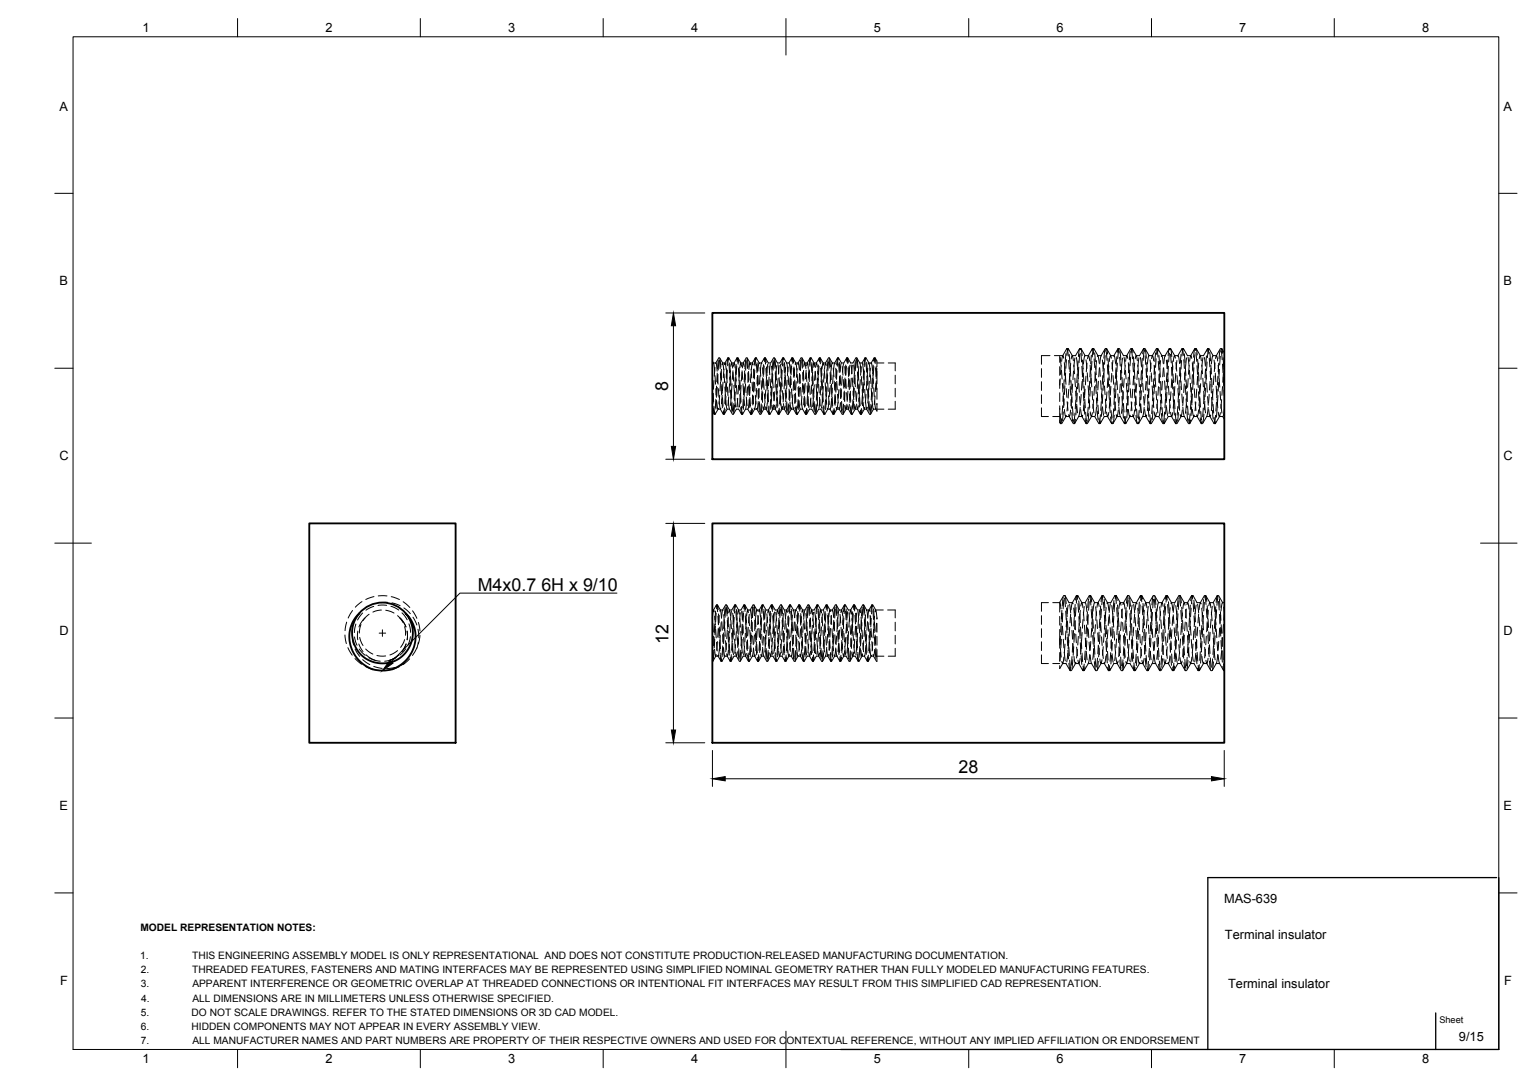
ISO-10303-21;
HEADER;
/* Generated by software containing ST-Developer
 * from STEP Tools, Inc. (www.steptools.com) 
 */

FILE_DESCRIPTION(
/* description */ ('Independent maintained push-to-latch/pull-to-reset mushroom-operator 
CAD. Two opposed spring-loaded ball detents in turned circular seats b
ias both travel stops; direct normally-closed bridge opens6mm when pre
ssed. Rounded palm/pull rim, captured head screw, removable detent clo
sures, native Coil spring families, insulated shared terminals and ord
inary machining features. Manual geometric states and ideal same-mater
ial spring-energy direction only; no electrical/safety certification, 
force/contact dynamics, wear, load or life rating. Requested blue/gray
 visual palette, not safety identification. External wiring/anchors an
d application engineering omitted.'),
/* implementation_level */ '2;1');

FILE_NAME(
/* name */ 'Terminal insulator.step',
/* time_stamp */ '2026-11-08T17:54:26-08:00',
/* author */ (''),
/* organization */ (''),
/* preprocessor_version */ 'ST-DEVELOPER v20.2',
/* originating_system */ 'Autodesk Translation Framework v15.17.0.0',
/* authorisation */ '');

FILE_SCHEMA (('AUTOMOTIVE_DESIGN { 1 0 10303 214 3 1 1 }'));
ENDSEC;

DATA;
#10=MECHANICAL_DESIGN_GEOMETRIC_PRESENTATION_REPRESENTATION('',(#197),#43980);
#163=SHAPE_REPRESENTATION_RELATIONSHIP('SRR','None',#44063,#180);
#180=ADVANCED_BREP_SHAPE_REPRESENTATION('',(#214),#43970);
#197=STYLED_ITEM('',(#44156),#214);
#214=MANIFOLD_SOLID_BREP('Body1',#11238);
#243=B_SPLINE_SURFACE_WITH_KNOTS('',3,3,((#32192,#32193,#32194,#32195,#32196,
#32197,#32198,#32199,#32200,#32201,#32202,#32203,#32204,#32205,#32206,#32207,
#32208,#32209,#32210,#32211,#32212,#32213,#32214,#32215,#32216,#32217,#32218,
#32219,#32220,#32221,#32222,#32223,#32224,#32225,#32226,#32227,#32228,#32229,
#32230,#32231,#32232,#32233,#32234,#32235,#32236,#32237,#32238,#32239,#32240,
#32241,#32242,#32243,#32244,#32245,#32246,#32247,#32248,#32249,#32250,#32251,
#32252,#32253,#32254,#32255,#32256,#32257,#32258,#32259,#32260,#32261,#32262,
#32263,#32264,#32265,#32266,#32267,#32268,#32269,#32270,#32271,#32272,#32273,
#32274,#32275,#32276,#32277,#32278,#32279,#32280,#32281,#32282,#32283,#32284,
#32285,#32286,#32287,#32288,#32289,#32290,#32291,#32292,#32293,#32294,#32295,
#32296,#32297,#32298,#32299,#32300,#32301,#32302,#32303,#32304,#32305,#32306,
#32307,#32308,#32309,#32310),(#32311,#32312,#32313,#32314,#32315,#32316,
#32317,#32318,#32319,#32320,#32321,#32322,#32323,#32324,#32325,#32326,#32327,
#32328,#32329,#32330,#32331,#32332,#32333,#32334,#32335,#32336,#32337,#32338,
#32339,#32340,#32341,#32342,#32343,#32344,#32345,#32346,#32347,#32348,#32349,
#32350,#32351,#32352,#32353,#32354,#32355,#32356,#32357,#32358,#32359,#32360,
#32361,#32362,#32363,#32364,#32365,#32366,#32367,#32368,#32369,#32370,#32371,
#32372,#32373,#32374,#32375,#32376,#32377,#32378,#32379,#32380,#32381,#32382,
#32383,#32384,#32385,#32386,#32387,#32388,#32389,#32390,#32391,#32392,#32393,
#32394,#32395,#32396,#32397,#32398,#32399,#32400,#32401,#32402,#32403,#32404,
#32405,#32406,#32407,#32408,#32409,#32410,#32411,#32412,#32413,#32414,#32415,
#32416,#32417,#32418,#32419,#32420,#32421,#32422,#32423,#32424,#32425,#32426,
#32427,#32428,#32429),(#32430,#32431,#32432,#32433,#32434,#32435,#32436,
#32437,#32438,#32439,#32440,#32441,#32442,#32443,#32444,#32445,#32446,#32447,
#32448,#32449,#32450,#32451,#32452,#32453,#32454,#32455,#32456,#32457,#32458,
#32459,#32460,#32461,#32462,#32463,#32464,#32465,#32466,#32467,#32468,#32469,
#32470,#32471,#32472,#32473,#32474,#32475,#32476,#32477,#32478,#32479,#32480,
#32481,#32482,#32483,#32484,#32485,#32486,#32487,#32488,#32489,#32490,#32491,
#32492,#32493,#32494,#32495,#32496,#32497,#32498,#32499,#32500,#32501,#32502,
#32503,#32504,#32505,#32506,#32507,#32508,#32509,#32510,#32511,#32512,#32513,
#32514,#32515,#32516,#32517,#32518,#32519,#32520,#32521,#32522,#32523,#32524,
#32525,#32526,#32527,#32528,#32529,#32530,#32531,#32532,#32533,#32534,#32535,
#32536,#32537,#32538,#32539,#32540,#32541,#32542,#32543,#32544,#32545,#32546,
#32547,#32548),(#32549,#32550,#32551,#32552,#32553,#32554,#32555,#32556,
#32557,#32558,#32559,#32560,#32561,#32562,#32563,#32564,#32565,#32566,#32567,
#32568,#32569,#32570,#32571,#32572,#32573,#32574,#32575,#32576,#32577,#32578,
#32579,#32580,#32581,#32582,#32583,#32584,#32585,#32586,#32587,#32588,#32589,
#32590,#32591,#32592,#32593,#32594,#32595,#32596,#32597,#32598,#32599,#32600,
#32601,#32602,#32603,#32604,#32605,#32606,#32607,#32608,#32609,#32610,#32611,
#32612,#32613,#32614,#32615,#32616,#32617,#32618,#32619,#32620,#32621,#32622,
#32623,#32624,#32625,#32626,#32627,#32628,#32629,#32630,#32631,#32632,#32633,
#32634,#32635,#32636,#32637,#32638,#32639,#32640,#32641,#32642,#32643,#32644,
#32645,#32646,#32647,#32648,#32649,#32650,#32651,#32652,#32653,#32654,#32655,
#32656,#32657,#32658,#32659,#32660,#32661,#32662,#32663,#32664,#32665,#32666,
#32667)),.UNSPECIFIED.,.F.,.F.,.F.,(4,4),(4,1,1,1,1,1,1,1,1,1,1,1,1,1,1,
1,1,1,1,1,1,1,1,1,1,1,1,1,1,1,1,1,1,1,1,1,1,1,1,1,1,1,1,1,1,1,1,1,1,1,1,
1,1,1,1,1,1,1,1,1,1,1,1,1,1,1,1,1,1,1,1,1,1,1,1,1,1,1,1,1,1,1,1,1,1,1,1,
1,1,1,1,1,1,1,1,1,1,1,1,1,1,1,1,1,1,1,1,1,1,1,1,1,1,1,1,1,4),(0.,0.0321584099938621),
(11.8553612635792,12.8477570223809,13.8401527811825,14.8325485399841,15.8249442987858,
16.8173400575874,17.809735816389,18.8021315751907,19.7945273339923,20.7869230927939,
21.7793188515956,22.7717146103972,23.7641103691988,24.7565061280005,25.7489018868021,
26.7412976456037,27.7336934044054,28.726089163207,29.7184849220086,30.7108806808103,
31.7032764396119,32.6956721984135,33.6880679572152,34.6804637160168,35.6728594748184,
36.6652552336201,37.6576509924217,38.6500467512233,39.642442510025,40.6348382688266,
41.6272340276282,42.6196297864299,43.6120255452315,44.6044213040331,45.5968170628348,
46.5892128216364,47.581608580438,48.5740043392397,49.5664000980413,50.5587958568429,
51.5511916156446,52.5435873744462,53.5359831332478,54.5283788920495,55.5207746508511,
56.5131704096527,57.5055661684544,58.497961927256,59.4903576860576,60.4827534448593,
61.4751492036609,62.4675449624625,63.4599407212642,64.4523364800658,65.4447322388674,
66.4371279976691,67.4295237564707,68.4219195152723,69.4143152740739,70.4067110328756,
71.3991067916772,72.3915025504788,73.3838983092805,74.3762940680821,75.3686898268838,
76.3610855856854,77.353481344487,78.3458771032886,79.3382728620903,80.3306686208919,
81.3230643796935,82.3154601384952,83.3078558972968,84.3002516560985,85.2926474149001,
86.2850431737017,87.2774389325033,88.269834691305,89.2622304501066,90.2546262089082,
91.2470219677099,92.2394177265115,93.2318134853131,94.2242092441148,95.2166050029164,
96.209000761718,97.2013965205197,98.1937922793213,99.1861880381229,100.178583796925,
101.170979555726,102.163375314528,103.155771073329,104.148166832131,105.140562590933,
106.132958349734,107.125354108536,108.117749867338,109.110145626139,110.102541384941,
111.094937143743,112.087332902544,113.079728661346,114.072124420147,115.064520178949,
116.056915937751,117.049311696552,118.041707455354,119.034103214156,120.026498972957,
121.018894731759,122.01129049056,123.003686249362,123.996082008164,124.988477766965,
125.980873525767,126.973269284569),.UNSPECIFIED.);
#244=B_SPLINE_SURFACE_WITH_KNOTS('',3,3,((#32742,#32743,#32744,#32745,#32746,
#32747,#32748,#32749,#32750,#32751,#32752,#32753,#32754,#32755,#32756,#32757,
#32758,#32759,#32760,#32761,#32762,#32763,#32764,#32765,#32766,#32767,#32768,
#32769,#32770,#32771,#32772,#32773,#32774,#32775,#32776,#32777,#32778,#32779,
#32780,#32781,#32782,#32783,#32784,#32785,#32786,#32787,#32788,#32789,#32790,
#32791,#32792,#32793,#32794,#32795,#32796,#32797,#32798,#32799,#32800,#32801,
#32802,#32803,#32804,#32805,#32806,#32807,#32808,#32809,#32810,#32811,#32812,
#32813,#32814,#32815,#32816,#32817,#32818,#32819,#32820,#32821,#32822,#32823,
#32824,#32825,#32826,#32827,#32828,#32829,#32830,#32831,#32832,#32833,#32834,
#32835,#32836,#32837,#32838,#32839,#32840,#32841,#32842,#32843,#32844,#32845,
#32846,#32847,#32848,#32849,#32850,#32851,#32852,#32853,#32854,#32855,#32856,
#32857,#32858,#32859,#32860),(#32861,#32862,#32863,#32864,#32865,#32866,
#32867,#32868,#32869,#32870,#32871,#32872,#32873,#32874,#32875,#32876,#32877,
#32878,#32879,#32880,#32881,#32882,#32883,#32884,#32885,#32886,#32887,#32888,
#32889,#32890,#32891,#32892,#32893,#32894,#32895,#32896,#32897,#32898,#32899,
#32900,#32901,#32902,#32903,#32904,#32905,#32906,#32907,#32908,#32909,#32910,
#32911,#32912,#32913,#32914,#32915,#32916,#32917,#32918,#32919,#32920,#32921,
#32922,#32923,#32924,#32925,#32926,#32927,#32928,#32929,#32930,#32931,#32932,
#32933,#32934,#32935,#32936,#32937,#32938,#32939,#32940,#32941,#32942,#32943,
#32944,#32945,#32946,#32947,#32948,#32949,#32950,#32951,#32952,#32953,#32954,
#32955,#32956,#32957,#32958,#32959,#32960,#32961,#32962,#32963,#32964,#32965,
#32966,#32967,#32968,#32969,#32970,#32971,#32972,#32973,#32974,#32975,#32976,
#32977,#32978,#32979),(#32980,#32981,#32982,#32983,#32984,#32985,#32986,
#32987,#32988,#32989,#32990,#32991,#32992,#32993,#32994,#32995,#32996,#32997,
#32998,#32999,#33000,#33001,#33002,#33003,#33004,#33005,#33006,#33007,#33008,
#33009,#33010,#33011,#33012,#33013,#33014,#33015,#33016,#33017,#33018,#33019,
#33020,#33021,#33022,#33023,#33024,#33025,#33026,#33027,#33028,#33029,#33030,
#33031,#33032,#33033,#33034,#33035,#33036,#33037,#33038,#33039,#33040,#33041,
#33042,#33043,#33044,#33045,#33046,#33047,#33048,#33049,#33050,#33051,#33052,
#33053,#33054,#33055,#33056,#33057,#33058,#33059,#33060,#33061,#33062,#33063,
#33064,#33065,#33066,#33067,#33068,#33069,#33070,#33071,#33072,#33073,#33074,
#33075,#33076,#33077,#33078,#33079,#33080,#33081,#33082,#33083,#33084,#33085,
#33086,#33087,#33088,#33089,#33090,#33091,#33092,#33093,#33094,#33095,#33096,
#33097,#33098),(#33099,#33100,#33101,#33102,#33103,#33104,#33105,#33106,
#33107,#33108,#33109,#33110,#33111,#33112,#33113,#33114,#33115,#33116,#33117,
#33118,#33119,#33120,#33121,#33122,#33123,#33124,#33125,#33126,#33127,#33128,
#33129,#33130,#33131,#33132,#33133,#33134,#33135,#33136,#33137,#33138,#33139,
#33140,#33141,#33142,#33143,#33144,#33145,#33146,#33147,#33148,#33149,#33150,
#33151,#33152,#33153,#33154,#33155,#33156,#33157,#33158,#33159,#33160,#33161,
#33162,#33163,#33164,#33165,#33166,#33167,#33168,#33169,#33170,#33171,#33172,
#33173,#33174,#33175,#33176,#33177,#33178,#33179,#33180,#33181,#33182,#33183,
#33184,#33185,#33186,#33187,#33188,#33189,#33190,#33191,#33192,#33193,#33194,
#33195,#33196,#33197,#33198,#33199,#33200,#33201,#33202,#33203,#33204,#33205,
#33206,#33207,#33208,#33209,#33210,#33211,#33212,#33213,#33214,#33215,#33216,
#33217)),.UNSPECIFIED.,.F.,.F.,.F.,(4,4),(4,1,1,1,1,1,1,1,1,1,1,1,1,1,1,
1,1,1,1,1,1,1,1,1,1,1,1,1,1,1,1,1,1,1,1,1,1,1,1,1,1,1,1,1,1,1,1,1,1,1,1,
1,1,1,1,1,1,1,1,1,1,1,1,1,1,1,1,1,1,1,1,1,1,1,1,1,1,1,1,1,1,1,1,1,1,1,1,
1,1,1,1,1,1,1,1,1,1,1,1,1,1,1,1,1,1,1,1,1,1,1,1,1,1,1,1,1,4),(0.,0.0321584099938621),
(14.3984001269718,15.3907958857734,16.383191644575,17.3755874033767,18.3679831621783,
19.3603789209799,20.3527746797816,21.3451704385832,22.3375661973848,23.3299619561865,
24.3223577149881,25.3147534737897,26.3071492325914,27.299544991393,28.2919407501946,
29.2843365089963,30.2767322677979,31.2691280265995,32.2615237854012,33.2539195442028,
34.2463153030044,35.2387110618061,36.2311068206077,37.2235025794093,38.215898338211,
39.2082940970126,40.2006898558142,41.1930856146159,42.1854813734175,43.1778771322191,
44.1702728910208,45.1626686498224,46.155064408624,47.1474601674257,48.1398559262273,
49.1322516850289,50.1246474438306,51.1170432026322,52.1094389614338,53.1018347202355,
54.0942304790371,55.0866262378387,56.0790219966403,57.071417755442,58.0638135142436,
59.0562092730452,60.0486050318469,61.0410007906485,62.0333965494501,63.0257923082518,
64.0181880670534,65.010583825855,66.0029795846567,66.9953753434583,67.9877711022599,
68.9801668610616,69.9725626198632,70.9649583786648,71.9573541374665,72.9497498962681,
73.9421456550697,74.9345414138714,75.926937172673,76.9193329314746,77.9117286902763,
78.9041244490779,79.8965202078795,80.8889159666812,81.8813117254828,82.8737074842844,
83.8661032430861,84.8584990018877,85.8508947606893,86.8432905194909,87.8356862782926,
88.8280820370942,89.8204777958959,90.8128735546975,91.8052693134991,92.7976650723007,
93.7900608311024,94.782456589904,95.7748523487057,96.7672481075073,97.7596438663089,
98.7520396251105,99.7444353839122,100.736831142714,101.729226901515,102.721622660317,
103.714018419119,104.70641417792,105.698809936722,106.691205695524,107.683601454325,
108.675997213127,109.668392971929,110.66078873073,111.653184489532,112.645580248333,
113.637976007135,114.630371765937,115.622767524738,116.61516328354,117.607559042342,
118.599954801143,119.592350559945,120.584746318746,121.577142077548,122.56953783635,
123.561933595151,124.554329353953,125.546725112755,126.539120871556,127.531516630358,
128.52391238916,129.516308147961),.UNSPECIFIED.);
#245=B_SPLINE_SURFACE_WITH_KNOTS('',3,3,((#33424,#33425,#33426,#33427,#33428,
#33429,#33430,#33431,#33432,#33433,#33434,#33435,#33436,#33437,#33438,#33439,
#33440,#33441,#33442,#33443,#33444,#33445,#33446,#33447,#33448,#33449,#33450,
#33451,#33452,#33453,#33454,#33455,#33456,#33457,#33458,#33459,#33460,#33461,
#33462,#33463,#33464,#33465,#33466,#33467,#33468,#33469,#33470,#33471,#33472,
#33473,#33474,#33475,#33476,#33477,#33478,#33479,#33480,#33481,#33482,#33483,
#33484,#33485,#33486,#33487,#33488,#33489,#33490,#33491,#33492,#33493,#33494,
#33495,#33496,#33497,#33498,#33499,#33500,#33501,#33502,#33503,#33504,#33505,
#33506,#33507,#33508,#33509),(#33510,#33511,#33512,#33513,#33514,#33515,
#33516,#33517,#33518,#33519,#33520,#33521,#33522,#33523,#33524,#33525,#33526,
#33527,#33528,#33529,#33530,#33531,#33532,#33533,#33534,#33535,#33536,#33537,
#33538,#33539,#33540,#33541,#33542,#33543,#33544,#33545,#33546,#33547,#33548,
#33549,#33550,#33551,#33552,#33553,#33554,#33555,#33556,#33557,#33558,#33559,
#33560,#33561,#33562,#33563,#33564,#33565,#33566,#33567,#33568,#33569,#33570,
#33571,#33572,#33573,#33574,#33575,#33576,#33577,#33578,#33579,#33580,#33581,
#33582,#33583,#33584,#33585,#33586,#33587,#33588,#33589,#33590,#33591,#33592,
#33593,#33594,#33595),(#33596,#33597,#33598,#33599,#33600,#33601,#33602,
#33603,#33604,#33605,#33606,#33607,#33608,#33609,#33610,#33611,#33612,#33613,
#33614,#33615,#33616,#33617,#33618,#33619,#33620,#33621,#33622,#33623,#33624,
#33625,#33626,#33627,#33628,#33629,#33630,#33631,#33632,#33633,#33634,#33635,
#33636,#33637,#33638,#33639,#33640,#33641,#33642,#33643,#33644,#33645,#33646,
#33647,#33648,#33649,#33650,#33651,#33652,#33653,#33654,#33655,#33656,#33657,
#33658,#33659,#33660,#33661,#33662,#33663,#33664,#33665,#33666,#33667,#33668,
#33669,#33670,#33671,#33672,#33673,#33674,#33675,#33676,#33677,#33678,#33679,
#33680,#33681),(#33682,#33683,#33684,#33685,#33686,#33687,#33688,#33689,
#33690,#33691,#33692,#33693,#33694,#33695,#33696,#33697,#33698,#33699,#33700,
#33701,#33702,#33703,#33704,#33705,#33706,#33707,#33708,#33709,#33710,#33711,
#33712,#33713,#33714,#33715,#33716,#33717,#33718,#33719,#33720,#33721,#33722,
#33723,#33724,#33725,#33726,#33727,#33728,#33729,#33730,#33731,#33732,#33733,
#33734,#33735,#33736,#33737,#33738,#33739,#33740,#33741,#33742,#33743,#33744,
#33745,#33746,#33747,#33748,#33749,#33750,#33751,#33752,#33753,#33754,#33755,
#33756,#33757,#33758,#33759,#33760,#33761,#33762,#33763,#33764,#33765,#33766,
#33767)),.UNSPECIFIED.,.F.,.F.,.F.,(4,4),(4,1,1,1,1,1,1,1,1,1,1,1,1,1,1,
1,1,1,1,1,1,1,1,1,1,1,1,1,1,1,1,1,1,1,1,1,1,1,1,1,1,1,1,1,1,1,1,1,1,1,1,
1,1,1,1,1,1,1,1,1,1,1,1,1,1,1,1,1,1,1,1,1,1,1,1,1,1,1,1,1,1,1,1,4),(0.,
0.0448889834294934),(11.8615800042567,12.8591513772396,13.8567227502225,
14.8542941232054,15.8518654961884,16.8494368691713,17.8470082421542,18.8445796151372,
19.8421509881201,20.839722361103,21.837293734086,22.8348651070689,23.8324364800518,
24.8300078530348,25.8275792260177,26.8251505990006,27.8227219719836,28.8202933449665,
29.8178647179494,30.8154360909324,31.8130074639153,32.8105788368982,33.8081502098812,
34.8057215828641,35.803292955847,36.80086432883,37.7984357018129,38.7960070747958,
39.7935784477788,40.7911498207617,41.7887211937446,42.7862925667276,43.7838639397105,
44.7814353126934,45.7790066856764,46.7765780586593,47.7741494316422,48.7717208046252,
49.7692921776081,50.766863550591,51.764434923574,52.7620062965569,53.7595776695398,
54.7571490425228,55.7547204155057,56.7522917884886,57.7498631614716,58.7474345344545,
59.7450059074374,60.7425772804204,61.7401486534033,62.7377200263862,63.7352913993692,
64.7328627723521,65.730434145335,66.728005518318,67.7255768913009,68.7231482642838,
69.7207196372668,70.7182910102497,71.7158623832326,72.7134337562156,73.7110051291985,
74.7085765021814,75.7061478751643,76.7037192481473,77.7012906211302,78.6988619941132,
79.6964333670961,80.694004740079,81.691576113062,82.6891474860449,83.6867188590278,
84.6842902320108,85.6818616049937,86.6794329779766,87.6770043509595,88.6745757239425,
89.6721470969254,90.6697184699083,91.6672898428913,92.6648612158742,93.6624325888571,
94.6600039618401),.UNSPECIFIED.);
#246=B_SPLINE_SURFACE_WITH_KNOTS('',3,3,((#33845,#33846,#33847,#33848,#33849,
#33850,#33851,#33852,#33853,#33854,#33855,#33856,#33857,#33858,#33859,#33860,
#33861,#33862,#33863,#33864,#33865,#33866,#33867,#33868,#33869,#33870,#33871,
#33872,#33873,#33874,#33875,#33876,#33877,#33878,#33879,#33880,#33881,#33882,
#33883,#33884,#33885,#33886,#33887,#33888,#33889,#33890,#33891,#33892,#33893,
#33894,#33895,#33896,#33897,#33898,#33899,#33900,#33901,#33902,#33903,#33904,
#33905,#33906,#33907,#33908,#33909,#33910,#33911,#33912,#33913,#33914,#33915,
#33916,#33917,#33918,#33919,#33920,#33921,#33922,#33923,#33924,#33925,#33926,
#33927,#33928,#33929,#33930),(#33931,#33932,#33933,#33934,#33935,#33936,
#33937,#33938,#33939,#33940,#33941,#33942,#33943,#33944,#33945,#33946,#33947,
#33948,#33949,#33950,#33951,#33952,#33953,#33954,#33955,#33956,#33957,#33958,
#33959,#33960,#33961,#33962,#33963,#33964,#33965,#33966,#33967,#33968,#33969,
#33970,#33971,#33972,#33973,#33974,#33975,#33976,#33977,#33978,#33979,#33980,
#33981,#33982,#33983,#33984,#33985,#33986,#33987,#33988,#33989,#33990,#33991,
#33992,#33993,#33994,#33995,#33996,#33997,#33998,#33999,#34000,#34001,#34002,
#34003,#34004,#34005,#34006,#34007,#34008,#34009,#34010,#34011,#34012,#34013,
#34014,#34015,#34016),(#34017,#34018,#34019,#34020,#34021,#34022,#34023,
#34024,#34025,#34026,#34027,#34028,#34029,#34030,#34031,#34032,#34033,#34034,
#34035,#34036,#34037,#34038,#34039,#34040,#34041,#34042,#34043,#34044,#34045,
#34046,#34047,#34048,#34049,#34050,#34051,#34052,#34053,#34054,#34055,#34056,
#34057,#34058,#34059,#34060,#34061,#34062,#34063,#34064,#34065,#34066,#34067,
#34068,#34069,#34070,#34071,#34072,#34073,#34074,#34075,#34076,#34077,#34078,
#34079,#34080,#34081,#34082,#34083,#34084,#34085,#34086,#34087,#34088,#34089,
#34090,#34091,#34092,#34093,#34094,#34095,#34096,#34097,#34098,#34099,#34100,
#34101,#34102),(#34103,#34104,#34105,#34106,#34107,#34108,#34109,#34110,
#34111,#34112,#34113,#34114,#34115,#34116,#34117,#34118,#34119,#34120,#34121,
#34122,#34123,#34124,#34125,#34126,#34127,#34128,#34129,#34130,#34131,#34132,
#34133,#34134,#34135,#34136,#34137,#34138,#34139,#34140,#34141,#34142,#34143,
#34144,#34145,#34146,#34147,#34148,#34149,#34150,#34151,#34152,#34153,#34154,
#34155,#34156,#34157,#34158,#34159,#34160,#34161,#34162,#34163,#34164,#34165,
#34166,#34167,#34168,#34169,#34170,#34171,#34172,#34173,#34174,#34175,#34176,
#34177,#34178,#34179,#34180,#34181,#34182,#34183,#34184,#34185,#34186,#34187,
#34188)),.UNSPECIFIED.,.F.,.F.,.F.,(4,4),(4,1,1,1,1,1,1,1,1,1,1,1,1,1,1,
1,1,1,1,1,1,1,1,1,1,1,1,1,1,1,1,1,1,1,1,1,1,1,1,1,1,1,1,1,1,1,1,1,1,1,1,
1,1,1,1,1,1,1,1,1,1,1,1,1,1,1,1,1,1,1,1,1,1,1,1,1,1,1,1,1,1,1,1,4),(0.,
0.0448889834294934),(14.3981410127769,15.3957123857598,16.3932837587428,
17.3908551317257,18.3884265047086,19.3859978776916,20.3835692506745,21.3811406236574,
22.3787119966404,23.3762833696233,24.3738547426062,25.3714261155892,26.3689974885721,
27.366568861555,28.364140234538,29.3617116075209,30.3592829805038,31.3568543534868,
32.3544257264697,33.3519970994526,34.3495684724355,35.3471398454185,36.3447112184014,
37.3422825913843,38.3398539643673,39.3374253373502,40.3349967103331,41.3325680833161,
42.330139456299,43.3277108292819,44.3252822022649,45.3228535752478,46.3204249482307,
47.3179963212137,48.3155676941966,49.3131390671795,50.3107104401625,51.3082818131454,
52.3058531861283,53.3034245591113,54.3009959320942,55.2985673050771,56.2961386780601,
57.293710051043,58.2912814240259,59.2888527970089,60.2864241699918,61.2839955429747,
62.2815669159577,63.2791382889406,64.2767096619235,65.2742810349065,66.2718524078894,
67.2694237808723,68.2669951538553,69.2645665268382,70.2621378998211,71.2597092728041,
72.257280645787,73.2548520187699,74.2524233917529,75.2499947647358,76.2475661377187,
77.2451375107017,78.2427088836846,79.2402802566675,80.2378516296505,81.2354230026334,
82.2329943756163,83.2305657485993,84.2281371215822,85.2257084945651,86.2232798675481,
87.220851240531,88.2184226135139,89.2159939864969,90.2135653594798,91.2111367324627,
92.2087081054457,93.2062794784286,94.2038508514115,95.2014222243944,96.1989935973774,
97.1965649703603),.UNSPECIFIED.);
#315=FACE_BOUND('',#1577,.T.);
#316=FACE_BOUND('',#1579,.T.);
#413=PLANE('',#11969);
#414=PLANE('',#11972);
#415=PLANE('',#11973);
#416=PLANE('',#11976);
#417=PLANE('',#11977);
#418=PLANE('',#11978);
#419=PLANE('',#11979);
#420=PLANE('',#11980);
#421=PLANE('',#11981);
#422=PLANE('',#11982);
#820=FACE_OUTER_BOUND('',#1499,.T.);
#821=FACE_OUTER_BOUND('',#1500,.T.);
#822=FACE_OUTER_BOUND('',#1501,.T.);
#823=FACE_OUTER_BOUND('',#1502,.T.);
#824=FACE_OUTER_BOUND('',#1503,.T.);
#825=FACE_OUTER_BOUND('',#1504,.T.);
#826=FACE_OUTER_BOUND('',#1505,.T.);
#827=FACE_OUTER_BOUND('',#1506,.T.);
#828=FACE_OUTER_BOUND('',#1507,.T.);
#829=FACE_OUTER_BOUND('',#1508,.T.);
#830=FACE_OUTER_BOUND('',#1509,.T.);
#831=FACE_OUTER_BOUND('',#1510,.T.);
#832=FACE_OUTER_BOUND('',#1511,.T.);
#833=FACE_OUTER_BOUND('',#1512,.T.);
#834=FACE_OUTER_BOUND('',#1513,.T.);
#835=FACE_OUTER_BOUND('',#1514,.T.);
#836=FACE_OUTER_BOUND('',#1515,.T.);
#837=FACE_OUTER_BOUND('',#1516,.T.);
#838=FACE_OUTER_BOUND('',#1517,.T.);
#839=FACE_OUTER_BOUND('',#1518,.T.);
#840=FACE_OUTER_BOUND('',#1519,.T.);
#841=FACE_OUTER_BOUND('',#1520,.T.);
#842=FACE_OUTER_BOUND('',#1521,.T.);
#843=FACE_OUTER_BOUND('',#1522,.T.);
#844=FACE_OUTER_BOUND('',#1523,.T.);
#845=FACE_OUTER_BOUND('',#1524,.T.);
#846=FACE_OUTER_BOUND('',#1525,.T.);
#847=FACE_OUTER_BOUND('',#1526,.T.);
#848=FACE_OUTER_BOUND('',#1527,.T.);
#849=FACE_OUTER_BOUND('',#1528,.T.);
#850=FACE_OUTER_BOUND('',#1529,.T.);
#851=FACE_OUTER_BOUND('',#1530,.T.);
#852=FACE_OUTER_BOUND('',#1531,.T.);
#853=FACE_OUTER_BOUND('',#1532,.T.);
#854=FACE_OUTER_BOUND('',#1533,.T.);
#855=FACE_OUTER_BOUND('',#1534,.T.);
#856=FACE_OUTER_BOUND('',#1535,.T.);
#857=FACE_OUTER_BOUND('',#1536,.T.);
#858=FACE_OUTER_BOUND('',#1537,.T.);
#859=FACE_OUTER_BOUND('',#1538,.T.);
#860=FACE_OUTER_BOUND('',#1539,.T.);
#861=FACE_OUTER_BOUND('',#1540,.T.);
#862=FACE_OUTER_BOUND('',#1541,.T.);
#863=FACE_OUTER_BOUND('',#1542,.T.);
#864=FACE_OUTER_BOUND('',#1543,.T.);
#865=FACE_OUTER_BOUND('',#1544,.T.);
#866=FACE_OUTER_BOUND('',#1545,.T.);
#867=FACE_OUTER_BOUND('',#1546,.T.);
#868=FACE_OUTER_BOUND('',#1547,.T.);
#869=FACE_OUTER_BOUND('',#1548,.T.);
#870=FACE_OUTER_BOUND('',#1549,.T.);
#871=FACE_OUTER_BOUND('',#1550,.T.);
#872=FACE_OUTER_BOUND('',#1551,.T.);
#873=FACE_OUTER_BOUND('',#1552,.T.);
#874=FACE_OUTER_BOUND('',#1553,.T.);
#875=FACE_OUTER_BOUND('',#1554,.T.);
#876=FACE_OUTER_BOUND('',#1555,.T.);
#877=FACE_OUTER_BOUND('',#1556,.T.);
#878=FACE_OUTER_BOUND('',#1557,.T.);
#879=FACE_OUTER_BOUND('',#1558,.T.);
#880=FACE_OUTER_BOUND('',#1559,.T.);
#881=FACE_OUTER_BOUND('',#1560,.T.);
#882=FACE_OUTER_BOUND('',#1561,.T.);
#883=FACE_OUTER_BOUND('',#1562,.T.);
#884=FACE_OUTER_BOUND('',#1563,.T.);
#885=FACE_OUTER_BOUND('',#1564,.T.);
#886=FACE_OUTER_BOUND('',#1565,.T.);
#887=FACE_OUTER_BOUND('',#1566,.T.);
#888=FACE_OUTER_BOUND('',#1567,.T.);
#889=FACE_OUTER_BOUND('',#1568,.T.);
#890=FACE_OUTER_BOUND('',#1569,.T.);
#891=FACE_OUTER_BOUND('',#1570,.T.);
#892=FACE_OUTER_BOUND('',#1571,.T.);
#893=FACE_OUTER_BOUND('',#1572,.T.);
#894=FACE_OUTER_BOUND('',#1573,.T.);
#895=FACE_OUTER_BOUND('',#1574,.T.);
#896=FACE_OUTER_BOUND('',#1575,.T.);
#897=FACE_OUTER_BOUND('',#1576,.T.);
#898=FACE_OUTER_BOUND('',#1578,.T.);
#1499=EDGE_LOOP('',(#8651,#8652,#8653,#8654,#8655,#8656,#8657,#8658));
#1500=EDGE_LOOP('',(#8659,#8660,#8661,#8662));
#1501=EDGE_LOOP('',(#8663,#8664,#8665,#8666));
#1502=EDGE_LOOP('',(#8667,#8668,#8669,#8670));
#1503=EDGE_LOOP('',(#8671,#8672,#8673,#8674));
#1504=EDGE_LOOP('',(#8675,#8676,#8677,#8678));
#1505=EDGE_LOOP('',(#8679,#8680,#8681,#8682));
#1506=EDGE_LOOP('',(#8683,#8684,#8685,#8686));
#1507=EDGE_LOOP('',(#8687,#8688,#8689,#8690));
#1508=EDGE_LOOP('',(#8691,#8692,#8693,#8694));
#1509=EDGE_LOOP('',(#8695,#8696,#8697,#8698));
#1510=EDGE_LOOP('',(#8699,#8700,#8701,#8702));
#1511=EDGE_LOOP('',(#8703,#8704,#8705,#8706));
#1512=EDGE_LOOP('',(#8707,#8708,#8709,#8710));
#1513=EDGE_LOOP('',(#8711,#8712,#8713,#8714));
#1514=EDGE_LOOP('',(#8715,#8716,#8717,#8718));
#1515=EDGE_LOOP('',(#8719,#8720,#8721,#8722));
#1516=EDGE_LOOP('',(#8723,#8724,#8725,#8726));
#1517=EDGE_LOOP('',(#8727,#8728,#8729,#8730));
#1518=EDGE_LOOP('',(#8731,#8732,#8733,#8734));
#1519=EDGE_LOOP('',(#8735,#8736,#8737,#8738));
#1520=EDGE_LOOP('',(#8739,#8740,#8741,#8742));
#1521=EDGE_LOOP('',(#8743,#8744,#8745,#8746));
#1522=EDGE_LOOP('',(#8747,#8748,#8749,#8750));
#1523=EDGE_LOOP('',(#8751,#8752,#8753,#8754));
#1524=EDGE_LOOP('',(#8755,#8756,#8757,#8758,#8759,#8760,#8761,#8762));
#1525=EDGE_LOOP('',(#8763,#8764,#8765,#8766));
#1526=EDGE_LOOP('',(#8767,#8768,#8769,#8770));
#1527=EDGE_LOOP('',(#8771,#8772,#8773,#8774));
#1528=EDGE_LOOP('',(#8775,#8776,#8777,#8778));
#1529=EDGE_LOOP('',(#8779,#8780,#8781,#8782));
#1530=EDGE_LOOP('',(#8783,#8784,#8785,#8786));
#1531=EDGE_LOOP('',(#8787,#8788,#8789,#8790));
#1532=EDGE_LOOP('',(#8791,#8792,#8793,#8794));
#1533=EDGE_LOOP('',(#8795,#8796,#8797,#8798));
#1534=EDGE_LOOP('',(#8799,#8800,#8801,#8802));
#1535=EDGE_LOOP('',(#8803,#8804,#8805,#8806));
#1536=EDGE_LOOP('',(#8807,#8808,#8809,#8810));
#1537=EDGE_LOOP('',(#8811,#8812,#8813,#8814));
#1538=EDGE_LOOP('',(#8815,#8816,#8817,#8818));
#1539=EDGE_LOOP('',(#8819,#8820,#8821,#8822));
#1540=EDGE_LOOP('',(#8823,#8824,#8825,#8826));
#1541=EDGE_LOOP('',(#8827,#8828,#8829,#8830));
#1542=EDGE_LOOP('',(#8831,#8832,#8833,#8834));
#1543=EDGE_LOOP('',(#8835,#8836,#8837,#8838));
#1544=EDGE_LOOP('',(#8839,#8840,#8841,#8842));
#1545=EDGE_LOOP('',(#8843,#8844,#8845,#8846));
#1546=EDGE_LOOP('',(#8847,#8848,#8849,#8850));
#1547=EDGE_LOOP('',(#8851,#8852,#8853,#8854));
#1548=EDGE_LOOP('',(#8855,#8856,#8857,#8858));
#1549=EDGE_LOOP('',(#8859,#8860,#8861,#8862));
#1550=EDGE_LOOP('',(#8863,#8864,#8865,#8866));
#1551=EDGE_LOOP('',(#8867,#8868,#8869,#8870));
#1552=EDGE_LOOP('',(#8871,#8872,#8873,#8874));
#1553=EDGE_LOOP('',(#8875,#8876,#8877,#8878));
#1554=EDGE_LOOP('',(#8879,#8880,#8881,#8882));
#1555=EDGE_LOOP('',(#8883,#8884,#8885,#8886));
#1556=EDGE_LOOP('',(#8887,#8888,#8889,#8890));
#1557=EDGE_LOOP('',(#8891,#8892,#8893,#8894));
#1558=EDGE_LOOP('',(#8895,#8896,#8897,#8898));
#1559=EDGE_LOOP('',(#8899,#8900,#8901,#8902));
#1560=EDGE_LOOP('',(#8903,#8904,#8905,#8906,#8907));
#1561=EDGE_LOOP('',(#8908,#8909,#8910,#8911));
#1562=EDGE_LOOP('',(#8912,#8913,#8914,#8915,#8916,#8917,#8918,#8919,#8920,
#8921,#8922,#8923,#8924,#8925,#8926,#8927,#8928,#8929,#8930,#8931,#8932,
#8933,#8934,#8935,#8936,#8937,#8938,#8939,#8940,#8941,#8942,#8943,#8944,
#8945,#8946,#8947,#8948,#8949,#8950,#8951));
#1563=EDGE_LOOP('',(#8952,#8953,#8954,#8955,#8956,#8957,#8958,#8959,#8960,
#8961,#8962,#8963,#8964,#8965,#8966,#8967,#8968,#8969,#8970,#8971,#8972,
#8973,#8974,#8975,#8976,#8977,#8978,#8979,#8980,#8981,#8982,#8983,#8984,
#8985,#8986,#8987,#8988,#8989,#8990,#8991));
#1564=EDGE_LOOP('',(#8992,#8993,#8994,#8995));
#1565=EDGE_LOOP('',(#8996));
#1566=EDGE_LOOP('',(#8997,#8998,#8999,#9000));
#1567=EDGE_LOOP('',(#9001,#9002,#9003,#9004));
#1568=EDGE_LOOP('',(#9005,#9006,#9007,#9008,#9009,#9010,#9011,#9012,#9013,
#9014,#9015,#9016,#9017,#9018,#9019,#9020,#9021,#9022,#9023,#9024,#9025,
#9026,#9027,#9028,#9029,#9030,#9031,#9032,#9033,#9034));
#1569=EDGE_LOOP('',(#9035,#9036,#9037,#9038,#9039,#9040,#9041,#9042,#9043,
#9044,#9045,#9046,#9047,#9048,#9049,#9050,#9051,#9052,#9053,#9054,#9055,
#9056,#9057,#9058,#9059,#9060,#9061,#9062,#9063));
#1570=EDGE_LOOP('',(#9064,#9065,#9066,#9067));
#1571=EDGE_LOOP('',(#9068));
#1572=EDGE_LOOP('',(#9069,#9070,#9071,#9072));
#1573=EDGE_LOOP('',(#9073,#9074,#9075,#9076));
#1574=EDGE_LOOP('',(#9077,#9078,#9079,#9080));
#1575=EDGE_LOOP('',(#9081,#9082,#9083,#9084));
#1576=EDGE_LOOP('',(#9085,#9086,#9087,#9088));
#1577=EDGE_LOOP('',(#9089,#9090,#9091,#9092));
#1578=EDGE_LOOP('',(#9093,#9094,#9095,#9096));
#1579=EDGE_LOOP('',(#9097,#9098,#9099,#9100));
#1936=CIRCLE('',#11898,0.1666);
#1937=CIRCLE('',#11899,0.1666);
#1938=CIRCLE('',#11911,0.1666);
#1939=CIRCLE('',#11913,0.205475);
#1940=CIRCLE('',#11926,0.205475);
#1941=CIRCLE('',#11928,0.12645);
#1942=CIRCLE('',#11929,0.12645);
#1943=CIRCLE('',#11930,0.12645);
#1944=CIRCLE('',#11948,0.12645);
#1945=CIRCLE('',#11950,0.1543);
#1946=CIRCLE('',#11968,0.1543);
#2422=B_SPLINE_CURVE_WITH_KNOTS('',3,(#29861,#29862,#29863,#29864,#29865,
#29866,#29867,#29868,#29869,#29870,#29871,#29872,#29873,#29874,#29875,#29876,
#29877,#29878,#29879,#29880,#29881,#29882),.UNSPECIFIED.,.F.,.F.,(4,3,3,
3,3,3,3,4),(76.7080459413271,76.8129957196858,77.8105670926688,78.8081384656517,
79.8057098386346,80.8032812116176,81.8008525846005,82.7984239575834),
 .UNSPECIFIED.);
#2423=B_SPLINE_CURVE_WITH_KNOTS('',3,(#29886,#29887,#29888,#29889,#29890,
#29891,#29892),.UNSPECIFIED.,.F.,.F.,(4,3,4),(-80.783811092309,-79.8057098386346,
-79.2446069498474),.UNSPECIFIED.);
#2424=B_SPLINE_CURVE_WITH_KNOTS('',3,(#29896,#29897,#29898,#29899,#29900,
#29901,#29902,#29903,#29904,#29905,#29906,#29907,#29908,#29909,#29910,#29911,
#29912,#29913,#29914,#29915,#29916,#29917),.UNSPECIFIED.,.F.,.F.,(4,3,3,
3,3,3,3,4),(-79.2446069498474,-78.8081384656517,-77.8105670926688,-76.8129957196858,
-75.8154243467029,-74.81785297372,-73.820281600737,-72.9614216426678),
 .UNSPECIFIED.);
#2425=B_SPLINE_CURVE_WITH_KNOTS('',3,(#29922,#29923,#29924,#29925,#29926,
#29927,#29928,#29929,#29930,#29931,#29932,#29933,#29934,#29935,#29936,#29937,
#29938,#29939,#29940,#29941,#29942,#29943),.UNSPECIFIED.,.F.,.F.,(4,3,3,
3,3,3,3,4),(70.4248606341475,70.8275674817882,71.8251388547712,72.8227102277541,
73.820281600737,74.81785297372,75.8154243467029,76.7080459413271),
 .UNSPECIFIED.);
#2426=B_SPLINE_CURVE_WITH_KNOTS('',3,(#29944,#29945,#29946,#29947,#29948,
#29949,#29950,#29951,#29952,#29953,#29954,#29955,#29956,#29957,#29958,#29959,
#29960,#29961,#29962,#29963,#29964,#29965,#29966,#29967,#29968),
 .UNSPECIFIED.,.F.,.F.,(4,3,3,3,3,3,3,3,4),(-72.9614216426678,-72.8227102277541,
-71.8251388547712,-70.8275674817882,-69.8299961088053,-68.8324247358224,
-67.8348533628394,-66.8372819898565,-66.6782363354882),.UNSPECIFIED.);
#2427=B_SPLINE_CURVE_WITH_KNOTS('',3,(#29973,#29974,#29975,#29976,#29977,
#29978,#29979,#29980,#29981,#29982,#29983,#29984,#29985,#29986,#29987,#29988,
#29989,#29990,#29991,#29992,#29993,#29994),.UNSPECIFIED.,.F.,.F.,(4,3,3,
3,3,3,3,4),(64.1416753269679,64.8421392438906,65.8397106168736,66.8372819898565,
67.8348533628394,68.8324247358224,69.8299961088053,70.4248606341475),
 .UNSPECIFIED.);
#2428=B_SPLINE_CURVE_WITH_KNOTS('',3,(#29995,#29996,#29997,#29998,#29999,
#30000,#30001,#30002,#30003,#30004,#30005,#30006,#30007,#30008,#30009,#30010,
#30011,#30012,#30013,#30014,#30015,#30016),.UNSPECIFIED.,.F.,.F.,(4,3,3,
3,3,3,3,4),(-66.6782363354882,-65.8397106168736,-64.8421392438907,-63.8445678709077,
-62.8469964979248,-61.8494251249419,-60.8518537519589,-60.3950510283086),
 .UNSPECIFIED.);
#2429=B_SPLINE_CURVE_WITH_KNOTS('',3,(#30021,#30022,#30023,#30024,#30025,
#30026,#30027,#30028,#30029,#30030,#30031,#30032,#30033,#30034,#30035,#30036,
#30037,#30038,#30039,#30040,#30041,#30042),.UNSPECIFIED.,.F.,.F.,(4,3,3,
3,3,3,3,4),(57.8584900197883,58.856711005993,59.854282378976,60.8518537519589,
61.8494251249418,62.8469964979247,63.8445678709077,64.1416753269679),
 .UNSPECIFIED.);
#2430=B_SPLINE_CURVE_WITH_KNOTS('',3,(#30043,#30044,#30045,#30046,#30047,
#30048,#30049,#30050,#30051,#30052,#30053,#30054,#30055,#30056,#30057,#30058,
#30059,#30060,#30061,#30062,#30063,#30064),.UNSPECIFIED.,.F.,.F.,(4,3,3,
3,3,3,3,4),(-60.3950510283086,-59.854282378976,-58.856711005993,-57.8591396330101,
-56.8615682600272,-55.8639968870442,-54.8664255140613,-54.111865721129),
 .UNSPECIFIED.);
#2431=B_SPLINE_CURVE_WITH_KNOTS('',3,(#30069,#30070,#30071,#30072,#30073,
#30074,#30075,#30076,#30077,#30078,#30079,#30080,#30081,#30082,#30083,#30084,
#30085,#30086,#30087,#30088,#30089,#30090),.UNSPECIFIED.,.F.,.F.,(4,3,3,
3,3,3,3,4),(51.5753047126087,51.8737113951125,52.8712827680954,53.8688541410784,
54.8664255140613,55.8639968870442,56.8615682600272,57.8584900197883),
 .UNSPECIFIED.);
#2432=B_SPLINE_CURVE_WITH_KNOTS('',3,(#30091,#30092,#30093,#30094,#30095,
#30096,#30097,#30098,#30099,#30100,#30101,#30102,#30103,#30104,#30105,#30106,
#30107,#30108,#30109,#30110,#30111,#30112,#30113,#30114,#30115),
 .UNSPECIFIED.,.F.,.F.,(4,3,3,3,3,3,3,3,4),(-54.111865721129,-53.8688541410784,
-52.8712827680954,-51.8737113951125,-50.8761400221296,-49.8785686491466,
-48.8809972761637,-47.8834259031808,-47.8286804139494),.UNSPECIFIED.);
#2433=B_SPLINE_CURVE_WITH_KNOTS('',3,(#30120,#30121,#30122,#30123,#30124,
#30125,#30126,#30127,#30128,#30129,#30130,#30131,#30132,#30133,#30134,#30135,
#30136,#30137,#30138,#30139,#30140,#30141),.UNSPECIFIED.,.F.,.F.,(4,3,3,
3,3,3,3,4),(45.2921194054291,45.8882831572149,46.8858545301978,47.8834259031808,
48.8809972761637,49.8785686491466,50.8761400221296,51.5753047126087),
 .UNSPECIFIED.);
#2434=B_SPLINE_CURVE_WITH_KNOTS('',3,(#30142,#30143,#30144,#30145,#30146,
#30147,#30148,#30149,#30150,#30151,#30152,#30153,#30154,#30155,#30156,#30157,
#30158,#30159,#30160,#30161,#30162,#30163),.UNSPECIFIED.,.F.,.F.,(4,3,3,
3,3,3,3,4),(-47.8286804139494,-46.8858545301979,-45.8882831572149,-44.890711784232,
-43.893140411249,-42.8955690382661,-41.8979976652832,-41.5454951067698),
 .UNSPECIFIED.);
#2435=B_SPLINE_CURVE_WITH_KNOTS('',3,(#30168,#30169,#30170,#30171,#30172,
#30173,#30174,#30175,#30176,#30177,#30178,#30179,#30180,#30181,#30182,#30183,
#30184,#30185,#30186,#30187,#30188,#30189),.UNSPECIFIED.,.F.,.F.,(4,3,3,
3,3,3,3,4),(39.0089340982495,39.9028549193173,40.9004262923002,41.8979976652832,
42.8955690382661,43.893140411249,44.890711784232,45.2921194054291),
 .UNSPECIFIED.);
#2436=B_SPLINE_CURVE_WITH_KNOTS('',3,(#30190,#30191,#30192,#30193,#30194,
#30195,#30196,#30197,#30198,#30199,#30200,#30201,#30202,#30203,#30204,#30205,
#30206,#30207,#30208,#30209,#30210,#30211),.UNSPECIFIED.,.F.,.F.,(4,3,3,
3,3,3,3,4),(-41.5454951067698,-40.9004262923003,-39.9028549193173,-38.9052835463344,
-37.9077121733515,-36.9101408003685,-35.9125694273856,-35.2623097995902),
 .UNSPECIFIED.);
#2437=B_SPLINE_CURVE_WITH_KNOTS('',3,(#30216,#30217,#30218,#30219,#30220,
#30221,#30222,#30223,#30224,#30225,#30226,#30227,#30228,#30229,#30230,#30231,
#30232,#30233,#30234,#30235,#30236,#30237,#30238,#30239,#30240),
 .UNSPECIFIED.,.F.,.F.,(4,3,3,3,3,3,3,3,4),(32.7257487910699,32.9198553084368,
33.9174266814197,34.9149980544027,35.9125694273856,36.9101408003685,37.9077121733514,
38.9052835463344,39.0089340982495),.UNSPECIFIED.);
#2438=B_SPLINE_CURVE_WITH_KNOTS('',3,(#30241,#30242,#30243,#30244,#30245,
#30246,#30247,#30248,#30249,#30250,#30251,#30252,#30253,#30254,#30255,#30256,
#30257,#30258,#30259,#30260,#30261,#30262),.UNSPECIFIED.,.F.,.F.,(4,3,3,
3,3,3,3,4),(-35.2623097995902,-34.9149980544027,-33.9174266814197,-32.9198553084368,
-31.9222839354538,-30.9247125624709,-29.927141189488,-28.9791244924106),
 .UNSPECIFIED.);
#2439=B_SPLINE_CURVE_WITH_KNOTS('',3,(#30267,#30268,#30269,#30270,#30271,
#30272,#30273,#30274,#30275,#30276,#30277,#30278,#30279,#30280,#30281,#30282,
#30283,#30284,#30285,#30286,#30287,#30288),.UNSPECIFIED.,.F.,.F.,(4,3,3,
3,3,3,3,4),(26.4425634838903,26.9344270705392,27.9319984435221,28.929569816505,
29.927141189488,30.9247125624709,31.9222839354538,32.7257487910699),
 .UNSPECIFIED.);
#2440=B_SPLINE_CURVE_WITH_KNOTS('',3,(#30289,#30290,#30291,#30292,#30293,
#30294,#30295,#30296,#30297,#30298,#30299,#30300,#30301,#30302,#30303,#30304,
#30305,#30306,#30307,#30308,#30309,#30310,#30311,#30312,#30313),
 .UNSPECIFIED.,.F.,.F.,(4,3,3,3,3,3,3,3,4),(-28.9791244924106,-28.929569816505,
-27.9319984435221,-26.9344270705392,-25.9368556975562,-24.9392843245733,
-23.9417129515904,-22.9441415786075,-22.695939185231),.UNSPECIFIED.);
#2441=B_SPLINE_CURVE_WITH_KNOTS('',3,(#30318,#30319,#30320,#30321,#30322,
#30323,#30324,#30325,#30326,#30327,#30328,#30329,#30330,#30331,#30332,#30333,
#30334,#30335,#30336,#30337,#30338,#30339),.UNSPECIFIED.,.F.,.F.,(4,3,3,
3,3,3,3,4),(20.1593781767107,20.9489988326416,21.9465702056245,22.9441415786074,
23.9417129515904,24.9392843245733,25.9368556975562,26.4425634838903),
 .UNSPECIFIED.);
#2442=B_SPLINE_CURVE_WITH_KNOTS('',3,(#30340,#30341,#30342,#30343,#30344,
#30345,#30346,#30347,#30348,#30349,#30350,#30351,#30352,#30353,#30354,#30355,
#30356,#30357,#30358,#30359,#30360,#30361),.UNSPECIFIED.,.F.,.F.,(4,3,3,
3,3,3,3,4),(-22.695939185231,-21.9465702056245,-20.9489988326416,-19.9514274596586,
-18.9538560866757,-17.9562847136928,-16.9587133407099,-16.4127538780514),
 .UNSPECIFIED.);
#2443=B_SPLINE_CURVE_WITH_KNOTS('',3,(#30366,#30367,#30368,#30369,#30370,
#30371,#30372,#30373,#30374,#30375,#30376,#30377,#30378,#30379,#30380,#30381,
#30382,#30383,#30384,#30385,#30386,#30387,#30388,#30389,#30390),
 .UNSPECIFIED.,.F.,.F.,(4,3,3,3,3,3,3,3,4),(13.8761928695311,13.9659992217611,
14.963570594744,15.9611419677269,16.9587133407099,17.9562847136928,18.9538560866757,
19.9514274596586,20.1593781767107),.UNSPECIFIED.);
#2444=B_SPLINE_CURVE_WITH_KNOTS('',3,(#30391,#30392,#30393,#30394,#30395,
#30396,#30397,#30398,#30399,#30400,#30401,#30402,#30403,#30404,#30405,#30406,
#30407,#30408,#30409,#30410,#30411,#30412),.UNSPECIFIED.,.F.,.F.,(4,3,3,
3,3,3,3,4),(-16.4127538780514,-15.9611419677269,-14.963570594744,-13.9659992217611,
-12.9684278487781,-11.9708564757952,-10.9732851028123,-10.1295685708718),
 .UNSPECIFIED.);
#2445=B_SPLINE_CURVE_WITH_KNOTS('',3,(#30418,#30419,#30420,#30421,#30422,
#30423,#30424,#30425,#30426,#30427,#30428,#30429,#30430),.UNSPECIFIED.,
 .F.,.F.,(4,3,3,3,4),(-3.84638326369226,-2.9927141189488,-1.99514274596587,
-0.997571372982931,0.),.UNSPECIFIED.);
#2446=B_SPLINE_CURVE_WITH_KNOTS('',3,(#30433,#30434,#30435,#30436,#30437,
#30438,#30439,#30440,#30441,#30442,#30443,#30444,#30445,#30446,#30447,#30448,
#30449,#30450,#30451),.UNSPECIFIED.,.F.,.F.,(4,3,3,3,3,3,4),(2.01461286527445,
2.9927141189488,3.99028549193173,4.98785686491467,5.9854282378976,6.98299961088053,
7.59300756235155),.UNSPECIFIED.);
#2447=B_SPLINE_CURVE_WITH_KNOTS('',3,(#30457,#30458,#30459,#30460,#30461,
#30462,#30463),.UNSPECIFIED.,.F.,.F.,(4,1,1,1,4),(91.106186954104,91.6672898428913,
92.6648612158742,93.6624325888571,94.6600039618401),.UNSPECIFIED.);
#2448=B_SPLINE_CURVE_WITH_KNOTS('',3,(#30466,#30467,#30468,#30469,#30470,
#30471,#30472,#30473),.UNSPECIFIED.,.F.,.F.,(4,1,1,1,1,4),(91.106186954104,
91.2111367324627,92.2087081054457,93.2062794784286,94.2038508514115,95.1819521050859),
 .UNSPECIFIED.);
#2449=B_SPLINE_CURVE_WITH_KNOTS('',3,(#30478,#30479,#30480,#30481,#30482,
#30483,#30484,#30485,#30486,#30487),.UNSPECIFIED.,.F.,.F.,(4,1,1,1,1,1,
1,4),(84.8230016469244,85.6818616049937,86.6794329779766,87.6770043509595,
88.6745757239425,89.6721470969254,90.6697184699083,91.106186954104),
 .UNSPECIFIED.);
#2450=B_SPLINE_CURVE_WITH_KNOTS('',3,(#30488,#30489,#30490,#30491,#30492,
#30493,#30494,#30495,#30496,#30497),.UNSPECIFIED.,.F.,.F.,(4,1,1,1,1,1,
1,4),(84.8230016469244,85.2257084945651,86.2232798675481,87.220851240531,
88.2184226135139,89.2159939864969,90.2135653594798,91.106186954104),
 .UNSPECIFIED.);
#2451=B_SPLINE_CURVE_WITH_KNOTS('',3,(#30502,#30503,#30504,#30505,#30506,
#30507,#30508,#30509,#30510,#30511,#30512),.UNSPECIFIED.,.F.,.F.,(4,1,1,
1,1,1,1,1,4),(78.5398163397448,78.6988619941132,79.6964333670961,80.694004740079,
81.691576113062,82.6891474860449,83.6867188590278,84.6842902320108,84.8230016469244),
 .UNSPECIFIED.);
#2452=B_SPLINE_CURVE_WITH_KNOTS('',3,(#30513,#30514,#30515,#30516,#30517,
#30518,#30519,#30520,#30521,#30522),.UNSPECIFIED.,.F.,.F.,(4,1,1,1,1,1,
1,4),(78.5398163397448,79.2402802566675,80.2378516296505,81.2354230026334,
82.2329943756163,83.2305657485993,84.2281371215822,84.8230016469244),
 .UNSPECIFIED.);
#2453=B_SPLINE_CURVE_WITH_KNOTS('',3,(#30527,#30528,#30529,#30530,#30531,
#30532,#30533,#30534,#30535,#30536),.UNSPECIFIED.,.F.,.F.,(4,1,1,1,1,1,
1,4),(72.2566310325652,72.7134337562156,73.7110051291985,74.7085765021814,
75.7061478751643,76.7037192481473,77.7012906211302,78.5398163397448),
 .UNSPECIFIED.);
#2454=B_SPLINE_CURVE_WITH_KNOTS('',3,(#30537,#30538,#30539,#30540,#30541,
#30542,#30543,#30544,#30545,#30546,#30547),.UNSPECIFIED.,.F.,.F.,(4,1,1,
1,1,1,1,1,4),(72.2566310325652,72.257280645787,73.2548520187699,74.2524233917529,
75.2499947647358,76.2475661377187,77.2451375107017,78.2427088836846,78.5398163397448),
 .UNSPECIFIED.);
#2455=B_SPLINE_CURVE_WITH_KNOTS('',3,(#30552,#30553,#30554,#30555,#30556,
#30557,#30558,#30559,#30560,#30561),.UNSPECIFIED.,.F.,.F.,(4,1,1,1,1,1,
1,4),(65.9734457253856,66.728005518318,67.7255768913009,68.7231482642838,
69.7207196372668,70.7182910102497,71.7158623832326,72.2566310325652),
 .UNSPECIFIED.);
#2456=B_SPLINE_CURVE_WITH_KNOTS('',3,(#30562,#30563,#30564,#30565,#30566,
#30567,#30568,#30569,#30570,#30571),.UNSPECIFIED.,.F.,.F.,(4,1,1,1,1,1,
1,4),(65.9734457253856,66.2718524078894,67.2694237808723,68.2669951538553,
69.2645665268382,70.2621378998211,71.2597092728041,72.2566310325652),
 .UNSPECIFIED.);
#2457=B_SPLINE_CURVE_WITH_KNOTS('',3,(#30576,#30577,#30578,#30579,#30580,
#30581,#30582,#30583,#30584,#30585,#30586),.UNSPECIFIED.,.F.,.F.,(4,1,1,
1,1,1,1,1,4),(59.690260418206,59.7450059074374,60.7425772804204,61.7401486534033,
62.7377200263862,63.7352913993692,64.7328627723521,65.730434145335,65.9734457253856),
 .UNSPECIFIED.);
#2458=B_SPLINE_CURVE_WITH_KNOTS('',3,(#30587,#30588,#30589,#30590,#30591,
#30592,#30593,#30594,#30595,#30596),.UNSPECIFIED.,.F.,.F.,(4,1,1,1,1,1,
1,4),(59.690260418206,60.2864241699918,61.2839955429747,62.2815669159577,
63.2791382889406,64.2767096619235,65.2742810349065,65.9734457253856),
 .UNSPECIFIED.);
#2459=B_SPLINE_CURVE_WITH_KNOTS('',3,(#30601,#30602,#30603,#30604,#30605,
#30606,#30607,#30608,#30609,#30610),.UNSPECIFIED.,.F.,.F.,(4,1,1,1,1,1,
1,4),(53.4070751110264,53.7595776695398,54.7571490425228,55.7547204155057,
56.7522917884886,57.7498631614716,58.7474345344545,59.690260418206),
 .UNSPECIFIED.);
#2460=B_SPLINE_CURVE_WITH_KNOTS('',3,(#30611,#30612,#30613,#30614,#30615,
#30616,#30617,#30618,#30619,#30620),.UNSPECIFIED.,.F.,.F.,(4,1,1,1,1,1,
1,4),(53.4070751110264,54.3009959320942,55.2985673050771,56.2961386780601,
57.293710051043,58.2912814240259,59.2888527970089,59.690260418206),
 .UNSPECIFIED.);
#2461=B_SPLINE_CURVE_WITH_KNOTS('',3,(#30625,#30626,#30627,#30628,#30629,
#30630,#30631,#30632,#30633,#30634),.UNSPECIFIED.,.F.,.F.,(4,1,1,1,1,1,
1,4),(47.1238898038468,47.7741494316422,48.7717208046252,49.7692921776081,
50.766863550591,51.764434923574,52.7620062965569,53.4070751110264),
 .UNSPECIFIED.);
#2462=B_SPLINE_CURVE_WITH_KNOTS('',3,(#30635,#30636,#30637,#30638,#30639,
#30640,#30641,#30642,#30643,#30644,#30645),.UNSPECIFIED.,.F.,.F.,(4,1,1,
1,1,1,1,1,4),(47.1238898038468,47.3179963212137,48.3155676941966,49.3131390671795,
50.3107104401625,51.3082818131454,52.3058531861283,53.3034245591113,53.4070751110264),
 .UNSPECIFIED.);
#2463=B_SPLINE_CURVE_WITH_KNOTS('',3,(#30650,#30651,#30652,#30653,#30654,
#30655,#30656,#30657,#30658,#30659),.UNSPECIFIED.,.F.,.F.,(4,1,1,1,1,1,
1,4),(40.8407044966673,41.7887211937446,42.7862925667276,43.7838639397105,
44.7814353126934,45.7790066856764,46.7765780586593,47.1238898038468),
 .UNSPECIFIED.);
#2464=B_SPLINE_CURVE_WITH_KNOTS('',3,(#30660,#30661,#30662,#30663,#30664,
#30665,#30666,#30667,#30668,#30669),.UNSPECIFIED.,.F.,.F.,(4,1,1,1,1,1,
1,4),(40.8407044966673,41.3325680833161,42.330139456299,43.3277108292819,
44.3252822022649,45.3228535752478,46.3204249482307,47.1238898038468),
 .UNSPECIFIED.);
#2465=B_SPLINE_CURVE_WITH_KNOTS('',3,(#30674,#30675,#30676,#30677,#30678,
#30679,#30680,#30681,#30682,#30683,#30684),.UNSPECIFIED.,.F.,.F.,(4,1,1,
1,1,1,1,1,4),(34.5575191894876,34.8057215828641,35.803292955847,36.80086432883,
37.7984357018129,38.7960070747958,39.7935784477788,40.7911498207617,40.8407044966673),
 .UNSPECIFIED.);
#2466=B_SPLINE_CURVE_WITH_KNOTS('',3,(#30685,#30686,#30687,#30688,#30689,
#30690,#30691,#30692,#30693,#30694),.UNSPECIFIED.,.F.,.F.,(4,1,1,1,1,1,
1,4),(34.5575191894876,35.3471398454185,36.3447112184014,37.3422825913843,
38.3398539643673,39.3374253373502,40.3349967103331,40.8407044966673),
 .UNSPECIFIED.);
#2467=B_SPLINE_CURVE_WITH_KNOTS('',3,(#30699,#30700,#30701,#30702,#30703,
#30704,#30705,#30706,#30707,#30708),.UNSPECIFIED.,.F.,.F.,(4,1,1,1,1,1,
1,4),(28.2743338823081,28.8202933449665,29.8178647179494,30.8154360909324,
31.8130074639153,32.8105788368982,33.8081502098812,34.5575191894876),
 .UNSPECIFIED.);
#2468=B_SPLINE_CURVE_WITH_KNOTS('',3,(#30709,#30710,#30711,#30712,#30713,
#30714,#30715,#30716,#30717,#30718,#30719),.UNSPECIFIED.,.F.,.F.,(4,1,1,
1,1,1,1,1,4),(28.2743338823081,28.364140234538,29.3617116075209,30.3592829805038,
31.3568543534868,32.3544257264697,33.3519970994526,34.3495684724355,34.5575191894876),
 .UNSPECIFIED.);
#2469=B_SPLINE_CURVE_WITH_KNOTS('',3,(#30724,#30725,#30726,#30727,#30728,
#30729,#30730,#30731,#30732,#30733),.UNSPECIFIED.,.F.,.F.,(4,1,1,1,1,1,
1,4),(21.9911485751285,22.8348651070689,23.8324364800518,24.8300078530348,
25.8275792260177,26.8251505990006,27.8227219719836,28.2743338823081),
 .UNSPECIFIED.);
#2470=B_SPLINE_CURVE_WITH_KNOTS('',3,(#30734,#30735,#30736,#30737,#30738,
#30739,#30740,#30741,#30742,#30743),.UNSPECIFIED.,.F.,.F.,(4,1,1,1,1,1,
1,4),(21.9911485751285,22.3787119966404,23.3762833696233,24.3738547426062,
25.3714261155892,26.3689974885721,27.366568861555,28.2743338823081),
 .UNSPECIFIED.);
#2471=B_SPLINE_CURVE_WITH_KNOTS('',3,(#30749,#30750,#30751,#30752,#30753),
 .UNSPECIFIED.,.F.,.F.,(4,1,4),(14.3981410127769,15.3957123857598,15.7079632679489),
 .UNSPECIFIED.);
#2472=B_SPLINE_CURVE_WITH_KNOTS('',3,(#30756,#30757,#30758,#30759,#30760),
 .UNSPECIFIED.,.F.,.F.,(4,1,4),(13.8761928695311,14.8542941232054,15.7079632679489),
 .UNSPECIFIED.);
#2473=B_SPLINE_CURVE_WITH_KNOTS('',3,(#30766,#30767,#30768,#30769),
 .UNSPECIFIED.,.F.,.F.,(4,4),(114.40689867021,115.117908020989),
 .UNSPECIFIED.);
#2474=B_SPLINE_CURVE_WITH_KNOTS('',3,(#30777,#30778,#30779,#30780,#30781,
#30782,#30783,#30784,#30785,#30786),.UNSPECIFIED.,.F.,.F.,(4,3,3,4),(-113.097335529232,
-112.140720744584,-111.148324985783,-110.666752226423),.UNSPECIFIED.);
#2475=B_SPLINE_CURVE_WITH_KNOTS('',3,(#30791,#30792,#30793,#30794,#30795,
#30796,#30797,#30798,#30799,#30800,#30801,#30802,#30803,#30804,#30805,#30806,
#30807,#30808,#30809,#30810,#30811,#30812,#30813,#30814,#30815),
 .UNSPECIFIED.,.F.,.F.,(4,3,3,3,3,3,3,3,4),(108.12371336303,108.171137709378,
109.16353346818,110.155929226981,111.148324985783,112.140720744584,113.133116503386,
114.125512262188,114.40689867021),.UNSPECIFIED.);
#2476=B_SPLINE_CURVE_WITH_KNOTS('',3,(#30816,#30817,#30818,#30819,#30820,
#30821,#30822,#30823,#30824,#30825,#30826,#30827,#30828,#30829,#30830,#30831,
#30832,#30833,#30834,#30835,#30836,#30837),.UNSPECIFIED.,.F.,.F.,(4,3,3,
3,3,3,3,4),(-110.666752226423,-110.155929226981,-109.16353346818,-108.171137709378,
-107.178741950576,-106.186346191775,-105.193950432973,-104.383566919243),
 .UNSPECIFIED.);
#2477=B_SPLINE_CURVE_WITH_KNOTS('',3,(#30842,#30843,#30844,#30845,#30846,
#30847,#30848,#30849,#30850,#30851,#30852,#30853,#30854,#30855,#30856,#30857,
#30858,#30859,#30860,#30861,#30862,#30863),.UNSPECIFIED.,.F.,.F.,(4,3,3,
3,3,3,3,4),(101.84052805585,102.216763156568,103.20915891537,104.201554674171,
105.193950432973,106.186346191775,107.178741950576,108.12371336303),
 .UNSPECIFIED.);
#2478=B_SPLINE_CURVE_WITH_KNOTS('',3,(#30864,#30865,#30866,#30867,#30868,
#30869,#30870,#30871,#30872,#30873,#30874,#30875,#30876,#30877,#30878,#30879,
#30880,#30881,#30882,#30883,#30884,#30885,#30886,#30887,#30888),
 .UNSPECIFIED.,.F.,.F.,(4,3,3,3,3,3,3,3,4),(-104.383566919243,-104.201554674171,
-103.20915891537,-102.216763156568,-101.224367397767,-100.231971638965,
-99.2395758801633,-98.2471801213616,-98.1003816120635),.UNSPECIFIED.);
#2479=B_SPLINE_CURVE_WITH_KNOTS('',3,(#30893,#30894,#30895,#30896,#30897,
#30898,#30899,#30900,#30901,#30902,#30903,#30904,#30905,#30906,#30907,#30908,
#30909,#30910,#30911,#30912,#30913,#30914),.UNSPECIFIED.,.F.,.F.,(4,3,3,
3,3,3,3,4),(95.5573427486709,96.2623886037584,97.25478436256,98.2471801213616,
99.2395758801633,100.231971638965,101.224367397767,101.84052805585),
 .UNSPECIFIED.);
#2480=B_SPLINE_CURVE_WITH_KNOTS('',3,(#30915,#30916,#30917,#30918,#30919,
#30920,#30921,#30922,#30923,#30924,#30925,#30926,#30927,#30928,#30929,#30930,
#30931,#30932,#30933,#30934,#30935,#30936),.UNSPECIFIED.,.F.,.F.,(4,3,3,
3,3,3,3,4),(-98.1003816120635,-97.25478436256,-96.2623886037584,-95.2699928449567,
-94.2775970861551,-93.2852013273535,-92.2928055685519,-91.8171963048839),
 .UNSPECIFIED.);
#2481=B_SPLINE_CURVE_WITH_KNOTS('',3,(#30941,#30942,#30943,#30944,#30945,
#30946,#30947,#30948,#30949,#30950,#30951,#30952,#30953,#30954,#30955,#30956,
#30957,#30958,#30959,#30960,#30961,#30962,#30963,#30964,#30965),
 .UNSPECIFIED.,.F.,.F.,(4,3,3,3,3,3,3,3,4),(89.2741574414912,89.3156182921469,
90.3080140509486,91.3004098097502,92.2928055685518,93.2852013273535,94.2775970861551,
95.2699928449567,95.5573427486709),.UNSPECIFIED.);
#2482=B_SPLINE_CURVE_WITH_KNOTS('',3,(#30966,#30967,#30968,#30969,#30970,
#30971,#30972,#30973,#30974,#30975,#30976,#30977,#30978,#30979,#30980,#30981,
#30982,#30983,#30984,#30985,#30986,#30987),.UNSPECIFIED.,.F.,.F.,(4,3,3,
3,3,3,3,4),(-91.8171963048839,-91.3004098097502,-90.3080140509486,-89.315618292147,
-88.3232225333453,-87.3308267745437,-86.338431015742,-85.5340109977043),
 .UNSPECIFIED.);
#2483=B_SPLINE_CURVE_WITH_KNOTS('',3,(#30992,#30993,#30994,#30995,#30996,
#30997,#30998,#30999,#31000,#31001,#31002,#31003,#31004,#31005,#31006,#31007,
#31008,#31009,#31010,#31011,#31012,#31013),.UNSPECIFIED.,.F.,.F.,(4,3,3,
3,3,3,3,4),(82.9909721343117,83.3612437393372,84.3536394981388,85.3460352569404,
86.338431015742,87.3308267745437,88.3232225333453,89.2741574414912),
 .UNSPECIFIED.);
#2484=B_SPLINE_CURVE_WITH_KNOTS('',3,(#31014,#31015,#31016,#31017,#31018,
#31019,#31020,#31021,#31022,#31023,#31024,#31025,#31026,#31027,#31028,#31029,
#31030,#31031,#31032,#31033,#31034,#31035,#31036,#31037,#31038),
 .UNSPECIFIED.,.F.,.F.,(4,3,3,3,3,3,3,3,4),(-85.5340109977043,-85.3460352569404,
-84.3536394981388,-83.3612437393372,-82.3688479805355,-81.3764522217339,
-80.3840564629323,-79.3916607041306,-79.2508256905247),.UNSPECIFIED.);
#2485=B_SPLINE_CURVE_WITH_KNOTS('',3,(#31043,#31044,#31045,#31046,#31047,
#31048,#31049,#31050,#31051,#31052,#31053,#31054,#31055,#31056,#31057,#31058,
#31059,#31060,#31061,#31062,#31063,#31064),.UNSPECIFIED.,.F.,.F.,(4,3,3,
3,3,3,3,4),(76.7077868271321,77.4068691865273,78.399264945329,79.3916607041306,
80.3840564629322,81.3764522217339,82.3688479805355,82.9909721343117),
 .UNSPECIFIED.);
#2486=B_SPLINE_CURVE_WITH_KNOTS('',3,(#31065,#31066,#31067,#31068,#31069,
#31070,#31071,#31072,#31073,#31074,#31075,#31076,#31077,#31078,#31079,#31080,
#31081,#31082,#31083,#31084,#31085,#31086),.UNSPECIFIED.,.F.,.F.,(4,3,3,
3,3,3,3,4),(-79.2508256905247,-78.399264945329,-77.4068691865274,-76.4144734277257,
-75.4220776689241,-74.4296819101224,-73.4372861513208,-72.9676403833451),
 .UNSPECIFIED.);
#2487=B_SPLINE_CURVE_WITH_KNOTS('',3,(#31091,#31092,#31093,#31094,#31095,
#31096,#31097,#31098,#31099,#31100,#31101,#31102,#31103,#31104,#31105,#31106,
#31107,#31108,#31109,#31110,#31111,#31112,#31113,#31114,#31115),
 .UNSPECIFIED.,.F.,.F.,(4,3,3,3,3,3,3,3,4),(70.4246015199525,70.4600988749159,
71.4524946337175,72.4448903925192,73.4372861513208,74.4296819101224,75.4220776689241,
76.4144734277257,76.7077868271321),.UNSPECIFIED.);
#2488=B_SPLINE_CURVE_WITH_KNOTS('',3,(#31116,#31117,#31118,#31119,#31120,
#31121,#31122,#31123,#31124,#31125,#31126,#31127,#31128,#31129,#31130,#31131,
#31132,#31133,#31134,#31135,#31136,#31137),.UNSPECIFIED.,.F.,.F.,(4,3,3,
3,3,3,3,4),(-72.9676403833451,-72.4448903925192,-71.4524946337175,-70.4600988749159,
-69.4677031161143,-68.4753073573127,-67.482911598511,-66.6844550761655),
 .UNSPECIFIED.);
#2489=B_SPLINE_CURVE_WITH_KNOTS('',3,(#31142,#31143,#31144,#31145,#31146,
#31147,#31148,#31149,#31150,#31151,#31152,#31153,#31154,#31155,#31156,#31157,
#31158,#31159,#31160,#31161,#31162,#31163),.UNSPECIFIED.,.F.,.F.,(4,3,3,
3,3,3,3,4),(64.1414162127729,64.5057243221061,65.4981200809078,66.4905158397094,
67.482911598511,68.4753073573126,69.4677031161143,70.4246015199525),
 .UNSPECIFIED.);
#2490=B_SPLINE_CURVE_WITH_KNOTS('',3,(#31164,#31165,#31166,#31167,#31168,
#31169,#31170,#31171,#31172,#31173,#31174,#31175,#31176,#31177,#31178,#31179,
#31180,#31181,#31182,#31183,#31184,#31185,#31186,#31187,#31188),
 .UNSPECIFIED.,.F.,.F.,(4,3,3,3,3,3,3,3,4),(-66.6844550761655,-66.4905158397094,
-65.4981200809078,-64.5057243221061,-63.5133285633045,-62.5209328045029,
-61.5285370457012,-60.5361412868996,-60.4012697689859),.UNSPECIFIED.);
#2491=B_SPLINE_CURVE_WITH_KNOTS('',3,(#31193,#31194,#31195,#31196,#31197,
#31198,#31199,#31200,#31201,#31202,#31203,#31204,#31205,#31206,#31207,#31208,
#31209,#31210,#31211,#31212,#31213,#31214),.UNSPECIFIED.,.F.,.F.,(4,3,3,
3,3,3,3,4),(57.8582309055933,58.5513497692963,59.543745528098,60.5361412868996,
61.5285370457012,62.5209328045029,63.5133285633045,64.1414162127729),
 .UNSPECIFIED.);
#2492=B_SPLINE_CURVE_WITH_KNOTS('',3,(#31215,#31216,#31217,#31218,#31219,
#31220,#31221,#31222,#31223,#31224,#31225,#31226,#31227,#31228,#31229,#31230,
#31231,#31232,#31233,#31234,#31235,#31236),.UNSPECIFIED.,.F.,.F.,(4,3,3,
3,3,3,3,4),(-60.4012697689859,-59.543745528098,-58.5513497692964,-57.5589540104947,
-56.5665582516931,-55.5741624928914,-54.5817667340898,-54.1180844618063),
 .UNSPECIFIED.);
#2493=B_SPLINE_CURVE_WITH_KNOTS('',3,(#31241,#31242,#31243,#31244,#31245,
#31246,#31247,#31248,#31249,#31250,#31251,#31252,#31253,#31254,#31255,#31256,
#31257,#31258,#31259,#31260,#31261,#31262,#31263,#31264,#31265),
 .UNSPECIFIED.,.F.,.F.,(4,3,3,3,3,3,3,3,4),(51.5750455984137,51.6045794576849,
52.5969752164865,53.5893709752882,54.5817667340898,55.5741624928914,56.5665582516931,
57.5589540104947,57.8582309055933),.UNSPECIFIED.);
#2494=B_SPLINE_CURVE_WITH_KNOTS('',3,(#31266,#31267,#31268,#31269,#31270,
#31271,#31272,#31273,#31274,#31275,#31276,#31277,#31278,#31279,#31280,#31281,
#31282,#31283,#31284,#31285,#31286,#31287),.UNSPECIFIED.,.F.,.F.,(4,3,3,
3,3,3,3,4),(-54.1180844618063,-53.5893709752882,-52.5969752164865,-51.6045794576849,
-50.6121836988833,-49.6197879400816,-48.62739218128,-47.8348991546267),
 .UNSPECIFIED.);
#2495=B_SPLINE_CURVE_WITH_KNOTS('',3,(#31292,#31293,#31294,#31295,#31296,
#31297,#31298,#31299,#31300,#31301,#31302,#31303,#31304,#31305,#31306,#31307,
#31308,#31309,#31310,#31311,#31312,#31313),.UNSPECIFIED.,.F.,.F.,(4,3,3,
3,3,3,3,4),(45.2918602912341,45.6502049048751,46.6426006636767,47.6349964224784,
48.62739218128,49.6197879400816,50.6121836988833,51.5750455984137),
 .UNSPECIFIED.);
#2496=B_SPLINE_CURVE_WITH_KNOTS('',3,(#31314,#31315,#31316,#31317,#31318,
#31319,#31320,#31321,#31322,#31323,#31324,#31325,#31326,#31327,#31328,#31329,
#31330,#31331,#31332,#31333,#31334,#31335,#31336,#31337,#31338),
 .UNSPECIFIED.,.F.,.F.,(4,3,3,3,3,3,3,3,4),(-47.8348991546267,-47.6349964224784,
-46.6426006636767,-45.6502049048751,-44.6578091460735,-43.6654133872718,
-42.6730176284702,-41.6806218696686,-41.5517138474472),.UNSPECIFIED.);
#2497=B_SPLINE_CURVE_WITH_KNOTS('',3,(#31343,#31344,#31345,#31346,#31347,
#31348,#31349,#31350,#31351,#31352,#31353,#31354,#31355,#31356,#31357,#31358,
#31359,#31360,#31361,#31362,#31363,#31364),.UNSPECIFIED.,.F.,.F.,(4,3,3,
3,3,3,3,4),(39.0086749840545,39.6958303520653,40.6882261108669,41.6806218696686,
42.6730176284702,43.6654133872718,44.6578091460735,45.2918602912341),
 .UNSPECIFIED.);
#2498=B_SPLINE_CURVE_WITH_KNOTS('',3,(#31365,#31366,#31367,#31368,#31369,
#31370,#31371,#31372,#31373,#31374,#31375,#31376,#31377,#31378,#31379,#31380,
#31381,#31382,#31383,#31384,#31385,#31386),.UNSPECIFIED.,.F.,.F.,(4,3,3,
3,3,3,3,4),(-41.5517138474472,-40.6882261108669,-39.6958303520653,-38.7034345932637,
-37.711038834462,-36.7186430756604,-35.7262473168588,-35.2685285402675),
 .UNSPECIFIED.);
#2499=B_SPLINE_CURVE_WITH_KNOTS('',3,(#31391,#31392,#31393,#31394,#31395,
#31396,#31397,#31398,#31399,#31400,#31401,#31402,#31403,#31404,#31405,#31406,
#31407,#31408,#31409,#31410,#31411,#31412,#31413,#31414,#31415),
 .UNSPECIFIED.,.F.,.F.,(4,3,3,3,3,3,3,3,4),(32.725489676875,32.7490600404539,
33.7414557992555,34.7338515580571,35.7262473168588,36.7186430756604,37.711038834462,
38.7034345932637,39.0086749840545),.UNSPECIFIED.);
#2500=B_SPLINE_CURVE_WITH_KNOTS('',3,(#31416,#31417,#31418,#31419,#31420,
#31421,#31422,#31423,#31424,#31425,#31426,#31427,#31428,#31429,#31430,#31431,
#31432,#31433,#31434,#31435,#31436,#31437),.UNSPECIFIED.,.F.,.F.,(4,3,3,
3,3,3,3,4),(-35.2685285402675,-34.7338515580572,-33.7414557992555,-32.7490600404539,
-31.7566642816523,-30.7642685228506,-29.771872764049,-28.985343233088),
 .UNSPECIFIED.);
#2501=B_SPLINE_CURVE_WITH_KNOTS('',3,(#31442,#31443,#31444,#31445,#31446,
#31447,#31448,#31449,#31450,#31451,#31452,#31453,#31454,#31455,#31456,#31457,
#31458,#31459,#31460,#31461,#31462,#31463),.UNSPECIFIED.,.F.,.F.,(4,3,3,
3,3,3,3,4),(26.4423043696953,26.7946854876441,27.7870812464457,28.7794770052473,
29.771872764049,30.7642685228506,31.7566642816522,32.725489676875),
 .UNSPECIFIED.);
#2502=B_SPLINE_CURVE_WITH_KNOTS('',3,(#31464,#31465,#31466,#31467,#31468,
#31469,#31470,#31471,#31472,#31473,#31474,#31475,#31476,#31477,#31478,#31479,
#31480,#31481,#31482,#31483,#31484,#31485,#31486,#31487,#31488),
 .UNSPECIFIED.,.F.,.F.,(4,3,3,3,3,3,3,3,4),(-28.985343233088,-28.7794770052474,
-27.7870812464457,-26.7946854876441,-25.8022897288425,-24.8098939700408,
-23.8174982112392,-22.8251024524376,-22.7021579259084),.UNSPECIFIED.);
#2503=B_SPLINE_CURVE_WITH_KNOTS('',3,(#31493,#31494,#31495,#31496,#31497,
#31498,#31499,#31500,#31501,#31502,#31503,#31504,#31505,#31506,#31507,#31508,
#31509,#31510,#31511,#31512,#31513,#31514),.UNSPECIFIED.,.F.,.F.,(4,3,3,
3,3,3,3,4),(20.1591190625158,20.8403109348343,21.8327066936359,22.8251024524376,
23.8174982112392,24.8098939700408,25.8022897288424,26.4423043696953),
 .UNSPECIFIED.);
#2504=B_SPLINE_CURVE_WITH_KNOTS('',3,(#31515,#31516,#31517,#31518,#31519,
#31520,#31521,#31522,#31523,#31524,#31525,#31526,#31527,#31528,#31529,#31530,
#31531,#31532,#31533,#31534,#31535,#31536),.UNSPECIFIED.,.F.,.F.,(4,3,3,
3,3,3,3,4),(-22.7021579259084,-21.8327066936359,-20.8403109348343,-19.8479151760327,
-18.855519417231,-17.8631236584294,-16.8707278996278,-16.4189726187288),
 .UNSPECIFIED.);
#2505=B_SPLINE_CURVE_WITH_KNOTS('',3,(#31541,#31542,#31543,#31544,#31545,
#31546,#31547,#31548,#31549,#31550,#31551,#31552,#31553,#31554,#31555,#31556,
#31557,#31558,#31559,#31560,#31561,#31562,#31563,#31564,#31565),
 .UNSPECIFIED.,.F.,.F.,(4,3,3,3,3,3,3,3,4),(13.8759337553361,13.8935406232229,
14.8859363820245,15.8783321408261,16.8707278996278,17.8631236584294,18.855519417231,
19.8479151760327,20.1591190625158),.UNSPECIFIED.);
#2506=B_SPLINE_CURVE_WITH_KNOTS('',3,(#31566,#31567,#31568,#31569,#31570,
#31571,#31572,#31573,#31574,#31575,#31576,#31577,#31578,#31579,#31580,#31581,
#31582,#31583,#31584,#31585,#31586,#31587),.UNSPECIFIED.,.F.,.F.,(4,3,3,
3,3,3,3,4),(-16.4189726187288,-15.8783321408261,-14.8859363820245,-13.8935406232229,
-12.9011448644212,-11.9087491056196,-10.916353346818,-10.1357873115492),
 .UNSPECIFIED.);
#2507=B_SPLINE_CURVE_WITH_KNOTS('',3,(#31593,#31594,#31595,#31596,#31597,
#31598,#31599,#31600,#31601,#31602,#31603,#31604,#31605),.UNSPECIFIED.,
 .F.,.F.,(4,3,3,3,4),(-3.85260200436961,-2.9771872764049,-1.98479151760327,
-0.992395758801633,0.),.UNSPECIFIED.);
#2508=B_SPLINE_CURVE_WITH_KNOTS('',3,(#31608,#31609,#31610,#31611,#31612,
#31613,#31614,#31615,#31616,#31617,#31618,#31619,#31620,#31621,#31622,#31623,
#31624,#31625,#31626),.UNSPECIFIED.,.F.,.F.,(4,3,3,3,3,3,4),(2.0205724917569,
2.9771872764049,3.96958303520653,4.96197879400816,5.9543745528098,6.94677031161143,
7.59274844815659),.UNSPECIFIED.);
#2509=B_SPLINE_CURVE_WITH_KNOTS('',3,(#31632,#31633,#31634,#31635,#31636,
#31637,#31638,#31639),.UNSPECIFIED.,.F.,.F.,(4,1,1,1,1,4),(122.522113490002,
123.003686249362,123.996082008164,124.988477766965,125.980873525767,126.973269284569),
 .UNSPECIFIED.);
#2510=B_SPLINE_CURVE_WITH_KNOTS('',3,(#31642,#31643,#31644,#31645,#31646,
#31647,#31648,#31649,#31650),.UNSPECIFIED.,.F.,.F.,(4,1,1,1,1,1,4),(122.522113490002,
122.56953783635,123.561933595151,124.554329353953,125.546725112755,126.539120871556,
127.495735656204),.UNSPECIFIED.);
#2511=B_SPLINE_CURVE_WITH_KNOTS('',3,(#31655,#31656,#31657,#31658,#31659,
#31660,#31661,#31662,#31663,#31664),.UNSPECIFIED.,.F.,.F.,(4,1,1,1,1,1,
1,4),(116.238928182822,117.049311696552,118.041707455354,119.034103214156,
120.026498972957,121.018894731759,122.01129049056,122.522113490002),
 .UNSPECIFIED.);
#2512=B_SPLINE_CURVE_WITH_KNOTS('',3,(#31665,#31666,#31667,#31668,#31669,
#31670,#31671,#31672,#31673,#31674),.UNSPECIFIED.,.F.,.F.,(4,1,1,1,1,1,
1,4),(116.238928182822,116.61516328354,117.607559042342,118.599954801143,
119.592350559945,120.584746318746,121.577142077548,122.522113490002),
 .UNSPECIFIED.);
#2513=B_SPLINE_CURVE_WITH_KNOTS('',3,(#31679,#31680,#31681,#31682,#31683,
#31684,#31685,#31686,#31687,#31688,#31689),.UNSPECIFIED.,.F.,.F.,(4,1,1,
1,1,1,1,1,4),(109.955742875643,110.102541384941,111.094937143743,112.087332902544,
113.079728661346,114.072124420147,115.064520178949,116.056915937751,116.238928182822),
 .UNSPECIFIED.);
#2514=B_SPLINE_CURVE_WITH_KNOTS('',3,(#31690,#31691,#31692,#31693,#31694,
#31695,#31696,#31697,#31698,#31699),.UNSPECIFIED.,.F.,.F.,(4,1,1,1,1,1,
1,4),(109.955742875643,110.66078873073,111.653184489532,112.645580248333,
113.637976007135,114.630371765937,115.622767524738,116.238928182822),
 .UNSPECIFIED.);
#2515=B_SPLINE_CURVE_WITH_KNOTS('',3,(#31704,#31705,#31706,#31707,#31708,
#31709,#31710,#31711,#31712,#31713),.UNSPECIFIED.,.F.,.F.,(4,1,1,1,1,1,
1,4),(103.672557568463,104.148166832131,105.140562590933,106.132958349734,
107.125354108536,108.117749867338,109.110145626139,109.955742875643),
 .UNSPECIFIED.);
#2516=B_SPLINE_CURVE_WITH_KNOTS('',3,(#31714,#31715,#31716,#31717,#31718,
#31719,#31720,#31721,#31722,#31723,#31724),.UNSPECIFIED.,.F.,.F.,(4,1,1,
1,1,1,1,1,4),(103.672557568463,103.714018419119,104.70641417792,105.698809936722,
106.691205695524,107.683601454325,108.675997213127,109.668392971929,109.955742875643),
 .UNSPECIFIED.);
#2517=B_SPLINE_CURVE_WITH_KNOTS('',3,(#31729,#31730,#31731,#31732,#31733,
#31734,#31735,#31736,#31737,#31738),.UNSPECIFIED.,.F.,.F.,(4,1,1,1,1,1,
1,4),(97.3893722612835,98.1937922793213,99.1861880381229,100.178583796925,
101.170979555726,102.163375314528,103.155771073329,103.672557568463),
 .UNSPECIFIED.);
#2518=B_SPLINE_CURVE_WITH_KNOTS('',3,(#31739,#31740,#31741,#31742,#31743,
#31744,#31745,#31746,#31747,#31748),.UNSPECIFIED.,.F.,.F.,(4,1,1,1,1,1,
1,4),(97.3893722612835,97.7596438663089,98.7520396251105,99.7444353839122,
100.736831142714,101.729226901515,102.721622660317,103.672557568463),
 .UNSPECIFIED.);
#2519=B_SPLINE_CURVE_WITH_KNOTS('',3,(#31753,#31754,#31755,#31756,#31757,
#31758,#31759,#31760,#31761,#31762,#31763),.UNSPECIFIED.,.F.,.F.,(4,1,1,
1,1,1,1,1,4),(91.106186954104,91.2470219677099,92.2394177265115,93.2318134853131,
94.2242092441148,95.2166050029164,96.209000761718,97.2013965205197,97.3893722612835),
 .UNSPECIFIED.);
#2520=B_SPLINE_CURVE_WITH_KNOTS('',3,(#31764,#31765,#31766,#31767,#31768,
#31769,#31770,#31771,#31772,#31773),.UNSPECIFIED.,.F.,.F.,(4,1,1,1,1,1,
1,4),(91.106186954104,91.8052693134991,92.7976650723007,93.7900608311024,
94.782456589904,95.7748523487057,96.7672481075073,97.3893722612835),
 .UNSPECIFIED.);
#2521=B_SPLINE_CURVE_WITH_KNOTS('',3,(#31778,#31779,#31780,#31781,#31782,
#31783,#31784,#31785,#31786,#31787),.UNSPECIFIED.,.F.,.F.,(4,1,1,1,1,1,
1,4),(84.8230016469243,85.2926474149001,86.2850431737017,87.2774389325033,
88.269834691305,89.2622304501066,90.2546262089082,91.106186954104),
 .UNSPECIFIED.);
#2522=B_SPLINE_CURVE_WITH_KNOTS('',3,(#31788,#31789,#31790,#31791,#31792,
#31793,#31794,#31795,#31796,#31797,#31798),.UNSPECIFIED.,.F.,.F.,(4,1,1,
1,1,1,1,1,4),(84.8230016469243,84.8584990018877,85.8508947606893,86.8432905194909,
87.8356862782926,88.8280820370942,89.8204777958959,90.8128735546975,91.106186954104),
 .UNSPECIFIED.);
#2523=B_SPLINE_CURVE_WITH_KNOTS('',3,(#31803,#31804,#31805,#31806,#31807,
#31808,#31809,#31810,#31811,#31812),.UNSPECIFIED.,.F.,.F.,(4,1,1,1,1,1,
1,4),(78.5398163397448,79.3382728620903,80.3306686208919,81.3230643796935,
82.3154601384952,83.3078558972968,84.3002516560985,84.8230016469243),
 .UNSPECIFIED.);
#2524=B_SPLINE_CURVE_WITH_KNOTS('',3,(#31813,#31814,#31815,#31816,#31817,
#31818,#31819,#31820,#31821,#31822),.UNSPECIFIED.,.F.,.F.,(4,1,1,1,1,1,
1,4),(78.5398163397448,78.9041244490779,79.8965202078795,80.8889159666812,
81.8813117254828,82.8737074842844,83.8661032430861,84.8230016469243),
 .UNSPECIFIED.);
#2525=B_SPLINE_CURVE_WITH_KNOTS('',3,(#31827,#31828,#31829,#31830,#31831,
#31832,#31833,#31834,#31835,#31836,#31837),.UNSPECIFIED.,.F.,.F.,(4,1,1,
1,1,1,1,1,4),(72.2566310325651,72.3915025504788,73.3838983092805,74.3762940680821,
75.3686898268838,76.3610855856854,77.353481344487,78.3458771032886,78.5398163397448),
 .UNSPECIFIED.);
#2526=B_SPLINE_CURVE_WITH_KNOTS('',3,(#31838,#31839,#31840,#31841,#31842,
#31843,#31844,#31845,#31846,#31847),.UNSPECIFIED.,.F.,.F.,(4,1,1,1,1,1,
1,4),(72.2566310325651,72.9497498962681,73.9421456550697,74.9345414138714,
75.926937172673,76.9193329314746,77.9117286902763,78.5398163397448),
 .UNSPECIFIED.);
#2527=B_SPLINE_CURVE_WITH_KNOTS('',3,(#31852,#31853,#31854,#31855,#31856,
#31857,#31858,#31859,#31860,#31861),.UNSPECIFIED.,.F.,.F.,(4,1,1,1,1,1,
1,4),(65.9734457253856,66.4371279976691,67.4295237564707,68.4219195152723,
69.4143152740739,70.4067110328756,71.3991067916772,72.2566310325651),
 .UNSPECIFIED.);
#2528=B_SPLINE_CURVE_WITH_KNOTS('',3,(#31862,#31863,#31864,#31865,#31866,
#31867,#31868,#31869,#31870,#31871,#31872),.UNSPECIFIED.,.F.,.F.,(4,1,1,
1,1,1,1,1,4),(65.9734457253856,66.0029795846567,66.9953753434583,67.9877711022599,
68.9801668610616,69.9725626198632,70.9649583786648,71.9573541374665,72.2566310325651),
 .UNSPECIFIED.);
#2529=B_SPLINE_CURVE_WITH_KNOTS('',3,(#31877,#31878,#31879,#31880,#31881,
#31882,#31883,#31884,#31885,#31886),.UNSPECIFIED.,.F.,.F.,(4,1,1,1,1,1,
1,4),(59.690260418206,60.4827534448593,61.4751492036609,62.4675449624625,
63.4599407212642,64.4523364800658,65.4447322388674,65.9734457253856),
 .UNSPECIFIED.);
#2530=B_SPLINE_CURVE_WITH_KNOTS('',3,(#31887,#31888,#31889,#31890,#31891,
#31892,#31893,#31894,#31895,#31896),.UNSPECIFIED.,.F.,.F.,(4,1,1,1,1,1,
1,4),(59.690260418206,60.0486050318469,61.0410007906485,62.0333965494501,
63.0257923082518,64.0181880670534,65.010583825855,65.9734457253856),
 .UNSPECIFIED.);
#2531=B_SPLINE_CURVE_WITH_KNOTS('',3,(#31901,#31902,#31903,#31904,#31905,
#31906,#31907,#31908,#31909,#31910,#31911),.UNSPECIFIED.,.F.,.F.,(4,1,1,
1,1,1,1,1,4),(53.4070751110264,53.5359831332478,54.5283788920495,55.5207746508511,
56.5131704096527,57.5055661684544,58.497961927256,59.4903576860576,59.690260418206),
 .UNSPECIFIED.);
#2532=B_SPLINE_CURVE_WITH_KNOTS('',3,(#31912,#31913,#31914,#31915,#31916,
#31917,#31918,#31919,#31920,#31921),.UNSPECIFIED.,.F.,.F.,(4,1,1,1,1,1,
1,4),(53.4070751110264,54.0942304790371,55.0866262378387,56.0790219966403,
57.071417755442,58.0638135142436,59.0562092730452,59.690260418206),
 .UNSPECIFIED.);
#2533=B_SPLINE_CURVE_WITH_KNOTS('',3,(#31926,#31927,#31928,#31929,#31930,
#31931,#31932,#31933,#31934,#31935),.UNSPECIFIED.,.F.,.F.,(4,1,1,1,1,1,
1,4),(47.1238898038468,47.581608580438,48.5740043392397,49.5664000980413,
50.5587958568429,51.5511916156446,52.5435873744462,53.4070751110264),
 .UNSPECIFIED.);
#2534=B_SPLINE_CURVE_WITH_KNOTS('',3,(#31936,#31937,#31938,#31939,#31940,
#31941,#31942,#31943,#31944,#31945,#31946),.UNSPECIFIED.,.F.,.F.,(4,1,1,
1,1,1,1,1,4),(47.1238898038468,47.1474601674257,48.1398559262273,49.1322516850289,
50.1246474438306,51.1170432026322,52.1094389614338,53.1018347202355,53.4070751110264),
 .UNSPECIFIED.);
#2535=B_SPLINE_CURVE_WITH_KNOTS('',3,(#31951,#31952,#31953,#31954,#31955,
#31956,#31957,#31958,#31959,#31960),.UNSPECIFIED.,.F.,.F.,(4,1,1,1,1,1,
1,4),(40.8407044966672,41.6272340276282,42.6196297864299,43.6120255452315,
44.6044213040331,45.5968170628348,46.5892128216364,47.1238898038468),
 .UNSPECIFIED.);
#2536=B_SPLINE_CURVE_WITH_KNOTS('',3,(#31961,#31962,#31963,#31964,#31965,
#31966,#31967,#31968,#31969,#31970),.UNSPECIFIED.,.F.,.F.,(4,1,1,1,1,1,
1,4),(40.8407044966672,41.1930856146159,42.1854813734175,43.1778771322191,
44.1702728910208,45.1626686498224,46.155064408624,47.1238898038468),
 .UNSPECIFIED.);
#2537=B_SPLINE_CURVE_WITH_KNOTS('',3,(#31975,#31976,#31977,#31978,#31979,
#31980,#31981,#31982,#31983,#31984,#31985),.UNSPECIFIED.,.F.,.F.,(4,1,1,
1,1,1,1,1,4),(34.5575191894876,34.6804637160168,35.6728594748184,36.6652552336201,
37.6576509924217,38.6500467512233,39.642442510025,40.6348382688266,40.8407044966672),
 .UNSPECIFIED.);
#2538=B_SPLINE_CURVE_WITH_KNOTS('',3,(#31986,#31987,#31988,#31989,#31990,
#31991,#31992,#31993,#31994,#31995),.UNSPECIFIED.,.F.,.F.,(4,1,1,1,1,1,
1,4),(34.5575191894876,35.2387110618061,36.2311068206077,37.2235025794093,
38.215898338211,39.2082940970126,40.2006898558142,40.8407044966672),
 .UNSPECIFIED.);
#2539=B_SPLINE_CURVE_WITH_KNOTS('',3,(#32000,#32001,#32002,#32003,#32004,
#32005,#32006,#32007,#32008,#32009),.UNSPECIFIED.,.F.,.F.,(4,1,1,1,1,1,
1,4),(28.274333882308,28.726089163207,29.7184849220086,30.7108806808103,
31.7032764396119,32.6956721984135,33.6880679572152,34.5575191894876),
 .UNSPECIFIED.);
#2540=B_SPLINE_CURVE_WITH_KNOTS('',3,(#32010,#32011,#32012,#32013,#32014,
#32015,#32016,#32017,#32018,#32019,#32020),.UNSPECIFIED.,.F.,.F.,(4,1,1,
1,1,1,1,1,4),(28.274333882308,28.2919407501946,29.2843365089963,30.2767322677979,
31.2691280265995,32.2615237854012,33.2539195442028,34.2463153030044,34.5575191894876),
 .UNSPECIFIED.);
#2541=B_SPLINE_CURVE_WITH_KNOTS('',3,(#32025,#32026,#32027,#32028,#32029,
#32030,#32031,#32032,#32033,#32034),.UNSPECIFIED.,.F.,.F.,(4,1,1,1,1,1,
1,4),(21.9911485751284,22.7717146103972,23.7641103691988,24.7565061280005,
25.7489018868021,26.7412976456037,27.7336934044054,28.274333882308),
 .UNSPECIFIED.);
#2542=B_SPLINE_CURVE_WITH_KNOTS('',3,(#32035,#32036,#32037,#32038,#32039,
#32040,#32041,#32042,#32043,#32044),.UNSPECIFIED.,.F.,.F.,(4,1,1,1,1,1,
1,4),(21.9911485751284,22.3375661973848,23.3299619561865,24.3223577149881,
25.3147534737897,26.3071492325914,27.299544991393,28.274333882308),
 .UNSPECIFIED.);
#2543=B_SPLINE_CURVE_WITH_KNOTS('',3,(#32050,#32051,#32052,#32053,#32054),
 .UNSPECIFIED.,.F.,.F.,(4,1,4),(14.3984001269718,15.3907958857734,15.7079632679489),
 .UNSPECIFIED.);
#2544=B_SPLINE_CURVE_WITH_KNOTS('',3,(#32057,#32058,#32059,#32060,#32061),
 .UNSPECIFIED.,.F.,.F.,(4,1,4),(13.8759337553361,14.8325485399841,15.7079632679489),
 .UNSPECIFIED.);
#2545=B_SPLINE_CURVE_WITH_KNOTS('',3,(#32063,#32064,#32065,#32066,#32067,
#32068,#32069,#32070,#32071,#32072,#32073,#32074,#32075,#32076,#32077,#32078,
#32079,#32080,#32081,#32082,#32083,#32084,#32085,#32086,#32087,#32088,#32089,
#32090,#32091,#32092,#32093,#32094,#32095,#32096,#32097,#32098,#32099,#32100,
#32101,#32102,#32103,#32104,#32105,#32106,#32107,#32108,#32109,#32110,#32111,
#32112,#32113,#32114),.UNSPECIFIED.,.F.,.F.,(4,3,3,3,3,3,3,3,3,3,3,3,3,
3,3,3,3,4),(-0.286347380332279,-0.266347789416864,-0.254098115456061,-0.230501751705225,
-0.216536610693349,-0.18668269284242,-0.173443188538191,-0.164130900566406,
-0.152678732927651,-0.129952909210668,-0.116365164485228,-0.106745630798174,
-0.0814440134366876,-0.0640046809373957,-0.0520446962100768,-0.0197039455308333,
-0.00553916135222766,0.),.UNSPECIFIED.);
#2546=B_SPLINE_CURVE_WITH_KNOTS('',3,(#32115,#32116,#32117,#32118,#32119,
#32120,#32121,#32122,#32123,#32124,#32125,#32126,#32127,#32128,#32129,#32130,
#32131,#32132,#32133,#32134,#32135,#32136,#32137,#32138,#32139,#32140,#32141,
#32142,#32143,#32144,#32145,#32146,#32147,#32148,#32149,#32150,#32151,#32152,
#32153,#32154,#32155,#32156,#32157,#32158,#32159,#32160,#32161,#32162,#32163,
#32164,#32165,#32166,#32167,#32168,#32169),.UNSPECIFIED.,.F.,.F.,(4,3,3,
3,3,3,3,3,3,3,3,3,3,3,3,3,3,3,4),(-0.2851428039951,-0.264876660632172,-0.2498967274825,
-0.236025660645345,-0.214587312757531,-0.204671023974553,-0.173775777047669,
-0.160111619860766,-0.150128525406277,-0.138317788758425,-0.118237251615849,
-0.10321155298755,-0.092840846421164,-0.0707715126256338,-0.0558839316601653,
-0.043797399607841,-0.0161434201156718,-0.00456351123904309,0.),
 .UNSPECIFIED.);
#2547=B_SPLINE_CURVE_WITH_KNOTS('',3,(#32171,#32172,#32173,#32174,#32175,
#32176,#32177,#32178,#32179,#32180,#32181),.UNSPECIFIED.,.F.,.F.,(4,1,1,
1,1,1,1,1,4),(15.7079632679489,15.8249442987858,16.8173400575874,17.809735816389,
18.8021315751907,19.7945273339923,20.7869230927939,21.7793188515956,21.9911485751284),
 .UNSPECIFIED.);
#2548=B_SPLINE_CURVE_WITH_KNOTS('',3,(#32182,#32183,#32184,#32185,#32186,
#32187,#32188,#32189,#32190,#32191),.UNSPECIFIED.,.F.,.F.,(4,1,1,1,1,1,
1,4),(15.7079632679489,16.383191644575,17.3755874033767,18.3679831621783,
19.3603789209799,20.3527746797816,21.3451704385832,21.9911485751284),
 .UNSPECIFIED.);
#2549=B_SPLINE_CURVE_WITH_KNOTS('',3,(#32668,#32669,#32670,#32671,#32672,
#32673,#32674,#32675,#32676,#32677,#32678,#32679,#32680,#32681,#32682,#32683,
#32684,#32685,#32686,#32687,#32688,#32689,#32690,#32691,#32692,#32693,#32694,
#32695,#32696,#32697,#32698,#32699,#32700,#32701,#32702,#32703,#32704,#32705,
#32706,#32707,#32708,#32709,#32710,#32711,#32712,#32713,#32714,#32715,#32716),
 .UNSPECIFIED.,.F.,.F.,(4,3,3,3,3,3,3,3,3,3,3,3,3,3,3,3,4),(0.,0.027427935344833,
0.0485975213880563,0.057338544085104,0.0868715743464506,0.0993492225585254,
0.10874754786483,0.133259321258805,0.148225404936155,0.157073224224447,
0.187711488807199,0.203788900709552,0.214227532674886,0.239511221647469,
0.25730153039039,0.279626282555456,0.285142803995123),.UNSPECIFIED.);
#2550=B_SPLINE_CURVE_WITH_KNOTS('',3,(#32717,#32718,#32719,#32720,#32721,
#32722,#32723,#32724,#32725,#32726,#32727,#32728,#32729,#32730,#32731,#32732,
#32733,#32734,#32735,#32736,#32737,#32738,#32739,#32740,#32741),
 .UNSPECIFIED.,.F.,.F.,(4,3,3,3,3,3,3,3,4),(-10.1357873115492,-9.92395758801633,
-8.9315618292147,-7.93916607041306,-6.94677031161143,-5.9543745528098,-4.96197879400816,
-3.96958303520653,-3.85260200436961),.UNSPECIFIED.);
#2551=B_SPLINE_CURVE_WITH_KNOTS('',3,(#33218,#33219,#33220,#33221,#33222,
#33223,#33224,#33225,#33226,#33227,#33228,#33229,#33230,#33231,#33232,#33233,
#33234,#33235,#33236,#33237,#33238,#33239),.UNSPECIFIED.,.F.,.F.,(4,3,3,
3,3,3,3,4),(7.59274844815659,7.93916607041306,8.9315618292147,9.92395758801632,
10.916353346818,11.9087491056196,12.9011448644212,13.8759337553361),
 .UNSPECIFIED.);
#2552=B_SPLINE_CURVE_WITH_KNOTS('',3,(#33240,#33241,#33242,#33243,#33244,
#33245,#33246,#33247,#33248,#33249,#33250,#33251,#33252,#33253,#33254,#33255,
#33256,#33257,#33258,#33259,#33260,#33261,#33262,#33263,#33264,#33265,#33266,
#33267,#33268,#33269,#33270,#33271,#33272,#33273,#33274,#33275,#33276,#33277,
#33278,#33279,#33280,#33281,#33282,#33283,#33284,#33285,#33286,#33287,#33288),
 .UNSPECIFIED.,.F.,.F.,(4,3,3,3,3,3,3,3,3,3,3,3,3,3,3,3,4),(0.,0.0320359961493654,
0.0578351282991586,0.0686833515155324,0.0999463544758613,0.113502099149543,
0.123023834848469,0.14759884188358,0.169881710030997,0.180117784856696,
0.205530503004595,0.220530951880297,0.231030371326071,0.247789211594336,
0.263619336128737,0.281768657448294,0.286347380332258),.UNSPECIFIED.);
#2553=B_SPLINE_CURVE_WITH_KNOTS('',3,(#33292,#33293,#33294,#33295,#33296,
#33297,#33298,#33299,#33300,#33301,#33302,#33303,#33304,#33305,#33306,#33307,
#33308,#33309,#33310,#33311,#33312,#33313,#33314,#33315,#33316,#33317,#33318,
#33319,#33320,#33321,#33322,#33323,#33324,#33325,#33326,#33327,#33328,#33329,
#33330,#33331,#33332,#33333,#33334,#33335,#33336,#33337,#33338,#33339,#33340,
#33341,#33342,#33343,#33344,#33345,#33346),.UNSPECIFIED.,.F.,.F.,(4,3,3,
3,3,3,3,3,3,3,3,3,3,3,3,3,3,3,4),(-0.378621596831434,-0.353562249903933,
-0.339726595154467,-0.324795073175994,-0.299958563910779,-0.289109739323556,
-0.25235894447449,-0.234461207277299,-0.219335840287605,-0.20082949567809,
-0.174834335133969,-0.155874235881852,-0.144961055903939,-0.109724944879178,
-0.089723852283725,-0.0773553386782937,-0.0372306048514265,-0.00401661180489575,
0.),.UNSPECIFIED.);
#2554=B_SPLINE_CURVE_WITH_KNOTS('',3,(#33347,#33348,#33349,#33350,#33351,
#33352,#33353,#33354,#33355,#33356,#33357,#33358,#33359,#33360,#33361,#33362,
#33363,#33364,#33365,#33366,#33367,#33368,#33369,#33370,#33371,#33372,#33373,
#33374,#33375,#33376,#33377,#33378,#33379,#33380,#33381,#33382,#33383,#33384,
#33385,#33386,#33387,#33388,#33389,#33390,#33391,#33392,#33393,#33394,#33395,
#33396,#33397,#33398,#33399,#33400,#33401),.UNSPECIFIED.,.F.,.F.,(4,3,3,
3,3,3,3,3,3,3,3,3,3,3,3,3,3,3,4),(-0.376940817211603,-0.35160224691684,
-0.332515709335319,-0.31822436103578,-0.288310916204436,-0.272711478712379,
-0.234501138719602,-0.216951876329547,-0.20548608487052,-0.180854828870935,
-0.153741722238776,-0.136717958714649,-0.126362699189128,-0.0955896266494597,
-0.0668165609022854,-0.0558907541314208,-0.0219997397314357,-0.00327040903045418,
0.),.UNSPECIFIED.);
#2555=B_SPLINE_CURVE_WITH_KNOTS('',3,(#33403,#33404,#33405,#33406,#33407,
#33408,#33409,#33410,#33411,#33412,#33413),.UNSPECIFIED.,.F.,.F.,(4,1,1,
1,1,1,1,1,4),(15.7079632679489,15.8518654961884,16.8494368691713,17.8470082421542,
18.8445796151372,19.8421509881201,20.839722361103,21.837293734086,21.9911485751285),
 .UNSPECIFIED.);
#2556=B_SPLINE_CURVE_WITH_KNOTS('',3,(#33414,#33415,#33416,#33417,#33418,
#33419,#33420,#33421,#33422,#33423),.UNSPECIFIED.,.F.,.F.,(4,1,1,1,1,1,
1,4),(15.7079632679489,16.3932837587428,17.3908551317257,18.3884265047086,
19.3859978776916,20.3835692506745,21.3811406236574,21.9911485751285),
 .UNSPECIFIED.);
#2557=B_SPLINE_CURVE_WITH_KNOTS('',3,(#33768,#33769,#33770,#33771,#33772,
#33773,#33774,#33775,#33776,#33777,#33778,#33779,#33780,#33781,#33782,#33783,
#33784,#33785,#33786,#33787,#33788,#33789,#33790,#33791,#33792,#33793,#33794,
#33795,#33796,#33797,#33798,#33799,#33800,#33801,#33802,#33803,#33804,#33805,
#33806,#33807,#33808,#33809,#33810,#33811,#33812,#33813,#33814,#33815,#33816,
#33817,#33818,#33819),.UNSPECIFIED.,.F.,.F.,(4,3,3,3,3,3,3,3,3,3,3,3,3,
3,3,3,3,4),(0.,0.0336989330766502,0.058737806914676,0.0734856897216009,
0.109795026944167,0.13287001176372,0.143641059388719,0.177205256270034,
0.195910789941764,0.207613330853891,0.24488927972035,0.269584354829063,
0.282495236861346,0.310139624218381,0.327566593080831,0.34255192583909,
0.372940760482297,0.376940817211641),.UNSPECIFIED.);
#2558=B_SPLINE_CURVE_WITH_KNOTS('',3,(#33820,#33821,#33822,#33823,#33824,
#33825,#33826,#33827,#33828,#33829,#33830,#33831,#33832,#33833,#33834,#33835,
#33836,#33837,#33838,#33839,#33840,#33841,#33842,#33843,#33844),
 .UNSPECIFIED.,.F.,.F.,(4,3,3,3,3,3,3,3,4),(-10.1295685708718,-9.97571372982933,
-8.9781423568464,-7.98057098386346,-6.98299961088053,-5.9854282378976,-4.98785686491466,
-3.99028549193173,-3.84638326369226),.UNSPECIFIED.);
#2559=B_SPLINE_CURVE_WITH_KNOTS('',3,(#34189,#34190,#34191,#34192,#34193,
#34194,#34195,#34196,#34197,#34198,#34199,#34200,#34201,#34202,#34203,#34204,
#34205,#34206,#34207,#34208,#34209,#34210),.UNSPECIFIED.,.F.,.F.,(4,3,3,
3,3,3,3,4),(7.59300756235155,7.98057098386346,8.9781423568464,9.97571372982933,
10.9732851028123,11.9708564757952,12.9684278487781,13.8761928695311),
 .UNSPECIFIED.);
#2560=B_SPLINE_CURVE_WITH_KNOTS('',3,(#34211,#34212,#34213,#34214,#34215,
#34216,#34217,#34218,#34219,#34220,#34221,#34222,#34223,#34224,#34225,#34226,
#34227,#34228,#34229,#34230,#34231,#34232,#34233,#34234,#34235,#34236,#34237,
#34238,#34239,#34240,#34241,#34242,#34243,#34244,#34245,#34246,#34247,#34248,
#34249,#34250,#34251,#34252,#34253,#34254,#34255,#34256,#34257,#34258,#34259,
#34260,#34261,#34262),.UNSPECIFIED.,.F.,.F.,(4,3,3,3,3,3,3,3,3,3,3,3,3,
3,3,3,3,4),(0.,0.0396836996751474,0.0598295377036724,0.0776045542344442,
0.089287041955902,0.127960856426141,0.1530367876033,0.165008599097631,0.197163594226426,
0.224449840232547,0.234157399588655,0.269452851616206,0.2876129966593,0.30541494242687,
0.333061769489462,0.34722178230466,0.375339207698859,0.378621596831421),
 .UNSPECIFIED.);
#3160=LINE('',#29859,#3792);
#3161=LINE('',#29894,#3793);
#3162=LINE('',#29921,#3794);
#3163=LINE('',#29972,#3795);
#3164=LINE('',#30020,#3796);
#3165=LINE('',#30068,#3797);
#3166=LINE('',#30119,#3798);
#3167=LINE('',#30167,#3799);
#3168=LINE('',#30215,#3800);
#3169=LINE('',#30266,#3801);
#3170=LINE('',#30317,#3802);
#3171=LINE('',#30365,#3803);
#3172=LINE('',#30416,#3804);
#3173=LINE('',#30455,#3805);
#3174=LINE('',#30477,#3806);
#3175=LINE('',#30501,#3807);
#3176=LINE('',#30526,#3808);
#3177=LINE('',#30551,#3809);
#3178=LINE('',#30575,#3810);
#3179=LINE('',#30600,#3811);
#3180=LINE('',#30624,#3812);
#3181=LINE('',#30649,#3813);
#3182=LINE('',#30673,#3814);
#3183=LINE('',#30698,#3815);
#3184=LINE('',#30723,#3816);
#3185=LINE('',#30747,#3817);
#3186=LINE('',#30764,#3818);
#3187=LINE('',#30773,#3819);
#3188=LINE('',#30790,#3820);
#3189=LINE('',#30841,#3821);
#3190=LINE('',#30892,#3822);
#3191=LINE('',#30940,#3823);
#3192=LINE('',#30991,#3824);
#3193=LINE('',#31042,#3825);
#3194=LINE('',#31090,#3826);
#3195=LINE('',#31141,#3827);
#3196=LINE('',#31192,#3828);
#3197=LINE('',#31240,#3829);
#3198=LINE('',#31291,#3830);
#3199=LINE('',#31342,#3831);
#3200=LINE('',#31390,#3832);
#3201=LINE('',#31441,#3833);
#3202=LINE('',#31492,#3834);
#3203=LINE('',#31540,#3835);
#3204=LINE('',#31591,#3836);
#3205=LINE('',#31630,#3837);
#3206=LINE('',#31654,#3838);
#3207=LINE('',#31678,#3839);
#3208=LINE('',#31703,#3840);
#3209=LINE('',#31728,#3841);
#3210=LINE('',#31752,#3842);
#3211=LINE('',#31777,#3843);
#3212=LINE('',#31802,#3844);
#3213=LINE('',#31826,#3845);
#3214=LINE('',#31851,#3846);
#3215=LINE('',#31876,#3847);
#3216=LINE('',#31900,#3848);
#3217=LINE('',#31925,#3849);
#3218=LINE('',#31950,#3850);
#3219=LINE('',#31974,#3851);
#3220=LINE('',#31999,#3852);
#3221=LINE('',#32024,#3853);
#3222=LINE('',#32048,#3854);
#3223=LINE('',#34268,#3855);
#3224=LINE('',#34270,#3856);
#3225=LINE('',#34272,#3857);
#3226=LINE('',#34273,#3858);
#3227=LINE('',#34276,#3859);
#3228=LINE('',#34278,#3860);
#3229=LINE('',#34279,#3861);
#3230=LINE('',#34282,#3862);
#3231=LINE('',#34284,#3863);
#3232=LINE('',#34285,#3864);
#3233=LINE('',#34287,#3865);
#3234=LINE('',#34288,#3866);
#3792=VECTOR('',#13521,0.2);
#3793=VECTOR('',#13524,0.2);
#3794=VECTOR('',#13529,0.2);
#3795=VECTOR('',#13532,0.2);
#3796=VECTOR('',#13535,0.2);
#3797=VECTOR('',#13538,0.2);
#3798=VECTOR('',#13541,0.2);
#3799=VECTOR('',#13544,0.2);
#3800=VECTOR('',#13547,0.2);
#3801=VECTOR('',#13550,0.2);
#3802=VECTOR('',#13553,0.2);
#3803=VECTOR('',#13556,0.2);
#3804=VECTOR('',#13559,0.2);
#3805=VECTOR('',#13564,0.205475);
#3806=VECTOR('',#13569,0.205475);
#3807=VECTOR('',#13572,0.205475);
#3808=VECTOR('',#13575,0.205475);
#3809=VECTOR('',#13578,0.205475);
#3810=VECTOR('',#13581,0.205475);
#3811=VECTOR('',#13584,0.205475);
#3812=VECTOR('',#13587,0.205475);
#3813=VECTOR('',#13590,0.205475);
#3814=VECTOR('',#13593,0.205475);
#3815=VECTOR('',#13596,0.205475);
#3816=VECTOR('',#13599,0.205475);
#3817=VECTOR('',#13602,0.205475);
#3818=VECTOR('',#13607,0.15);
#3819=VECTOR('',#13610,0.15);
#3820=VECTOR('',#13617,0.15);
#3821=VECTOR('',#13620,0.15);
#3822=VECTOR('',#13623,0.15);
#3823=VECTOR('',#13626,0.15);
#3824=VECTOR('',#13629,0.15);
#3825=VECTOR('',#13632,0.15);
#3826=VECTOR('',#13635,0.15);
#3827=VECTOR('',#13638,0.15);
#3828=VECTOR('',#13641,0.15);
#3829=VECTOR('',#13644,0.15);
#3830=VECTOR('',#13647,0.15);
#3831=VECTOR('',#13650,0.15);
#3832=VECTOR('',#13653,0.15);
#3833=VECTOR('',#13656,0.15);
#3834=VECTOR('',#13659,0.15);
#3835=VECTOR('',#13662,0.15);
#3836=VECTOR('',#13665,0.15);
#3837=VECTOR('',#13670,0.1543);
#3838=VECTOR('',#13675,0.1543);
#3839=VECTOR('',#13678,0.1543);
#3840=VECTOR('',#13681,0.1543);
#3841=VECTOR('',#13684,0.1543);
#3842=VECTOR('',#13687,0.1543);
#3843=VECTOR('',#13690,0.1543);
#3844=VECTOR('',#13693,0.1543);
#3845=VECTOR('',#13696,0.1543);
#3846=VECTOR('',#13699,0.1543);
#3847=VECTOR('',#13702,0.1543);
#3848=VECTOR('',#13705,0.1543);
#3849=VECTOR('',#13708,0.1543);
#3850=VECTOR('',#13711,0.1543);
#3851=VECTOR('',#13714,0.1543);
#3852=VECTOR('',#13717,0.1543);
#3853=VECTOR('',#13720,0.1543);
#3854=VECTOR('',#13723,0.1543);
#3855=VECTOR('',#13744,1.);
#3856=VECTOR('',#13745,1.);
#3857=VECTOR('',#13746,1.);
#3858=VECTOR('',#13747,1.);
#3859=VECTOR('',#13750,1.);
#3860=VECTOR('',#13751,1.);
#3861=VECTOR('',#13752,1.);
#3862=VECTOR('',#13755,1.);
#3863=VECTOR('',#13756,1.);
#3864=VECTOR('',#13757,1.);
#3865=VECTOR('',#13760,1.);
#3866=VECTOR('',#13761,1.);
#4688=VERTEX_POINT('',#29857);
#4689=VERTEX_POINT('',#29858);
#4690=VERTEX_POINT('',#29860);
#4691=VERTEX_POINT('',#29883);
#4692=VERTEX_POINT('',#29885);
#4693=VERTEX_POINT('',#29893);
#4694=VERTEX_POINT('',#29919);
#4695=VERTEX_POINT('',#29920);
#4696=VERTEX_POINT('',#29970);
#4697=VERTEX_POINT('',#29971);
#4698=VERTEX_POINT('',#30018);
#4699=VERTEX_POINT('',#30019);
#4700=VERTEX_POINT('',#30066);
#4701=VERTEX_POINT('',#30067);
#4702=VERTEX_POINT('',#30117);
#4703=VERTEX_POINT('',#30118);
#4704=VERTEX_POINT('',#30165);
#4705=VERTEX_POINT('',#30166);
#4706=VERTEX_POINT('',#30213);
#4707=VERTEX_POINT('',#30214);
#4708=VERTEX_POINT('',#30264);
#4709=VERTEX_POINT('',#30265);
#4710=VERTEX_POINT('',#30315);
#4711=VERTEX_POINT('',#30316);
#4712=VERTEX_POINT('',#30363);
#4713=VERTEX_POINT('',#30364);
#4714=VERTEX_POINT('',#30414);
#4715=VERTEX_POINT('',#30415);
#4716=VERTEX_POINT('',#30417);
#4717=VERTEX_POINT('',#30431);
#4718=VERTEX_POINT('',#30453);
#4719=VERTEX_POINT('',#30454);
#4720=VERTEX_POINT('',#30456);
#4721=VERTEX_POINT('',#30464);
#4722=VERTEX_POINT('',#30475);
#4723=VERTEX_POINT('',#30476);
#4724=VERTEX_POINT('',#30499);
#4725=VERTEX_POINT('',#30500);
#4726=VERTEX_POINT('',#30524);
#4727=VERTEX_POINT('',#30525);
#4728=VERTEX_POINT('',#30549);
#4729=VERTEX_POINT('',#30550);
#4730=VERTEX_POINT('',#30573);
#4731=VERTEX_POINT('',#30574);
#4732=VERTEX_POINT('',#30598);
#4733=VERTEX_POINT('',#30599);
#4734=VERTEX_POINT('',#30622);
#4735=VERTEX_POINT('',#30623);
#4736=VERTEX_POINT('',#30647);
#4737=VERTEX_POINT('',#30648);
#4738=VERTEX_POINT('',#30671);
#4739=VERTEX_POINT('',#30672);
#4740=VERTEX_POINT('',#30696);
#4741=VERTEX_POINT('',#30697);
#4742=VERTEX_POINT('',#30721);
#4743=VERTEX_POINT('',#30722);
#4744=VERTEX_POINT('',#30745);
#4745=VERTEX_POINT('',#30746);
#4746=VERTEX_POINT('',#30748);
#4747=VERTEX_POINT('',#30754);
#4748=VERTEX_POINT('',#30762);
#4749=VERTEX_POINT('',#30763);
#4750=VERTEX_POINT('',#30765);
#4751=VERTEX_POINT('',#30770);
#4752=VERTEX_POINT('',#30772);
#4753=VERTEX_POINT('',#30775);
#4754=VERTEX_POINT('',#30788);
#4755=VERTEX_POINT('',#30789);
#4756=VERTEX_POINT('',#30839);
#4757=VERTEX_POINT('',#30840);
#4758=VERTEX_POINT('',#30890);
#4759=VERTEX_POINT('',#30891);
#4760=VERTEX_POINT('',#30938);
#4761=VERTEX_POINT('',#30939);
#4762=VERTEX_POINT('',#30989);
#4763=VERTEX_POINT('',#30990);
#4764=VERTEX_POINT('',#31040);
#4765=VERTEX_POINT('',#31041);
#4766=VERTEX_POINT('',#31088);
#4767=VERTEX_POINT('',#31089);
#4768=VERTEX_POINT('',#31139);
#4769=VERTEX_POINT('',#31140);
#4770=VERTEX_POINT('',#31190);
#4771=VERTEX_POINT('',#31191);
#4772=VERTEX_POINT('',#31238);
#4773=VERTEX_POINT('',#31239);
#4774=VERTEX_POINT('',#31289);
#4775=VERTEX_POINT('',#31290);
#4776=VERTEX_POINT('',#31340);
#4777=VERTEX_POINT('',#31341);
#4778=VERTEX_POINT('',#31388);
#4779=VERTEX_POINT('',#31389);
#4780=VERTEX_POINT('',#31439);
#4781=VERTEX_POINT('',#31440);
#4782=VERTEX_POINT('',#31490);
#4783=VERTEX_POINT('',#31491);
#4784=VERTEX_POINT('',#31538);
#4785=VERTEX_POINT('',#31539);
#4786=VERTEX_POINT('',#31589);
#4787=VERTEX_POINT('',#31590);
#4788=VERTEX_POINT('',#31592);
#4789=VERTEX_POINT('',#31606);
#4790=VERTEX_POINT('',#31628);
#4791=VERTEX_POINT('',#31629);
#4792=VERTEX_POINT('',#31631);
#4793=VERTEX_POINT('',#31640);
#4794=VERTEX_POINT('',#31652);
#4795=VERTEX_POINT('',#31653);
#4796=VERTEX_POINT('',#31676);
#4797=VERTEX_POINT('',#31677);
#4798=VERTEX_POINT('',#31701);
#4799=VERTEX_POINT('',#31702);
#4800=VERTEX_POINT('',#31726);
#4801=VERTEX_POINT('',#31727);
#4802=VERTEX_POINT('',#31750);
#4803=VERTEX_POINT('',#31751);
#4804=VERTEX_POINT('',#31775);
#4805=VERTEX_POINT('',#31776);
#4806=VERTEX_POINT('',#31800);
#4807=VERTEX_POINT('',#31801);
#4808=VERTEX_POINT('',#31824);
#4809=VERTEX_POINT('',#31825);
#4810=VERTEX_POINT('',#31849);
#4811=VERTEX_POINT('',#31850);
#4812=VERTEX_POINT('',#31874);
#4813=VERTEX_POINT('',#31875);
#4814=VERTEX_POINT('',#31898);
#4815=VERTEX_POINT('',#31899);
#4816=VERTEX_POINT('',#31923);
#4817=VERTEX_POINT('',#31924);
#4818=VERTEX_POINT('',#31948);
#4819=VERTEX_POINT('',#31949);
#4820=VERTEX_POINT('',#31972);
#4821=VERTEX_POINT('',#31973);
#4822=VERTEX_POINT('',#31997);
#4823=VERTEX_POINT('',#31998);
#4824=VERTEX_POINT('',#32022);
#4825=VERTEX_POINT('',#32023);
#4826=VERTEX_POINT('',#32046);
#4827=VERTEX_POINT('',#32047);
#4828=VERTEX_POINT('',#32049);
#4829=VERTEX_POINT('',#32055);
#4830=VERTEX_POINT('',#34266);
#4831=VERTEX_POINT('',#34267);
#4832=VERTEX_POINT('',#34269);
#4833=VERTEX_POINT('',#34271);
#4834=VERTEX_POINT('',#34275);
#4835=VERTEX_POINT('',#34277);
#4836=VERTEX_POINT('',#34281);
#4837=VERTEX_POINT('',#34283);
#6095=EDGE_CURVE('',#4688,#4689,#3160,.T.);
#6096=EDGE_CURVE('',#4689,#4690,#2422,.T.);
#6097=EDGE_CURVE('',#4690,#4691,#1936,.T.);
#6098=EDGE_CURVE('',#4691,#4692,#2423,.T.);
#6099=EDGE_CURVE('',#4692,#4693,#3161,.T.);
#6100=EDGE_CURVE('',#4693,#4693,#1937,.F.);
#6101=EDGE_CURVE('',#4692,#4688,#2424,.T.);
#6102=EDGE_CURVE('',#4694,#4695,#3162,.T.);
#6103=EDGE_CURVE('',#4695,#4689,#2425,.T.);
#6104=EDGE_CURVE('',#4688,#4694,#2426,.T.);
#6105=EDGE_CURVE('',#4696,#4697,#3163,.T.);
#6106=EDGE_CURVE('',#4697,#4695,#2427,.T.);
#6107=EDGE_CURVE('',#4694,#4696,#2428,.T.);
#6108=EDGE_CURVE('',#4698,#4699,#3164,.T.);
#6109=EDGE_CURVE('',#4699,#4697,#2429,.T.);
#6110=EDGE_CURVE('',#4696,#4698,#2430,.T.);
#6111=EDGE_CURVE('',#4700,#4701,#3165,.T.);
#6112=EDGE_CURVE('',#4701,#4699,#2431,.T.);
#6113=EDGE_CURVE('',#4698,#4700,#2432,.T.);
#6114=EDGE_CURVE('',#4702,#4703,#3166,.T.);
#6115=EDGE_CURVE('',#4703,#4701,#2433,.T.);
#6116=EDGE_CURVE('',#4700,#4702,#2434,.T.);
#6117=EDGE_CURVE('',#4704,#4705,#3167,.T.);
#6118=EDGE_CURVE('',#4705,#4703,#2435,.T.);
#6119=EDGE_CURVE('',#4702,#4704,#2436,.T.);
#6120=EDGE_CURVE('',#4706,#4707,#3168,.T.);
#6121=EDGE_CURVE('',#4707,#4705,#2437,.T.);
#6122=EDGE_CURVE('',#4704,#4706,#2438,.T.);
#6123=EDGE_CURVE('',#4708,#4709,#3169,.T.);
#6124=EDGE_CURVE('',#4709,#4707,#2439,.T.);
#6125=EDGE_CURVE('',#4706,#4708,#2440,.T.);
#6126=EDGE_CURVE('',#4710,#4711,#3170,.T.);
#6127=EDGE_CURVE('',#4711,#4709,#2441,.T.);
#6128=EDGE_CURVE('',#4708,#4710,#2442,.T.);
#6129=EDGE_CURVE('',#4712,#4713,#3171,.T.);
#6130=EDGE_CURVE('',#4713,#4711,#2443,.T.);
#6131=EDGE_CURVE('',#4710,#4712,#2444,.T.);
#6132=EDGE_CURVE('',#4714,#4715,#3172,.T.);
#6133=EDGE_CURVE('',#4714,#4716,#2445,.T.);
#6134=EDGE_CURVE('',#4717,#4716,#1938,.F.);
#6135=EDGE_CURVE('',#4717,#4715,#2446,.T.);
#6136=EDGE_CURVE('',#4718,#4719,#3173,.T.);
#6137=EDGE_CURVE('',#4719,#4720,#2447,.T.);
#6138=EDGE_CURVE('',#4721,#4720,#1939,.T.);
#6139=EDGE_CURVE('',#4718,#4721,#2448,.T.);
#6140=EDGE_CURVE('',#4722,#4723,#3174,.T.);
#6141=EDGE_CURVE('',#4723,#4719,#2449,.T.);
#6142=EDGE_CURVE('',#4722,#4718,#2450,.T.);
#6143=EDGE_CURVE('',#4724,#4725,#3175,.T.);
#6144=EDGE_CURVE('',#4725,#4723,#2451,.T.);
#6145=EDGE_CURVE('',#4724,#4722,#2452,.T.);
#6146=EDGE_CURVE('',#4726,#4727,#3176,.T.);
#6147=EDGE_CURVE('',#4727,#4725,#2453,.T.);
#6148=EDGE_CURVE('',#4726,#4724,#2454,.T.);
#6149=EDGE_CURVE('',#4728,#4729,#3177,.T.);
#6150=EDGE_CURVE('',#4729,#4727,#2455,.T.);
#6151=EDGE_CURVE('',#4728,#4726,#2456,.T.);
#6152=EDGE_CURVE('',#4730,#4731,#3178,.T.);
#6153=EDGE_CURVE('',#4731,#4729,#2457,.T.);
#6154=EDGE_CURVE('',#4730,#4728,#2458,.T.);
#6155=EDGE_CURVE('',#4732,#4733,#3179,.T.);
#6156=EDGE_CURVE('',#4733,#4731,#2459,.T.);
#6157=EDGE_CURVE('',#4732,#4730,#2460,.T.);
#6158=EDGE_CURVE('',#4734,#4735,#3180,.T.);
#6159=EDGE_CURVE('',#4735,#4733,#2461,.T.);
#6160=EDGE_CURVE('',#4734,#4732,#2462,.T.);
#6161=EDGE_CURVE('',#4736,#4737,#3181,.T.);
#6162=EDGE_CURVE('',#4737,#4735,#2463,.T.);
#6163=EDGE_CURVE('',#4736,#4734,#2464,.T.);
#6164=EDGE_CURVE('',#4738,#4739,#3182,.T.);
#6165=EDGE_CURVE('',#4739,#4737,#2465,.T.);
#6166=EDGE_CURVE('',#4738,#4736,#2466,.T.);
#6167=EDGE_CURVE('',#4740,#4741,#3183,.T.);
#6168=EDGE_CURVE('',#4741,#4739,#2467,.T.);
#6169=EDGE_CURVE('',#4740,#4738,#2468,.T.);
#6170=EDGE_CURVE('',#4742,#4743,#3184,.T.);
#6171=EDGE_CURVE('',#4743,#4741,#2469,.T.);
#6172=EDGE_CURVE('',#4742,#4740,#2470,.T.);
#6173=EDGE_CURVE('',#4744,#4745,#3185,.T.);
#6174=EDGE_CURVE('',#4746,#4744,#2471,.T.);
#6175=EDGE_CURVE('',#4747,#4746,#1940,.T.);
#6176=EDGE_CURVE('',#4747,#4745,#2472,.T.);
#6177=EDGE_CURVE('',#4748,#4749,#3186,.T.);
#6178=EDGE_CURVE('',#4749,#4750,#2473,.T.);
#6179=EDGE_CURVE('',#4750,#4751,#1941,.T.);
#6180=EDGE_CURVE('',#4751,#4752,#3187,.T.);
#6181=EDGE_CURVE('',#4752,#4752,#1942,.F.);
#6182=EDGE_CURVE('',#4751,#4753,#1943,.T.);
#6183=EDGE_CURVE('',#4753,#4748,#2474,.T.);
#6184=EDGE_CURVE('',#4754,#4755,#3188,.T.);
#6185=EDGE_CURVE('',#4755,#4749,#2475,.T.);
#6186=EDGE_CURVE('',#4748,#4754,#2476,.T.);
#6187=EDGE_CURVE('',#4756,#4757,#3189,.T.);
#6188=EDGE_CURVE('',#4757,#4755,#2477,.T.);
#6189=EDGE_CURVE('',#4754,#4756,#2478,.T.);
#6190=EDGE_CURVE('',#4758,#4759,#3190,.T.);
#6191=EDGE_CURVE('',#4759,#4757,#2479,.T.);
#6192=EDGE_CURVE('',#4756,#4758,#2480,.T.);
#6193=EDGE_CURVE('',#4760,#4761,#3191,.T.);
#6194=EDGE_CURVE('',#4761,#4759,#2481,.T.);
#6195=EDGE_CURVE('',#4758,#4760,#2482,.T.);
#6196=EDGE_CURVE('',#4762,#4763,#3192,.T.);
#6197=EDGE_CURVE('',#4763,#4761,#2483,.T.);
#6198=EDGE_CURVE('',#4760,#4762,#2484,.T.);
#6199=EDGE_CURVE('',#4764,#4765,#3193,.T.);
#6200=EDGE_CURVE('',#4765,#4763,#2485,.T.);
#6201=EDGE_CURVE('',#4762,#4764,#2486,.T.);
#6202=EDGE_CURVE('',#4766,#4767,#3194,.T.);
#6203=EDGE_CURVE('',#4767,#4765,#2487,.T.);
#6204=EDGE_CURVE('',#4764,#4766,#2488,.T.);
#6205=EDGE_CURVE('',#4768,#4769,#3195,.T.);
#6206=EDGE_CURVE('',#4769,#4767,#2489,.T.);
#6207=EDGE_CURVE('',#4766,#4768,#2490,.T.);
#6208=EDGE_CURVE('',#4770,#4771,#3196,.T.);
#6209=EDGE_CURVE('',#4771,#4769,#2491,.T.);
#6210=EDGE_CURVE('',#4768,#4770,#2492,.T.);
#6211=EDGE_CURVE('',#4772,#4773,#3197,.T.);
#6212=EDGE_CURVE('',#4773,#4771,#2493,.T.);
#6213=EDGE_CURVE('',#4770,#4772,#2494,.T.);
#6214=EDGE_CURVE('',#4774,#4775,#3198,.T.);
#6215=EDGE_CURVE('',#4775,#4773,#2495,.T.);
#6216=EDGE_CURVE('',#4772,#4774,#2496,.T.);
#6217=EDGE_CURVE('',#4776,#4777,#3199,.T.);
#6218=EDGE_CURVE('',#4777,#4775,#2497,.T.);
#6219=EDGE_CURVE('',#4774,#4776,#2498,.T.);
#6220=EDGE_CURVE('',#4778,#4779,#3200,.T.);
#6221=EDGE_CURVE('',#4779,#4777,#2499,.T.);
#6222=EDGE_CURVE('',#4776,#4778,#2500,.T.);
#6223=EDGE_CURVE('',#4780,#4781,#3201,.T.);
#6224=EDGE_CURVE('',#4781,#4779,#2501,.T.);
#6225=EDGE_CURVE('',#4778,#4780,#2502,.T.);
#6226=EDGE_CURVE('',#4782,#4783,#3202,.T.);
#6227=EDGE_CURVE('',#4783,#4781,#2503,.T.);
#6228=EDGE_CURVE('',#4780,#4782,#2504,.T.);
#6229=EDGE_CURVE('',#4784,#4785,#3203,.T.);
#6230=EDGE_CURVE('',#4785,#4783,#2505,.T.);
#6231=EDGE_CURVE('',#4782,#4784,#2506,.T.);
#6232=EDGE_CURVE('',#4786,#4787,#3204,.T.);
#6233=EDGE_CURVE('',#4786,#4788,#2507,.T.);
#6234=EDGE_CURVE('',#4789,#4788,#1944,.T.);
#6235=EDGE_CURVE('',#4789,#4787,#2508,.T.);
#6236=EDGE_CURVE('',#4790,#4791,#3205,.T.);
#6237=EDGE_CURVE('',#4791,#4792,#2509,.T.);
#6238=EDGE_CURVE('',#4793,#4792,#1945,.T.);
#6239=EDGE_CURVE('',#4790,#4793,#2510,.T.);
#6240=EDGE_CURVE('',#4794,#4795,#3206,.T.);
#6241=EDGE_CURVE('',#4795,#4791,#2511,.T.);
#6242=EDGE_CURVE('',#4794,#4790,#2512,.T.);
#6243=EDGE_CURVE('',#4796,#4797,#3207,.T.);
#6244=EDGE_CURVE('',#4797,#4795,#2513,.T.);
#6245=EDGE_CURVE('',#4796,#4794,#2514,.T.);
#6246=EDGE_CURVE('',#4798,#4799,#3208,.T.);
#6247=EDGE_CURVE('',#4799,#4797,#2515,.T.);
#6248=EDGE_CURVE('',#4798,#4796,#2516,.T.);
#6249=EDGE_CURVE('',#4800,#4801,#3209,.T.);
#6250=EDGE_CURVE('',#4801,#4799,#2517,.T.);
#6251=EDGE_CURVE('',#4800,#4798,#2518,.T.);
#6252=EDGE_CURVE('',#4802,#4803,#3210,.T.);
#6253=EDGE_CURVE('',#4803,#4801,#2519,.T.);
#6254=EDGE_CURVE('',#4802,#4800,#2520,.T.);
#6255=EDGE_CURVE('',#4804,#4805,#3211,.T.);
#6256=EDGE_CURVE('',#4805,#4803,#2521,.T.);
#6257=EDGE_CURVE('',#4804,#4802,#2522,.T.);
#6258=EDGE_CURVE('',#4806,#4807,#3212,.T.);
#6259=EDGE_CURVE('',#4807,#4805,#2523,.T.);
#6260=EDGE_CURVE('',#4806,#4804,#2524,.T.);
#6261=EDGE_CURVE('',#4808,#4809,#3213,.T.);
#6262=EDGE_CURVE('',#4809,#4807,#2525,.T.);
#6263=EDGE_CURVE('',#4808,#4806,#2526,.T.);
#6264=EDGE_CURVE('',#4810,#4811,#3214,.T.);
#6265=EDGE_CURVE('',#4811,#4809,#2527,.T.);
#6266=EDGE_CURVE('',#4810,#4808,#2528,.T.);
#6267=EDGE_CURVE('',#4812,#4813,#3215,.T.);
#6268=EDGE_CURVE('',#4813,#4811,#2529,.T.);
#6269=EDGE_CURVE('',#4812,#4810,#2530,.T.);
#6270=EDGE_CURVE('',#4814,#4815,#3216,.T.);
#6271=EDGE_CURVE('',#4815,#4813,#2531,.T.);
#6272=EDGE_CURVE('',#4814,#4812,#2532,.T.);
#6273=EDGE_CURVE('',#4816,#4817,#3217,.T.);
#6274=EDGE_CURVE('',#4817,#4815,#2533,.T.);
#6275=EDGE_CURVE('',#4816,#4814,#2534,.T.);
#6276=EDGE_CURVE('',#4818,#4819,#3218,.T.);
#6277=EDGE_CURVE('',#4819,#4817,#2535,.T.);
#6278=EDGE_CURVE('',#4818,#4816,#2536,.T.);
#6279=EDGE_CURVE('',#4820,#4821,#3219,.T.);
#6280=EDGE_CURVE('',#4821,#4819,#2537,.T.);
#6281=EDGE_CURVE('',#4820,#4818,#2538,.T.);
#6282=EDGE_CURVE('',#4822,#4823,#3220,.T.);
#6283=EDGE_CURVE('',#4823,#4821,#2539,.T.);
#6284=EDGE_CURVE('',#4822,#4820,#2540,.T.);
#6285=EDGE_CURVE('',#4824,#4825,#3221,.T.);
#6286=EDGE_CURVE('',#4825,#4823,#2541,.T.);
#6287=EDGE_CURVE('',#4824,#4822,#2542,.T.);
#6288=EDGE_CURVE('',#4826,#4827,#3222,.T.);
#6289=EDGE_CURVE('',#4828,#4826,#2543,.T.);
#6290=EDGE_CURVE('',#4829,#4828,#1946,.T.);
#6291=EDGE_CURVE('',#4829,#4827,#2544,.T.);
#6292=EDGE_CURVE('',#4750,#4793,#2545,.T.);
#6293=EDGE_CURVE('',#4792,#4753,#2546,.T.);
#6294=EDGE_CURVE('',#4827,#4825,#2547,.T.);
#6295=EDGE_CURVE('',#4826,#4824,#2548,.T.);
#6296=EDGE_CURVE('',#4788,#4829,#2549,.T.);
#6297=EDGE_CURVE('',#4784,#4786,#2550,.T.);
#6298=EDGE_CURVE('',#4787,#4785,#2551,.T.);
#6299=EDGE_CURVE('',#4828,#4789,#2552,.T.);
#6300=EDGE_CURVE('',#4690,#4721,#2553,.T.);
#6301=EDGE_CURVE('',#4720,#4691,#2554,.T.);
#6302=EDGE_CURVE('',#4745,#4743,#2555,.T.);
#6303=EDGE_CURVE('',#4744,#4742,#2556,.T.);
#6304=EDGE_CURVE('',#4716,#4747,#2557,.T.);
#6305=EDGE_CURVE('',#4712,#4714,#2558,.T.);
#6306=EDGE_CURVE('',#4715,#4713,#2559,.T.);
#6307=EDGE_CURVE('',#4746,#4717,#2560,.T.);
#6308=EDGE_CURVE('',#4830,#4831,#3223,.T.);
#6309=EDGE_CURVE('',#4831,#4832,#3224,.T.);
#6310=EDGE_CURVE('',#4833,#4832,#3225,.T.);
#6311=EDGE_CURVE('',#4830,#4833,#3226,.T.);
#6312=EDGE_CURVE('',#4834,#4830,#3227,.T.);
#6313=EDGE_CURVE('',#4835,#4833,#3228,.T.);
#6314=EDGE_CURVE('',#4834,#4835,#3229,.T.);
#6315=EDGE_CURVE('',#4836,#4834,#3230,.T.);
#6316=EDGE_CURVE('',#4837,#4835,#3231,.T.);
#6317=EDGE_CURVE('',#4836,#4837,#3232,.T.);
#6318=EDGE_CURVE('',#4831,#4836,#3233,.T.);
#6319=EDGE_CURVE('',#4832,#4837,#3234,.T.);
#8651=ORIENTED_EDGE('',*,*,#6095,.T.);
#8652=ORIENTED_EDGE('',*,*,#6096,.T.);
#8653=ORIENTED_EDGE('',*,*,#6097,.T.);
#8654=ORIENTED_EDGE('',*,*,#6098,.T.);
#8655=ORIENTED_EDGE('',*,*,#6099,.T.);
#8656=ORIENTED_EDGE('',*,*,#6100,.T.);
#8657=ORIENTED_EDGE('',*,*,#6099,.F.);
#8658=ORIENTED_EDGE('',*,*,#6101,.T.);
#8659=ORIENTED_EDGE('',*,*,#6102,.T.);
#8660=ORIENTED_EDGE('',*,*,#6103,.T.);
#8661=ORIENTED_EDGE('',*,*,#6095,.F.);
#8662=ORIENTED_EDGE('',*,*,#6104,.T.);
#8663=ORIENTED_EDGE('',*,*,#6105,.T.);
#8664=ORIENTED_EDGE('',*,*,#6106,.T.);
#8665=ORIENTED_EDGE('',*,*,#6102,.F.);
#8666=ORIENTED_EDGE('',*,*,#6107,.T.);
#8667=ORIENTED_EDGE('',*,*,#6108,.T.);
#8668=ORIENTED_EDGE('',*,*,#6109,.T.);
#8669=ORIENTED_EDGE('',*,*,#6105,.F.);
#8670=ORIENTED_EDGE('',*,*,#6110,.T.);
#8671=ORIENTED_EDGE('',*,*,#6111,.T.);
#8672=ORIENTED_EDGE('',*,*,#6112,.T.);
#8673=ORIENTED_EDGE('',*,*,#6108,.F.);
#8674=ORIENTED_EDGE('',*,*,#6113,.T.);
#8675=ORIENTED_EDGE('',*,*,#6114,.T.);
#8676=ORIENTED_EDGE('',*,*,#6115,.T.);
#8677=ORIENTED_EDGE('',*,*,#6111,.F.);
#8678=ORIENTED_EDGE('',*,*,#6116,.T.);
#8679=ORIENTED_EDGE('',*,*,#6117,.T.);
#8680=ORIENTED_EDGE('',*,*,#6118,.T.);
#8681=ORIENTED_EDGE('',*,*,#6114,.F.);
#8682=ORIENTED_EDGE('',*,*,#6119,.T.);
#8683=ORIENTED_EDGE('',*,*,#6120,.T.);
#8684=ORIENTED_EDGE('',*,*,#6121,.T.);
#8685=ORIENTED_EDGE('',*,*,#6117,.F.);
#8686=ORIENTED_EDGE('',*,*,#6122,.T.);
#8687=ORIENTED_EDGE('',*,*,#6123,.T.);
#8688=ORIENTED_EDGE('',*,*,#6124,.T.);
#8689=ORIENTED_EDGE('',*,*,#6120,.F.);
#8690=ORIENTED_EDGE('',*,*,#6125,.T.);
#8691=ORIENTED_EDGE('',*,*,#6126,.T.);
#8692=ORIENTED_EDGE('',*,*,#6127,.T.);
#8693=ORIENTED_EDGE('',*,*,#6123,.F.);
#8694=ORIENTED_EDGE('',*,*,#6128,.T.);
#8695=ORIENTED_EDGE('',*,*,#6129,.T.);
#8696=ORIENTED_EDGE('',*,*,#6130,.T.);
#8697=ORIENTED_EDGE('',*,*,#6126,.F.);
#8698=ORIENTED_EDGE('',*,*,#6131,.T.);
#8699=ORIENTED_EDGE('',*,*,#6132,.F.);
#8700=ORIENTED_EDGE('',*,*,#6133,.T.);
#8701=ORIENTED_EDGE('',*,*,#6134,.F.);
#8702=ORIENTED_EDGE('',*,*,#6135,.T.);
#8703=ORIENTED_EDGE('',*,*,#6136,.T.);
#8704=ORIENTED_EDGE('',*,*,#6137,.T.);
#8705=ORIENTED_EDGE('',*,*,#6138,.F.);
#8706=ORIENTED_EDGE('',*,*,#6139,.F.);
#8707=ORIENTED_EDGE('',*,*,#6140,.T.);
#8708=ORIENTED_EDGE('',*,*,#6141,.T.);
#8709=ORIENTED_EDGE('',*,*,#6136,.F.);
#8710=ORIENTED_EDGE('',*,*,#6142,.F.);
#8711=ORIENTED_EDGE('',*,*,#6143,.T.);
#8712=ORIENTED_EDGE('',*,*,#6144,.T.);
#8713=ORIENTED_EDGE('',*,*,#6140,.F.);
#8714=ORIENTED_EDGE('',*,*,#6145,.F.);
#8715=ORIENTED_EDGE('',*,*,#6146,.T.);
#8716=ORIENTED_EDGE('',*,*,#6147,.T.);
#8717=ORIENTED_EDGE('',*,*,#6143,.F.);
#8718=ORIENTED_EDGE('',*,*,#6148,.F.);
#8719=ORIENTED_EDGE('',*,*,#6149,.T.);
#8720=ORIENTED_EDGE('',*,*,#6150,.T.);
#8721=ORIENTED_EDGE('',*,*,#6146,.F.);
#8722=ORIENTED_EDGE('',*,*,#6151,.F.);
#8723=ORIENTED_EDGE('',*,*,#6152,.T.);
#8724=ORIENTED_EDGE('',*,*,#6153,.T.);
#8725=ORIENTED_EDGE('',*,*,#6149,.F.);
#8726=ORIENTED_EDGE('',*,*,#6154,.F.);
#8727=ORIENTED_EDGE('',*,*,#6155,.T.);
#8728=ORIENTED_EDGE('',*,*,#6156,.T.);
#8729=ORIENTED_EDGE('',*,*,#6152,.F.);
#8730=ORIENTED_EDGE('',*,*,#6157,.F.);
#8731=ORIENTED_EDGE('',*,*,#6158,.T.);
#8732=ORIENTED_EDGE('',*,*,#6159,.T.);
#8733=ORIENTED_EDGE('',*,*,#6155,.F.);
#8734=ORIENTED_EDGE('',*,*,#6160,.F.);
#8735=ORIENTED_EDGE('',*,*,#6161,.T.);
#8736=ORIENTED_EDGE('',*,*,#6162,.T.);
#8737=ORIENTED_EDGE('',*,*,#6158,.F.);
#8738=ORIENTED_EDGE('',*,*,#6163,.F.);
#8739=ORIENTED_EDGE('',*,*,#6164,.T.);
#8740=ORIENTED_EDGE('',*,*,#6165,.T.);
#8741=ORIENTED_EDGE('',*,*,#6161,.F.);
#8742=ORIENTED_EDGE('',*,*,#6166,.F.);
#8743=ORIENTED_EDGE('',*,*,#6167,.T.);
#8744=ORIENTED_EDGE('',*,*,#6168,.T.);
#8745=ORIENTED_EDGE('',*,*,#6164,.F.);
#8746=ORIENTED_EDGE('',*,*,#6169,.F.);
#8747=ORIENTED_EDGE('',*,*,#6170,.T.);
#8748=ORIENTED_EDGE('',*,*,#6171,.T.);
#8749=ORIENTED_EDGE('',*,*,#6167,.F.);
#8750=ORIENTED_EDGE('',*,*,#6172,.F.);
#8751=ORIENTED_EDGE('',*,*,#6173,.F.);
#8752=ORIENTED_EDGE('',*,*,#6174,.F.);
#8753=ORIENTED_EDGE('',*,*,#6175,.F.);
#8754=ORIENTED_EDGE('',*,*,#6176,.T.);
#8755=ORIENTED_EDGE('',*,*,#6177,.T.);
#8756=ORIENTED_EDGE('',*,*,#6178,.T.);
#8757=ORIENTED_EDGE('',*,*,#6179,.T.);
#8758=ORIENTED_EDGE('',*,*,#6180,.T.);
#8759=ORIENTED_EDGE('',*,*,#6181,.T.);
#8760=ORIENTED_EDGE('',*,*,#6180,.F.);
#8761=ORIENTED_EDGE('',*,*,#6182,.T.);
#8762=ORIENTED_EDGE('',*,*,#6183,.T.);
#8763=ORIENTED_EDGE('',*,*,#6184,.T.);
#8764=ORIENTED_EDGE('',*,*,#6185,.T.);
#8765=ORIENTED_EDGE('',*,*,#6177,.F.);
#8766=ORIENTED_EDGE('',*,*,#6186,.T.);
#8767=ORIENTED_EDGE('',*,*,#6187,.T.);
#8768=ORIENTED_EDGE('',*,*,#6188,.T.);
#8769=ORIENTED_EDGE('',*,*,#6184,.F.);
#8770=ORIENTED_EDGE('',*,*,#6189,.T.);
#8771=ORIENTED_EDGE('',*,*,#6190,.T.);
#8772=ORIENTED_EDGE('',*,*,#6191,.T.);
#8773=ORIENTED_EDGE('',*,*,#6187,.F.);
#8774=ORIENTED_EDGE('',*,*,#6192,.T.);
#8775=ORIENTED_EDGE('',*,*,#6193,.T.);
#8776=ORIENTED_EDGE('',*,*,#6194,.T.);
#8777=ORIENTED_EDGE('',*,*,#6190,.F.);
#8778=ORIENTED_EDGE('',*,*,#6195,.T.);
#8779=ORIENTED_EDGE('',*,*,#6196,.T.);
#8780=ORIENTED_EDGE('',*,*,#6197,.T.);
#8781=ORIENTED_EDGE('',*,*,#6193,.F.);
#8782=ORIENTED_EDGE('',*,*,#6198,.T.);
#8783=ORIENTED_EDGE('',*,*,#6199,.T.);
#8784=ORIENTED_EDGE('',*,*,#6200,.T.);
#8785=ORIENTED_EDGE('',*,*,#6196,.F.);
#8786=ORIENTED_EDGE('',*,*,#6201,.T.);
#8787=ORIENTED_EDGE('',*,*,#6202,.T.);
#8788=ORIENTED_EDGE('',*,*,#6203,.T.);
#8789=ORIENTED_EDGE('',*,*,#6199,.F.);
#8790=ORIENTED_EDGE('',*,*,#6204,.T.);
#8791=ORIENTED_EDGE('',*,*,#6205,.T.);
#8792=ORIENTED_EDGE('',*,*,#6206,.T.);
#8793=ORIENTED_EDGE('',*,*,#6202,.F.);
#8794=ORIENTED_EDGE('',*,*,#6207,.T.);
#8795=ORIENTED_EDGE('',*,*,#6208,.T.);
#8796=ORIENTED_EDGE('',*,*,#6209,.T.);
#8797=ORIENTED_EDGE('',*,*,#6205,.F.);
#8798=ORIENTED_EDGE('',*,*,#6210,.T.);
#8799=ORIENTED_EDGE('',*,*,#6211,.T.);
#8800=ORIENTED_EDGE('',*,*,#6212,.T.);
#8801=ORIENTED_EDGE('',*,*,#6208,.F.);
#8802=ORIENTED_EDGE('',*,*,#6213,.T.);
#8803=ORIENTED_EDGE('',*,*,#6214,.T.);
#8804=ORIENTED_EDGE('',*,*,#6215,.T.);
#8805=ORIENTED_EDGE('',*,*,#6211,.F.);
#8806=ORIENTED_EDGE('',*,*,#6216,.T.);
#8807=ORIENTED_EDGE('',*,*,#6217,.T.);
#8808=ORIENTED_EDGE('',*,*,#6218,.T.);
#8809=ORIENTED_EDGE('',*,*,#6214,.F.);
#8810=ORIENTED_EDGE('',*,*,#6219,.T.);
#8811=ORIENTED_EDGE('',*,*,#6220,.T.);
#8812=ORIENTED_EDGE('',*,*,#6221,.T.);
#8813=ORIENTED_EDGE('',*,*,#6217,.F.);
#8814=ORIENTED_EDGE('',*,*,#6222,.T.);
#8815=ORIENTED_EDGE('',*,*,#6223,.T.);
#8816=ORIENTED_EDGE('',*,*,#6224,.T.);
#8817=ORIENTED_EDGE('',*,*,#6220,.F.);
#8818=ORIENTED_EDGE('',*,*,#6225,.T.);
#8819=ORIENTED_EDGE('',*,*,#6226,.T.);
#8820=ORIENTED_EDGE('',*,*,#6227,.T.);
#8821=ORIENTED_EDGE('',*,*,#6223,.F.);
#8822=ORIENTED_EDGE('',*,*,#6228,.T.);
#8823=ORIENTED_EDGE('',*,*,#6229,.T.);
#8824=ORIENTED_EDGE('',*,*,#6230,.T.);
#8825=ORIENTED_EDGE('',*,*,#6226,.F.);
#8826=ORIENTED_EDGE('',*,*,#6231,.T.);
#8827=ORIENTED_EDGE('',*,*,#6232,.F.);
#8828=ORIENTED_EDGE('',*,*,#6233,.T.);
#8829=ORIENTED_EDGE('',*,*,#6234,.F.);
#8830=ORIENTED_EDGE('',*,*,#6235,.T.);
#8831=ORIENTED_EDGE('',*,*,#6236,.T.);
#8832=ORIENTED_EDGE('',*,*,#6237,.T.);
#8833=ORIENTED_EDGE('',*,*,#6238,.F.);
#8834=ORIENTED_EDGE('',*,*,#6239,.F.);
#8835=ORIENTED_EDGE('',*,*,#6240,.T.);
#8836=ORIENTED_EDGE('',*,*,#6241,.T.);
#8837=ORIENTED_EDGE('',*,*,#6236,.F.);
#8838=ORIENTED_EDGE('',*,*,#6242,.F.);
#8839=ORIENTED_EDGE('',*,*,#6243,.T.);
#8840=ORIENTED_EDGE('',*,*,#6244,.T.);
#8841=ORIENTED_EDGE('',*,*,#6240,.F.);
#8842=ORIENTED_EDGE('',*,*,#6245,.F.);
#8843=ORIENTED_EDGE('',*,*,#6246,.T.);
#8844=ORIENTED_EDGE('',*,*,#6247,.T.);
#8845=ORIENTED_EDGE('',*,*,#6243,.F.);
#8846=ORIENTED_EDGE('',*,*,#6248,.F.);
#8847=ORIENTED_EDGE('',*,*,#6249,.T.);
#8848=ORIENTED_EDGE('',*,*,#6250,.T.);
#8849=ORIENTED_EDGE('',*,*,#6246,.F.);
#8850=ORIENTED_EDGE('',*,*,#6251,.F.);
#8851=ORIENTED_EDGE('',*,*,#6252,.T.);
#8852=ORIENTED_EDGE('',*,*,#6253,.T.);
#8853=ORIENTED_EDGE('',*,*,#6249,.F.);
#8854=ORIENTED_EDGE('',*,*,#6254,.F.);
#8855=ORIENTED_EDGE('',*,*,#6255,.T.);
#8856=ORIENTED_EDGE('',*,*,#6256,.T.);
#8857=ORIENTED_EDGE('',*,*,#6252,.F.);
#8858=ORIENTED_EDGE('',*,*,#6257,.F.);
#8859=ORIENTED_EDGE('',*,*,#6258,.T.);
#8860=ORIENTED_EDGE('',*,*,#6259,.T.);
#8861=ORIENTED_EDGE('',*,*,#6255,.F.);
#8862=ORIENTED_EDGE('',*,*,#6260,.F.);
#8863=ORIENTED_EDGE('',*,*,#6261,.T.);
#8864=ORIENTED_EDGE('',*,*,#6262,.T.);
#8865=ORIENTED_EDGE('',*,*,#6258,.F.);
#8866=ORIENTED_EDGE('',*,*,#6263,.F.);
#8867=ORIENTED_EDGE('',*,*,#6264,.T.);
#8868=ORIENTED_EDGE('',*,*,#6265,.T.);
#8869=ORIENTED_EDGE('',*,*,#6261,.F.);
#8870=ORIENTED_EDGE('',*,*,#6266,.F.);
#8871=ORIENTED_EDGE('',*,*,#6267,.T.);
#8872=ORIENTED_EDGE('',*,*,#6268,.T.);
#8873=ORIENTED_EDGE('',*,*,#6264,.F.);
#8874=ORIENTED_EDGE('',*,*,#6269,.F.);
#8875=ORIENTED_EDGE('',*,*,#6270,.T.);
#8876=ORIENTED_EDGE('',*,*,#6271,.T.);
#8877=ORIENTED_EDGE('',*,*,#6267,.F.);
#8878=ORIENTED_EDGE('',*,*,#6272,.F.);
#8879=ORIENTED_EDGE('',*,*,#6273,.T.);
#8880=ORIENTED_EDGE('',*,*,#6274,.T.);
#8881=ORIENTED_EDGE('',*,*,#6270,.F.);
#8882=ORIENTED_EDGE('',*,*,#6275,.F.);
#8883=ORIENTED_EDGE('',*,*,#6276,.T.);
#8884=ORIENTED_EDGE('',*,*,#6277,.T.);
#8885=ORIENTED_EDGE('',*,*,#6273,.F.);
#8886=ORIENTED_EDGE('',*,*,#6278,.F.);
#8887=ORIENTED_EDGE('',*,*,#6279,.T.);
#8888=ORIENTED_EDGE('',*,*,#6280,.T.);
#8889=ORIENTED_EDGE('',*,*,#6276,.F.);
#8890=ORIENTED_EDGE('',*,*,#6281,.F.);
#8891=ORIENTED_EDGE('',*,*,#6282,.T.);
#8892=ORIENTED_EDGE('',*,*,#6283,.T.);
#8893=ORIENTED_EDGE('',*,*,#6279,.F.);
#8894=ORIENTED_EDGE('',*,*,#6284,.F.);
#8895=ORIENTED_EDGE('',*,*,#6285,.T.);
#8896=ORIENTED_EDGE('',*,*,#6286,.T.);
#8897=ORIENTED_EDGE('',*,*,#6282,.F.);
#8898=ORIENTED_EDGE('',*,*,#6287,.F.);
#8899=ORIENTED_EDGE('',*,*,#6288,.F.);
#8900=ORIENTED_EDGE('',*,*,#6289,.F.);
#8901=ORIENTED_EDGE('',*,*,#6290,.F.);
#8902=ORIENTED_EDGE('',*,*,#6291,.T.);
#8903=ORIENTED_EDGE('',*,*,#6179,.F.);
#8904=ORIENTED_EDGE('',*,*,#6292,.T.);
#8905=ORIENTED_EDGE('',*,*,#6238,.T.);
#8906=ORIENTED_EDGE('',*,*,#6293,.T.);
#8907=ORIENTED_EDGE('',*,*,#6182,.F.);
#8908=ORIENTED_EDGE('',*,*,#6288,.T.);
#8909=ORIENTED_EDGE('',*,*,#6294,.T.);
#8910=ORIENTED_EDGE('',*,*,#6285,.F.);
#8911=ORIENTED_EDGE('',*,*,#6295,.F.);
#8912=ORIENTED_EDGE('',*,*,#6293,.F.);
#8913=ORIENTED_EDGE('',*,*,#6237,.F.);
#8914=ORIENTED_EDGE('',*,*,#6241,.F.);
#8915=ORIENTED_EDGE('',*,*,#6244,.F.);
#8916=ORIENTED_EDGE('',*,*,#6247,.F.);
#8917=ORIENTED_EDGE('',*,*,#6250,.F.);
#8918=ORIENTED_EDGE('',*,*,#6253,.F.);
#8919=ORIENTED_EDGE('',*,*,#6256,.F.);
#8920=ORIENTED_EDGE('',*,*,#6259,.F.);
#8921=ORIENTED_EDGE('',*,*,#6262,.F.);
#8922=ORIENTED_EDGE('',*,*,#6265,.F.);
#8923=ORIENTED_EDGE('',*,*,#6268,.F.);
#8924=ORIENTED_EDGE('',*,*,#6271,.F.);
#8925=ORIENTED_EDGE('',*,*,#6274,.F.);
#8926=ORIENTED_EDGE('',*,*,#6277,.F.);
#8927=ORIENTED_EDGE('',*,*,#6280,.F.);
#8928=ORIENTED_EDGE('',*,*,#6283,.F.);
#8929=ORIENTED_EDGE('',*,*,#6286,.F.);
#8930=ORIENTED_EDGE('',*,*,#6294,.F.);
#8931=ORIENTED_EDGE('',*,*,#6291,.F.);
#8932=ORIENTED_EDGE('',*,*,#6296,.F.);
#8933=ORIENTED_EDGE('',*,*,#6233,.F.);
#8934=ORIENTED_EDGE('',*,*,#6297,.F.);
#8935=ORIENTED_EDGE('',*,*,#6231,.F.);
#8936=ORIENTED_EDGE('',*,*,#6228,.F.);
#8937=ORIENTED_EDGE('',*,*,#6225,.F.);
#8938=ORIENTED_EDGE('',*,*,#6222,.F.);
#8939=ORIENTED_EDGE('',*,*,#6219,.F.);
#8940=ORIENTED_EDGE('',*,*,#6216,.F.);
#8941=ORIENTED_EDGE('',*,*,#6213,.F.);
#8942=ORIENTED_EDGE('',*,*,#6210,.F.);
#8943=ORIENTED_EDGE('',*,*,#6207,.F.);
#8944=ORIENTED_EDGE('',*,*,#6204,.F.);
#8945=ORIENTED_EDGE('',*,*,#6201,.F.);
#8946=ORIENTED_EDGE('',*,*,#6198,.F.);
#8947=ORIENTED_EDGE('',*,*,#6195,.F.);
#8948=ORIENTED_EDGE('',*,*,#6192,.F.);
#8949=ORIENTED_EDGE('',*,*,#6189,.F.);
#8950=ORIENTED_EDGE('',*,*,#6186,.F.);
#8951=ORIENTED_EDGE('',*,*,#6183,.F.);
#8952=ORIENTED_EDGE('',*,*,#6292,.F.);
#8953=ORIENTED_EDGE('',*,*,#6178,.F.);
#8954=ORIENTED_EDGE('',*,*,#6185,.F.);
#8955=ORIENTED_EDGE('',*,*,#6188,.F.);
#8956=ORIENTED_EDGE('',*,*,#6191,.F.);
#8957=ORIENTED_EDGE('',*,*,#6194,.F.);
#8958=ORIENTED_EDGE('',*,*,#6197,.F.);
#8959=ORIENTED_EDGE('',*,*,#6200,.F.);
#8960=ORIENTED_EDGE('',*,*,#6203,.F.);
#8961=ORIENTED_EDGE('',*,*,#6206,.F.);
#8962=ORIENTED_EDGE('',*,*,#6209,.F.);
#8963=ORIENTED_EDGE('',*,*,#6212,.F.);
#8964=ORIENTED_EDGE('',*,*,#6215,.F.);
#8965=ORIENTED_EDGE('',*,*,#6218,.F.);
#8966=ORIENTED_EDGE('',*,*,#6221,.F.);
#8967=ORIENTED_EDGE('',*,*,#6224,.F.);
#8968=ORIENTED_EDGE('',*,*,#6227,.F.);
#8969=ORIENTED_EDGE('',*,*,#6230,.F.);
#8970=ORIENTED_EDGE('',*,*,#6298,.F.);
#8971=ORIENTED_EDGE('',*,*,#6235,.F.);
#8972=ORIENTED_EDGE('',*,*,#6299,.F.);
#8973=ORIENTED_EDGE('',*,*,#6289,.T.);
#8974=ORIENTED_EDGE('',*,*,#6295,.T.);
#8975=ORIENTED_EDGE('',*,*,#6287,.T.);
#8976=ORIENTED_EDGE('',*,*,#6284,.T.);
#8977=ORIENTED_EDGE('',*,*,#6281,.T.);
#8978=ORIENTED_EDGE('',*,*,#6278,.T.);
#8979=ORIENTED_EDGE('',*,*,#6275,.T.);
#8980=ORIENTED_EDGE('',*,*,#6272,.T.);
#8981=ORIENTED_EDGE('',*,*,#6269,.T.);
#8982=ORIENTED_EDGE('',*,*,#6266,.T.);
#8983=ORIENTED_EDGE('',*,*,#6263,.T.);
#8984=ORIENTED_EDGE('',*,*,#6260,.T.);
#8985=ORIENTED_EDGE('',*,*,#6257,.T.);
#8986=ORIENTED_EDGE('',*,*,#6254,.T.);
#8987=ORIENTED_EDGE('',*,*,#6251,.T.);
#8988=ORIENTED_EDGE('',*,*,#6248,.T.);
#8989=ORIENTED_EDGE('',*,*,#6245,.T.);
#8990=ORIENTED_EDGE('',*,*,#6242,.T.);
#8991=ORIENTED_EDGE('',*,*,#6239,.T.);
#8992=ORIENTED_EDGE('',*,*,#6232,.T.);
#8993=ORIENTED_EDGE('',*,*,#6298,.T.);
#8994=ORIENTED_EDGE('',*,*,#6229,.F.);
#8995=ORIENTED_EDGE('',*,*,#6297,.T.);
#8996=ORIENTED_EDGE('',*,*,#6181,.F.);
#8997=ORIENTED_EDGE('',*,*,#6097,.F.);
#8998=ORIENTED_EDGE('',*,*,#6300,.T.);
#8999=ORIENTED_EDGE('',*,*,#6138,.T.);
#9000=ORIENTED_EDGE('',*,*,#6301,.T.);
#9001=ORIENTED_EDGE('',*,*,#6173,.T.);
#9002=ORIENTED_EDGE('',*,*,#6302,.T.);
#9003=ORIENTED_EDGE('',*,*,#6170,.F.);
#9004=ORIENTED_EDGE('',*,*,#6303,.F.);
#9005=ORIENTED_EDGE('',*,*,#6301,.F.);
#9006=ORIENTED_EDGE('',*,*,#6137,.F.);
#9007=ORIENTED_EDGE('',*,*,#6141,.F.);
#9008=ORIENTED_EDGE('',*,*,#6144,.F.);
#9009=ORIENTED_EDGE('',*,*,#6147,.F.);
#9010=ORIENTED_EDGE('',*,*,#6150,.F.);
#9011=ORIENTED_EDGE('',*,*,#6153,.F.);
#9012=ORIENTED_EDGE('',*,*,#6156,.F.);
#9013=ORIENTED_EDGE('',*,*,#6159,.F.);
#9014=ORIENTED_EDGE('',*,*,#6162,.F.);
#9015=ORIENTED_EDGE('',*,*,#6165,.F.);
#9016=ORIENTED_EDGE('',*,*,#6168,.F.);
#9017=ORIENTED_EDGE('',*,*,#6171,.F.);
#9018=ORIENTED_EDGE('',*,*,#6302,.F.);
#9019=ORIENTED_EDGE('',*,*,#6176,.F.);
#9020=ORIENTED_EDGE('',*,*,#6304,.F.);
#9021=ORIENTED_EDGE('',*,*,#6133,.F.);
#9022=ORIENTED_EDGE('',*,*,#6305,.F.);
#9023=ORIENTED_EDGE('',*,*,#6131,.F.);
#9024=ORIENTED_EDGE('',*,*,#6128,.F.);
#9025=ORIENTED_EDGE('',*,*,#6125,.F.);
#9026=ORIENTED_EDGE('',*,*,#6122,.F.);
#9027=ORIENTED_EDGE('',*,*,#6119,.F.);
#9028=ORIENTED_EDGE('',*,*,#6116,.F.);
#9029=ORIENTED_EDGE('',*,*,#6113,.F.);
#9030=ORIENTED_EDGE('',*,*,#6110,.F.);
#9031=ORIENTED_EDGE('',*,*,#6107,.F.);
#9032=ORIENTED_EDGE('',*,*,#6104,.F.);
#9033=ORIENTED_EDGE('',*,*,#6101,.F.);
#9034=ORIENTED_EDGE('',*,*,#6098,.F.);
#9035=ORIENTED_EDGE('',*,*,#6300,.F.);
#9036=ORIENTED_EDGE('',*,*,#6096,.F.);
#9037=ORIENTED_EDGE('',*,*,#6103,.F.);
#9038=ORIENTED_EDGE('',*,*,#6106,.F.);
#9039=ORIENTED_EDGE('',*,*,#6109,.F.);
#9040=ORIENTED_EDGE('',*,*,#6112,.F.);
#9041=ORIENTED_EDGE('',*,*,#6115,.F.);
#9042=ORIENTED_EDGE('',*,*,#6118,.F.);
#9043=ORIENTED_EDGE('',*,*,#6121,.F.);
#9044=ORIENTED_EDGE('',*,*,#6124,.F.);
#9045=ORIENTED_EDGE('',*,*,#6127,.F.);
#9046=ORIENTED_EDGE('',*,*,#6130,.F.);
#9047=ORIENTED_EDGE('',*,*,#6306,.F.);
#9048=ORIENTED_EDGE('',*,*,#6135,.F.);
#9049=ORIENTED_EDGE('',*,*,#6307,.F.);
#9050=ORIENTED_EDGE('',*,*,#6174,.T.);
#9051=ORIENTED_EDGE('',*,*,#6303,.T.);
#9052=ORIENTED_EDGE('',*,*,#6172,.T.);
#9053=ORIENTED_EDGE('',*,*,#6169,.T.);
#9054=ORIENTED_EDGE('',*,*,#6166,.T.);
#9055=ORIENTED_EDGE('',*,*,#6163,.T.);
#9056=ORIENTED_EDGE('',*,*,#6160,.T.);
#9057=ORIENTED_EDGE('',*,*,#6157,.T.);
#9058=ORIENTED_EDGE('',*,*,#6154,.T.);
#9059=ORIENTED_EDGE('',*,*,#6151,.T.);
#9060=ORIENTED_EDGE('',*,*,#6148,.T.);
#9061=ORIENTED_EDGE('',*,*,#6145,.T.);
#9062=ORIENTED_EDGE('',*,*,#6142,.T.);
#9063=ORIENTED_EDGE('',*,*,#6139,.T.);
#9064=ORIENTED_EDGE('',*,*,#6132,.T.);
#9065=ORIENTED_EDGE('',*,*,#6306,.T.);
#9066=ORIENTED_EDGE('',*,*,#6129,.F.);
#9067=ORIENTED_EDGE('',*,*,#6305,.T.);
#9068=ORIENTED_EDGE('',*,*,#6100,.F.);
#9069=ORIENTED_EDGE('',*,*,#6308,.T.);
#9070=ORIENTED_EDGE('',*,*,#6309,.T.);
#9071=ORIENTED_EDGE('',*,*,#6310,.F.);
#9072=ORIENTED_EDGE('',*,*,#6311,.F.);
#9073=ORIENTED_EDGE('',*,*,#6312,.T.);
#9074=ORIENTED_EDGE('',*,*,#6311,.T.);
#9075=ORIENTED_EDGE('',*,*,#6313,.F.);
#9076=ORIENTED_EDGE('',*,*,#6314,.F.);
#9077=ORIENTED_EDGE('',*,*,#6315,.T.);
#9078=ORIENTED_EDGE('',*,*,#6314,.T.);
#9079=ORIENTED_EDGE('',*,*,#6316,.F.);
#9080=ORIENTED_EDGE('',*,*,#6317,.F.);
#9081=ORIENTED_EDGE('',*,*,#6318,.T.);
#9082=ORIENTED_EDGE('',*,*,#6317,.T.);
#9083=ORIENTED_EDGE('',*,*,#6319,.F.);
#9084=ORIENTED_EDGE('',*,*,#6309,.F.);
#9085=ORIENTED_EDGE('',*,*,#6319,.T.);
#9086=ORIENTED_EDGE('',*,*,#6316,.T.);
#9087=ORIENTED_EDGE('',*,*,#6313,.T.);
#9088=ORIENTED_EDGE('',*,*,#6310,.T.);
#9089=ORIENTED_EDGE('',*,*,#6299,.T.);
#9090=ORIENTED_EDGE('',*,*,#6234,.T.);
#9091=ORIENTED_EDGE('',*,*,#6296,.T.);
#9092=ORIENTED_EDGE('',*,*,#6290,.T.);
#9093=ORIENTED_EDGE('',*,*,#6318,.F.);
#9094=ORIENTED_EDGE('',*,*,#6308,.F.);
#9095=ORIENTED_EDGE('',*,*,#6312,.F.);
#9096=ORIENTED_EDGE('',*,*,#6315,.F.);
#9097=ORIENTED_EDGE('',*,*,#6307,.T.);
#9098=ORIENTED_EDGE('',*,*,#6134,.T.);
#9099=ORIENTED_EDGE('',*,*,#6304,.T.);
#9100=ORIENTED_EDGE('',*,*,#6175,.T.);
#10414=CYLINDRICAL_SURFACE('',#11897,0.1666);
#10415=CYLINDRICAL_SURFACE('',#11900,0.1666);
#10416=CYLINDRICAL_SURFACE('',#11901,0.1666);
#10417=CYLINDRICAL_SURFACE('',#11902,0.1666);
#10418=CYLINDRICAL_SURFACE('',#11903,0.1666);
#10419=CYLINDRICAL_SURFACE('',#11904,0.1666);
#10420=CYLINDRICAL_SURFACE('',#11905,0.1666);
#10421=CYLINDRICAL_SURFACE('',#11906,0.1666);
#10422=CYLINDRICAL_SURFACE('',#11907,0.1666);
#10423=CYLINDRICAL_SURFACE('',#11908,0.1666);
#10424=CYLINDRICAL_SURFACE('',#11909,0.1666);
#10425=CYLINDRICAL_SURFACE('',#11910,0.1666);
#10426=CYLINDRICAL_SURFACE('',#11912,0.205475);
#10427=CYLINDRICAL_SURFACE('',#11914,0.205475);
#10428=CYLINDRICAL_SURFACE('',#11915,0.205475);
#10429=CYLINDRICAL_SURFACE('',#11916,0.205475);
#10430=CYLINDRICAL_SURFACE('',#11917,0.205475);
#10431=CYLINDRICAL_SURFACE('',#11918,0.205475);
#10432=CYLINDRICAL_SURFACE('',#11919,0.205475);
#10433=CYLINDRICAL_SURFACE('',#11920,0.205475);
#10434=CYLINDRICAL_SURFACE('',#11921,0.205475);
#10435=CYLINDRICAL_SURFACE('',#11922,0.205475);
#10436=CYLINDRICAL_SURFACE('',#11923,0.205475);
#10437=CYLINDRICAL_SURFACE('',#11924,0.205475);
#10438=CYLINDRICAL_SURFACE('',#11925,0.205475);
#10439=CYLINDRICAL_SURFACE('',#11927,0.12645);
#10440=CYLINDRICAL_SURFACE('',#11931,0.12645);
#10441=CYLINDRICAL_SURFACE('',#11932,0.12645);
#10442=CYLINDRICAL_SURFACE('',#11933,0.12645);
#10443=CYLINDRICAL_SURFACE('',#11934,0.12645);
#10444=CYLINDRICAL_SURFACE('',#11935,0.12645);
#10445=CYLINDRICAL_SURFACE('',#11936,0.12645);
#10446=CYLINDRICAL_SURFACE('',#11937,0.12645);
#10447=CYLINDRICAL_SURFACE('',#11938,0.12645);
#10448=CYLINDRICAL_SURFACE('',#11939,0.12645);
#10449=CYLINDRICAL_SURFACE('',#11940,0.12645);
#10450=CYLINDRICAL_SURFACE('',#11941,0.12645);
#10451=CYLINDRICAL_SURFACE('',#11942,0.12645);
#10452=CYLINDRICAL_SURFACE('',#11943,0.12645);
#10453=CYLINDRICAL_SURFACE('',#11944,0.12645);
#10454=CYLINDRICAL_SURFACE('',#11945,0.12645);
#10455=CYLINDRICAL_SURFACE('',#11946,0.12645);
#10456=CYLINDRICAL_SURFACE('',#11947,0.12645);
#10457=CYLINDRICAL_SURFACE('',#11949,0.1543);
#10458=CYLINDRICAL_SURFACE('',#11951,0.1543);
#10459=CYLINDRICAL_SURFACE('',#11952,0.1543);
#10460=CYLINDRICAL_SURFACE('',#11953,0.1543);
#10461=CYLINDRICAL_SURFACE('',#11954,0.1543);
#10462=CYLINDRICAL_SURFACE('',#11955,0.1543);
#10463=CYLINDRICAL_SURFACE('',#11956,0.1543);
#10464=CYLINDRICAL_SURFACE('',#11957,0.1543);
#10465=CYLINDRICAL_SURFACE('',#11958,0.1543);
#10466=CYLINDRICAL_SURFACE('',#11959,0.1543);
#10467=CYLINDRICAL_SURFACE('',#11960,0.1543);
#10468=CYLINDRICAL_SURFACE('',#11961,0.1543);
#10469=CYLINDRICAL_SURFACE('',#11962,0.1543);
#10470=CYLINDRICAL_SURFACE('',#11963,0.1543);
#10471=CYLINDRICAL_SURFACE('',#11964,0.1543);
#10472=CYLINDRICAL_SURFACE('',#11965,0.1543);
#10473=CYLINDRICAL_SURFACE('',#11966,0.1543);
#10474=CYLINDRICAL_SURFACE('',#11967,0.1543);
#10475=CYLINDRICAL_SURFACE('',#11970,0.1543);
#10476=CYLINDRICAL_SURFACE('',#11971,0.12645);
#10477=CYLINDRICAL_SURFACE('',#11974,0.205475);
#10478=CYLINDRICAL_SURFACE('',#11975,0.1666);
#10945=ADVANCED_FACE('',(#820),#10414,.F.);
#10946=ADVANCED_FACE('',(#821),#10415,.F.);
#10947=ADVANCED_FACE('',(#822),#10416,.F.);
#10948=ADVANCED_FACE('',(#823),#10417,.F.);
#10949=ADVANCED_FACE('',(#824),#10418,.F.);
#10950=ADVANCED_FACE('',(#825),#10419,.F.);
#10951=ADVANCED_FACE('',(#826),#10420,.F.);
#10952=ADVANCED_FACE('',(#827),#10421,.F.);
#10953=ADVANCED_FACE('',(#828),#10422,.F.);
#10954=ADVANCED_FACE('',(#829),#10423,.F.);
#10955=ADVANCED_FACE('',(#830),#10424,.F.);
#10956=ADVANCED_FACE('',(#831),#10425,.F.);
#10957=ADVANCED_FACE('',(#832),#10426,.F.);
#10958=ADVANCED_FACE('',(#833),#10427,.F.);
#10959=ADVANCED_FACE('',(#834),#10428,.F.);
#10960=ADVANCED_FACE('',(#835),#10429,.F.);
#10961=ADVANCED_FACE('',(#836),#10430,.F.);
#10962=ADVANCED_FACE('',(#837),#10431,.F.);
#10963=ADVANCED_FACE('',(#838),#10432,.F.);
#10964=ADVANCED_FACE('',(#839),#10433,.F.);
#10965=ADVANCED_FACE('',(#840),#10434,.F.);
#10966=ADVANCED_FACE('',(#841),#10435,.F.);
#10967=ADVANCED_FACE('',(#842),#10436,.F.);
#10968=ADVANCED_FACE('',(#843),#10437,.F.);
#10969=ADVANCED_FACE('',(#844),#10438,.F.);
#10970=ADVANCED_FACE('',(#845),#10439,.F.);
#10971=ADVANCED_FACE('',(#846),#10440,.F.);
#10972=ADVANCED_FACE('',(#847),#10441,.F.);
#10973=ADVANCED_FACE('',(#848),#10442,.F.);
#10974=ADVANCED_FACE('',(#849),#10443,.F.);
#10975=ADVANCED_FACE('',(#850),#10444,.F.);
#10976=ADVANCED_FACE('',(#851),#10445,.F.);
#10977=ADVANCED_FACE('',(#852),#10446,.F.);
#10978=ADVANCED_FACE('',(#853),#10447,.F.);
#10979=ADVANCED_FACE('',(#854),#10448,.F.);
#10980=ADVANCED_FACE('',(#855),#10449,.F.);
#10981=ADVANCED_FACE('',(#856),#10450,.F.);
#10982=ADVANCED_FACE('',(#857),#10451,.F.);
#10983=ADVANCED_FACE('',(#858),#10452,.F.);
#10984=ADVANCED_FACE('',(#859),#10453,.F.);
#10985=ADVANCED_FACE('',(#860),#10454,.F.);
#10986=ADVANCED_FACE('',(#861),#10455,.F.);
#10987=ADVANCED_FACE('',(#862),#10456,.F.);
#10988=ADVANCED_FACE('',(#863),#10457,.F.);
#10989=ADVANCED_FACE('',(#864),#10458,.F.);
#10990=ADVANCED_FACE('',(#865),#10459,.F.);
#10991=ADVANCED_FACE('',(#866),#10460,.F.);
#10992=ADVANCED_FACE('',(#867),#10461,.F.);
#10993=ADVANCED_FACE('',(#868),#10462,.F.);
#10994=ADVANCED_FACE('',(#869),#10463,.F.);
#10995=ADVANCED_FACE('',(#870),#10464,.F.);
#10996=ADVANCED_FACE('',(#871),#10465,.F.);
#10997=ADVANCED_FACE('',(#872),#10466,.F.);
#10998=ADVANCED_FACE('',(#873),#10467,.F.);
#10999=ADVANCED_FACE('',(#874),#10468,.F.);
#11000=ADVANCED_FACE('',(#875),#10469,.F.);
#11001=ADVANCED_FACE('',(#876),#10470,.F.);
#11002=ADVANCED_FACE('',(#877),#10471,.F.);
#11003=ADVANCED_FACE('',(#878),#10472,.F.);
#11004=ADVANCED_FACE('',(#879),#10473,.F.);
#11005=ADVANCED_FACE('',(#880),#10474,.F.);
#11006=ADVANCED_FACE('',(#881),#413,.T.);
#11007=ADVANCED_FACE('',(#882),#10475,.F.);
#11008=ADVANCED_FACE('',(#883),#243,.F.);
#11009=ADVANCED_FACE('',(#884),#244,.F.);
#11010=ADVANCED_FACE('',(#885),#10476,.F.);
#11011=ADVANCED_FACE('',(#886),#414,.F.);
#11012=ADVANCED_FACE('',(#887),#415,.F.);
#11013=ADVANCED_FACE('',(#888),#10477,.F.);
#11014=ADVANCED_FACE('',(#889),#245,.F.);
#11015=ADVANCED_FACE('',(#890),#246,.F.);
#11016=ADVANCED_FACE('',(#891),#10478,.F.);
#11017=ADVANCED_FACE('',(#892),#416,.F.);
#11018=ADVANCED_FACE('',(#893),#417,.T.);
#11019=ADVANCED_FACE('',(#894),#418,.T.);
#11020=ADVANCED_FACE('',(#895),#419,.T.);
#11021=ADVANCED_FACE('',(#896),#420,.T.);
#11022=ADVANCED_FACE('',(#897,#315),#421,.T.);
#11023=ADVANCED_FACE('',(#898,#316),#422,.F.);
#11238=CLOSED_SHELL('',(#10945,#10946,#10947,#10948,#10949,#10950,#10951,
#10952,#10953,#10954,#10955,#10956,#10957,#10958,#10959,#10960,#10961,#10962,
#10963,#10964,#10965,#10966,#10967,#10968,#10969,#10970,#10971,#10972,#10973,
#10974,#10975,#10976,#10977,#10978,#10979,#10980,#10981,#10982,#10983,#10984,
#10985,#10986,#10987,#10988,#10989,#10990,#10991,#10992,#10993,#10994,#10995,
#10996,#10997,#10998,#10999,#11000,#11001,#11002,#11003,#11004,#11005,#11006,
#11007,#11008,#11009,#11010,#11011,#11012,#11013,#11014,#11015,#11016,#11017,
#11018,#11019,#11020,#11021,#11022,#11023));
#11896=AXIS2_PLACEMENT_3D('',#29855,#13517,#13518);
#11897=AXIS2_PLACEMENT_3D('',#29856,#13519,#13520);
#11898=AXIS2_PLACEMENT_3D('',#29884,#13522,#13523);
#11899=AXIS2_PLACEMENT_3D('',#29895,#13525,#13526);
#11900=AXIS2_PLACEMENT_3D('',#29918,#13527,#13528);
#11901=AXIS2_PLACEMENT_3D('',#29969,#13530,#13531);
#11902=AXIS2_PLACEMENT_3D('',#30017,#13533,#13534);
#11903=AXIS2_PLACEMENT_3D('',#30065,#13536,#13537);
#11904=AXIS2_PLACEMENT_3D('',#30116,#13539,#13540);
#11905=AXIS2_PLACEMENT_3D('',#30164,#13542,#13543);
#11906=AXIS2_PLACEMENT_3D('',#30212,#13545,#13546);
#11907=AXIS2_PLACEMENT_3D('',#30263,#13548,#13549);
#11908=AXIS2_PLACEMENT_3D('',#30314,#13551,#13552);
#11909=AXIS2_PLACEMENT_3D('',#30362,#13554,#13555);
#11910=AXIS2_PLACEMENT_3D('',#30413,#13557,#13558);
#11911=AXIS2_PLACEMENT_3D('',#30432,#13560,#13561);
#11912=AXIS2_PLACEMENT_3D('',#30452,#13562,#13563);
#11913=AXIS2_PLACEMENT_3D('',#30465,#13565,#13566);
#11914=AXIS2_PLACEMENT_3D('',#30474,#13567,#13568);
#11915=AXIS2_PLACEMENT_3D('',#30498,#13570,#13571);
#11916=AXIS2_PLACEMENT_3D('',#30523,#13573,#13574);
#11917=AXIS2_PLACEMENT_3D('',#30548,#13576,#13577);
#11918=AXIS2_PLACEMENT_3D('',#30572,#13579,#13580);
#11919=AXIS2_PLACEMENT_3D('',#30597,#13582,#13583);
#11920=AXIS2_PLACEMENT_3D('',#30621,#13585,#13586);
#11921=AXIS2_PLACEMENT_3D('',#30646,#13588,#13589);
#11922=AXIS2_PLACEMENT_3D('',#30670,#13591,#13592);
#11923=AXIS2_PLACEMENT_3D('',#30695,#13594,#13595);
#11924=AXIS2_PLACEMENT_3D('',#30720,#13597,#13598);
#11925=AXIS2_PLACEMENT_3D('',#30744,#13600,#13601);
#11926=AXIS2_PLACEMENT_3D('',#30755,#13603,#13604);
#11927=AXIS2_PLACEMENT_3D('',#30761,#13605,#13606);
#11928=AXIS2_PLACEMENT_3D('',#30771,#13608,#13609);
#11929=AXIS2_PLACEMENT_3D('',#30774,#13611,#13612);
#11930=AXIS2_PLACEMENT_3D('',#30776,#13613,#13614);
#11931=AXIS2_PLACEMENT_3D('',#30787,#13615,#13616);
#11932=AXIS2_PLACEMENT_3D('',#30838,#13618,#13619);
#11933=AXIS2_PLACEMENT_3D('',#30889,#13621,#13622);
#11934=AXIS2_PLACEMENT_3D('',#30937,#13624,#13625);
#11935=AXIS2_PLACEMENT_3D('',#30988,#13627,#13628);
#11936=AXIS2_PLACEMENT_3D('',#31039,#13630,#13631);
#11937=AXIS2_PLACEMENT_3D('',#31087,#13633,#13634);
#11938=AXIS2_PLACEMENT_3D('',#31138,#13636,#13637);
#11939=AXIS2_PLACEMENT_3D('',#31189,#13639,#13640);
#11940=AXIS2_PLACEMENT_3D('',#31237,#13642,#13643);
#11941=AXIS2_PLACEMENT_3D('',#31288,#13645,#13646);
#11942=AXIS2_PLACEMENT_3D('',#31339,#13648,#13649);
#11943=AXIS2_PLACEMENT_3D('',#31387,#13651,#13652);
#11944=AXIS2_PLACEMENT_3D('',#31438,#13654,#13655);
#11945=AXIS2_PLACEMENT_3D('',#31489,#13657,#13658);
#11946=AXIS2_PLACEMENT_3D('',#31537,#13660,#13661);
#11947=AXIS2_PLACEMENT_3D('',#31588,#13663,#13664);
#11948=AXIS2_PLACEMENT_3D('',#31607,#13666,#13667);
#11949=AXIS2_PLACEMENT_3D('',#31627,#13668,#13669);
#11950=AXIS2_PLACEMENT_3D('',#31641,#13671,#13672);
#11951=AXIS2_PLACEMENT_3D('',#31651,#13673,#13674);
#11952=AXIS2_PLACEMENT_3D('',#31675,#13676,#13677);
#11953=AXIS2_PLACEMENT_3D('',#31700,#13679,#13680);
#11954=AXIS2_PLACEMENT_3D('',#31725,#13682,#13683);
#11955=AXIS2_PLACEMENT_3D('',#31749,#13685,#13686);
#11956=AXIS2_PLACEMENT_3D('',#31774,#13688,#13689);
#11957=AXIS2_PLACEMENT_3D('',#31799,#13691,#13692);
#11958=AXIS2_PLACEMENT_3D('',#31823,#13694,#13695);
#11959=AXIS2_PLACEMENT_3D('',#31848,#13697,#13698);
#11960=AXIS2_PLACEMENT_3D('',#31873,#13700,#13701);
#11961=AXIS2_PLACEMENT_3D('',#31897,#13703,#13704);
#11962=AXIS2_PLACEMENT_3D('',#31922,#13706,#13707);
#11963=AXIS2_PLACEMENT_3D('',#31947,#13709,#13710);
#11964=AXIS2_PLACEMENT_3D('',#31971,#13712,#13713);
#11965=AXIS2_PLACEMENT_3D('',#31996,#13715,#13716);
#11966=AXIS2_PLACEMENT_3D('',#32021,#13718,#13719);
#11967=AXIS2_PLACEMENT_3D('',#32045,#13721,#13722);
#11968=AXIS2_PLACEMENT_3D('',#32056,#13724,#13725);
#11969=AXIS2_PLACEMENT_3D('',#32062,#13726,#13727);
#11970=AXIS2_PLACEMENT_3D('',#32170,#13728,#13729);
#11971=AXIS2_PLACEMENT_3D('',#33289,#13730,#13731);
#11972=AXIS2_PLACEMENT_3D('',#33290,#13732,#13733);
#11973=AXIS2_PLACEMENT_3D('',#33291,#13734,#13735);
#11974=AXIS2_PLACEMENT_3D('',#33402,#13736,#13737);
#11975=AXIS2_PLACEMENT_3D('',#34263,#13738,#13739);
#11976=AXIS2_PLACEMENT_3D('',#34264,#13740,#13741);
#11977=AXIS2_PLACEMENT_3D('',#34265,#13742,#13743);
#11978=AXIS2_PLACEMENT_3D('',#34274,#13748,#13749);
#11979=AXIS2_PLACEMENT_3D('',#34280,#13753,#13754);
#11980=AXIS2_PLACEMENT_3D('',#34286,#13758,#13759);
#11981=AXIS2_PLACEMENT_3D('',#34289,#13762,#13763);
#11982=AXIS2_PLACEMENT_3D('',#34290,#13764,#13765);
#13517=DIRECTION('axis',(0.,0.,1.));
#13518=DIRECTION('refdir',(1.,0.,0.));
#13519=DIRECTION('center_axis',(0.,0.,1.));
#13520=DIRECTION('ref_axis',(-1.,0.,0.));
#13521=DIRECTION('',(0.,0.,1.));
#13522=DIRECTION('center_axis',(0.,0.,-1.));
#13523=DIRECTION('ref_axis',(-1.,0.,0.));
#13524=DIRECTION('',(0.,0.,1.));
#13525=DIRECTION('center_axis',(0.,0.,-1.));
#13526=DIRECTION('ref_axis',(-1.,0.,0.));
#13527=DIRECTION('center_axis',(0.,0.,1.));
#13528=DIRECTION('ref_axis',(-1.,0.,0.));
#13529=DIRECTION('',(0.,0.,1.));
#13530=DIRECTION('center_axis',(0.,0.,1.));
#13531=DIRECTION('ref_axis',(-1.,0.,0.));
#13532=DIRECTION('',(0.,0.,1.));
#13533=DIRECTION('center_axis',(0.,0.,1.));
#13534=DIRECTION('ref_axis',(-1.,0.,0.));
#13535=DIRECTION('',(0.,0.,1.));
#13536=DIRECTION('center_axis',(0.,0.,1.));
#13537=DIRECTION('ref_axis',(-1.,0.,0.));
#13538=DIRECTION('',(0.,0.,1.));
#13539=DIRECTION('center_axis',(0.,0.,1.));
#13540=DIRECTION('ref_axis',(-1.,0.,0.));
#13541=DIRECTION('',(0.,0.,1.));
#13542=DIRECTION('center_axis',(0.,0.,1.));
#13543=DIRECTION('ref_axis',(-1.,0.,0.));
#13544=DIRECTION('',(0.,0.,1.));
#13545=DIRECTION('center_axis',(0.,0.,1.));
#13546=DIRECTION('ref_axis',(-1.,0.,0.));
#13547=DIRECTION('',(0.,0.,1.));
#13548=DIRECTION('center_axis',(0.,0.,1.));
#13549=DIRECTION('ref_axis',(-1.,0.,0.));
#13550=DIRECTION('',(0.,0.,1.));
#13551=DIRECTION('center_axis',(0.,0.,1.));
#13552=DIRECTION('ref_axis',(-1.,0.,0.));
#13553=DIRECTION('',(0.,0.,1.));
#13554=DIRECTION('center_axis',(0.,0.,1.));
#13555=DIRECTION('ref_axis',(-1.,0.,0.));
#13556=DIRECTION('',(0.,0.,1.));
#13557=DIRECTION('center_axis',(0.,0.,1.));
#13558=DIRECTION('ref_axis',(-0.938434237953747,-0.345457929473576,0.));
#13559=DIRECTION('',(0.,0.,1.));
#13560=DIRECTION('center_axis',(0.,0.,-1.));
#13561=DIRECTION('ref_axis',(-1.,0.,0.));
#13562=DIRECTION('center_axis',(0.,0.,1.));
#13563=DIRECTION('ref_axis',(-0.450135889590755,0.892960066801612,0.));
#13564=DIRECTION('',(-1.22464679914735E-16,-7.02543712147503E-30,1.));
#13565=DIRECTION('center_axis',(0.,0.,-1.));
#13566=DIRECTION('ref_axis',(-1.,-5.72445829159016E-14,0.));
#13567=DIRECTION('center_axis',(0.,0.,1.));
#13568=DIRECTION('ref_axis',(-1.,-5.72445829159016E-14,0.));
#13569=DIRECTION('',(-1.22464679914735E-16,-7.02543712147503E-30,1.));
#13570=DIRECTION('center_axis',(0.,0.,1.));
#13571=DIRECTION('ref_axis',(-1.,-5.72445829159016E-14,0.));
#13572=DIRECTION('',(-1.22464679914735E-16,-7.02543712147503E-30,1.));
#13573=DIRECTION('center_axis',(0.,0.,1.));
#13574=DIRECTION('ref_axis',(-1.,-5.72445829159016E-14,0.));
#13575=DIRECTION('',(-1.22464679914735E-16,-7.02543712147503E-30,1.));
#13576=DIRECTION('center_axis',(0.,0.,1.));
#13577=DIRECTION('ref_axis',(-1.,-5.72445829159016E-14,0.));
#13578=DIRECTION('',(-1.22464679914735E-16,-7.02543712147503E-30,1.));
#13579=DIRECTION('center_axis',(0.,0.,1.));
#13580=DIRECTION('ref_axis',(-1.,-5.72445829159016E-14,0.));
#13581=DIRECTION('',(-1.22464679914735E-16,-7.02543712147503E-30,1.));
#13582=DIRECTION('center_axis',(0.,0.,1.));
#13583=DIRECTION('ref_axis',(-1.,-5.72445829159016E-14,0.));
#13584=DIRECTION('',(-1.22464679914735E-16,-7.02543712147503E-30,1.));
#13585=DIRECTION('center_axis',(0.,0.,1.));
#13586=DIRECTION('ref_axis',(-1.,-5.72445829159016E-14,0.));
#13587=DIRECTION('',(-1.22464679914735E-16,-7.02543712147503E-30,1.));
#13588=DIRECTION('center_axis',(0.,0.,1.));
#13589=DIRECTION('ref_axis',(-1.,-5.72445829159016E-14,0.));
#13590=DIRECTION('',(-1.22464679914735E-16,-7.02543712147503E-30,1.));
#13591=DIRECTION('center_axis',(0.,0.,1.));
#13592=DIRECTION('ref_axis',(-1.,-5.72445829159016E-14,0.));
#13593=DIRECTION('',(-1.22464679914735E-16,-7.02543712147503E-30,1.));
#13594=DIRECTION('center_axis',(0.,0.,1.));
#13595=DIRECTION('ref_axis',(-1.,-5.72445829159016E-14,0.));
#13596=DIRECTION('',(-1.22464679914735E-16,-7.02543712147503E-30,1.));
#13597=DIRECTION('center_axis',(0.,0.,1.));
#13598=DIRECTION('ref_axis',(-1.,-5.72445829159016E-14,0.));
#13599=DIRECTION('',(-1.22464679914735E-16,-7.02543712147503E-30,1.));
#13600=DIRECTION('center_axis',(0.,0.,1.));
#13601=DIRECTION('ref_axis',(0.609351642559645,-0.79290010449606,0.));
#13602=DIRECTION('',(-1.22464679914735E-16,-7.02543712147503E-30,1.));
#13603=DIRECTION('center_axis',(0.,0.,1.));
#13604=DIRECTION('ref_axis',(-1.,-5.72445829159016E-14,0.));
#13605=DIRECTION('center_axis',(0.,0.,-1.));
#13606=DIRECTION('ref_axis',(1.,0.,0.));
#13607=DIRECTION('',(0.,0.,-1.));
#13608=DIRECTION('center_axis',(0.,0.,1.));
#13609=DIRECTION('ref_axis',(1.,0.,0.));
#13610=DIRECTION('',(0.,0.,-1.));
#13611=DIRECTION('center_axis',(0.,0.,1.));
#13612=DIRECTION('ref_axis',(1.,0.,0.));
#13613=DIRECTION('center_axis',(0.,0.,1.));
#13614=DIRECTION('ref_axis',(1.,0.,0.));
#13615=DIRECTION('center_axis',(0.,0.,-1.));
#13616=DIRECTION('ref_axis',(1.,0.,0.));
#13617=DIRECTION('',(0.,0.,-1.));
#13618=DIRECTION('center_axis',(0.,0.,-1.));
#13619=DIRECTION('ref_axis',(1.,0.,0.));
#13620=DIRECTION('',(0.,0.,-1.));
#13621=DIRECTION('center_axis',(0.,0.,-1.));
#13622=DIRECTION('ref_axis',(1.,0.,0.));
#13623=DIRECTION('',(0.,0.,-1.));
#13624=DIRECTION('center_axis',(0.,0.,-1.));
#13625=DIRECTION('ref_axis',(1.,0.,0.));
#13626=DIRECTION('',(0.,0.,-1.));
#13627=DIRECTION('center_axis',(0.,0.,-1.));
#13628=DIRECTION('ref_axis',(1.,0.,0.));
#13629=DIRECTION('',(0.,0.,-1.));
#13630=DIRECTION('center_axis',(0.,0.,-1.));
#13631=DIRECTION('ref_axis',(1.,0.,0.));
#13632=DIRECTION('',(0.,0.,-1.));
#13633=DIRECTION('center_axis',(0.,0.,-1.));
#13634=DIRECTION('ref_axis',(1.,0.,0.));
#13635=DIRECTION('',(0.,0.,-1.));
#13636=DIRECTION('center_axis',(0.,0.,-1.));
#13637=DIRECTION('ref_axis',(1.,0.,0.));
#13638=DIRECTION('',(0.,0.,-1.));
#13639=DIRECTION('center_axis',(0.,0.,-1.));
#13640=DIRECTION('ref_axis',(1.,0.,0.));
#13641=DIRECTION('',(0.,0.,-1.));
#13642=DIRECTION('center_axis',(0.,0.,-1.));
#13643=DIRECTION('ref_axis',(1.,0.,0.));
#13644=DIRECTION('',(0.,0.,-1.));
#13645=DIRECTION('center_axis',(0.,0.,-1.));
#13646=DIRECTION('ref_axis',(1.,0.,0.));
#13647=DIRECTION('',(0.,0.,-1.));
#13648=DIRECTION('center_axis',(0.,0.,-1.));
#13649=DIRECTION('ref_axis',(1.,0.,0.));
#13650=DIRECTION('',(0.,0.,-1.));
#13651=DIRECTION('center_axis',(0.,0.,-1.));
#13652=DIRECTION('ref_axis',(1.,0.,0.));
#13653=DIRECTION('',(0.,0.,-1.));
#13654=DIRECTION('center_axis',(0.,0.,-1.));
#13655=DIRECTION('ref_axis',(1.,0.,0.));
#13656=DIRECTION('',(0.,0.,-1.));
#13657=DIRECTION('center_axis',(0.,0.,-1.));
#13658=DIRECTION('ref_axis',(1.,0.,0.));
#13659=DIRECTION('',(0.,0.,-1.));
#13660=DIRECTION('center_axis',(0.,0.,-1.));
#13661=DIRECTION('ref_axis',(1.,0.,0.));
#13662=DIRECTION('',(0.,0.,-1.));
#13663=DIRECTION('center_axis',(0.,0.,-1.));
#13664=DIRECTION('ref_axis',(0.937376106323228,-0.348318870138132,0.));
#13665=DIRECTION('',(0.,0.,-1.));
#13666=DIRECTION('center_axis',(0.,0.,-1.));
#13667=DIRECTION('ref_axis',(1.,0.,0.));
#13668=DIRECTION('center_axis',(0.,0.,-1.));
#13669=DIRECTION('ref_axis',(1.,-9.27379496885572E-14,0.));
#13670=DIRECTION('',(1.22464679914735E-16,-1.13721209223846E-29,-1.));
#13671=DIRECTION('center_axis',(0.,0.,1.));
#13672=DIRECTION('ref_axis',(1.,-9.27379496885572E-14,0.));
#13673=DIRECTION('center_axis',(0.,0.,-1.));
#13674=DIRECTION('ref_axis',(1.,-9.27379496885572E-14,0.));
#13675=DIRECTION('',(1.22464679914735E-16,-1.13721209223846E-29,-1.));
#13676=DIRECTION('center_axis',(0.,0.,-1.));
#13677=DIRECTION('ref_axis',(1.,-9.27379496885572E-14,0.));
#13678=DIRECTION('',(1.22464679914735E-16,-1.13721209223846E-29,-1.));
#13679=DIRECTION('center_axis',(0.,0.,-1.));
#13680=DIRECTION('ref_axis',(1.,-9.27379496885572E-14,0.));
#13681=DIRECTION('',(1.22464679914735E-16,-1.13721209223846E-29,-1.));
#13682=DIRECTION('center_axis',(0.,0.,-1.));
#13683=DIRECTION('ref_axis',(1.,-9.27379496885572E-14,0.));
#13684=DIRECTION('',(1.22464679914735E-16,-1.13721209223846E-29,-1.));
#13685=DIRECTION('center_axis',(0.,0.,-1.));
#13686=DIRECTION('ref_axis',(1.,-9.27379496885572E-14,0.));
#13687=DIRECTION('',(1.22464679914735E-16,-1.13721209223846E-29,-1.));
#13688=DIRECTION('center_axis',(0.,0.,-1.));
#13689=DIRECTION('ref_axis',(1.,-9.27379496885572E-14,0.));
#13690=DIRECTION('',(1.22464679914735E-16,-1.13721209223846E-29,-1.));
#13691=DIRECTION('center_axis',(0.,0.,-1.));
#13692=DIRECTION('ref_axis',(1.,-9.27379496885572E-14,0.));
#13693=DIRECTION('',(1.22464679914735E-16,-1.13721209223846E-29,-1.));
#13694=DIRECTION('center_axis',(0.,0.,-1.));
#13695=DIRECTION('ref_axis',(1.,-9.27379496885572E-14,0.));
#13696=DIRECTION('',(1.22464679914735E-16,-1.13721209223846E-29,-1.));
#13697=DIRECTION('center_axis',(0.,0.,-1.));
#13698=DIRECTION('ref_axis',(1.,-9.27379496885572E-14,0.));
#13699=DIRECTION('',(1.22464679914735E-16,-1.13721209223846E-29,-1.));
#13700=DIRECTION('center_axis',(0.,0.,-1.));
#13701=DIRECTION('ref_axis',(1.,-9.27379496885572E-14,0.));
#13702=DIRECTION('',(1.22464679914735E-16,-1.13721209223846E-29,-1.));
#13703=DIRECTION('center_axis',(0.,0.,-1.));
#13704=DIRECTION('ref_axis',(1.,-9.27379496885572E-14,0.));
#13705=DIRECTION('',(1.22464679914735E-16,-1.13721209223846E-29,-1.));
#13706=DIRECTION('center_axis',(0.,0.,-1.));
#13707=DIRECTION('ref_axis',(1.,-9.27379496885572E-14,0.));
#13708=DIRECTION('',(1.22464679914735E-16,-1.13721209223846E-29,-1.));
#13709=DIRECTION('center_axis',(0.,0.,-1.));
#13710=DIRECTION('ref_axis',(1.,-9.27379496885572E-14,0.));
#13711=DIRECTION('',(1.22464679914735E-16,-1.13721209223846E-29,-1.));
#13712=DIRECTION('center_axis',(0.,0.,-1.));
#13713=DIRECTION('ref_axis',(1.,-9.27379496885572E-14,0.));
#13714=DIRECTION('',(1.22464679914735E-16,-1.13721209223846E-29,-1.));
#13715=DIRECTION('center_axis',(0.,0.,-1.));
#13716=DIRECTION('ref_axis',(1.,-9.27379496885572E-14,0.));
#13717=DIRECTION('',(1.22464679914735E-16,-1.13721209223846E-29,-1.));
#13718=DIRECTION('center_axis',(0.,0.,-1.));
#13719=DIRECTION('ref_axis',(1.,-9.27379496885572E-14,0.));
#13720=DIRECTION('',(1.22464679914735E-16,-1.13721209223846E-29,-1.));
#13721=DIRECTION('center_axis',(0.,0.,-1.));
#13722=DIRECTION('ref_axis',(-0.609161390867883,-0.793046278520936,0.));
#13723=DIRECTION('',(1.22464679914735E-16,-1.13721209223846E-29,-1.));
#13724=DIRECTION('center_axis',(0.,0.,-1.));
#13725=DIRECTION('ref_axis',(1.,-9.27379496885572E-14,0.));
#13726=DIRECTION('center_axis',(0.,0.,1.));
#13727=DIRECTION('ref_axis',(1.,0.,0.));
#13728=DIRECTION('center_axis',(0.,0.,-1.));
#13729=DIRECTION('ref_axis',(1.,-9.27379496885572E-14,0.));
#13730=DIRECTION('center_axis',(0.,0.,-1.));
#13731=DIRECTION('ref_axis',(1.,0.,0.));
#13732=DIRECTION('center_axis',(0.,0.,-1.));
#13733=DIRECTION('ref_axis',(1.,0.,0.));
#13734=DIRECTION('center_axis',(0.,0.,1.));
#13735=DIRECTION('ref_axis',(1.,0.,0.));
#13736=DIRECTION('center_axis',(0.,0.,1.));
#13737=DIRECTION('ref_axis',(-1.,-5.72445829159016E-14,0.));
#13738=DIRECTION('center_axis',(0.,0.,1.));
#13739=DIRECTION('ref_axis',(-1.,0.,0.));
#13740=DIRECTION('center_axis',(0.,0.,1.));
#13741=DIRECTION('ref_axis',(-1.,0.,0.));
#13742=DIRECTION('center_axis',(0.,1.,0.));
#13743=DIRECTION('ref_axis',(-1.,0.,0.));
#13744=DIRECTION('',(-1.,0.,0.));
#13745=DIRECTION('',(0.,0.,1.));
#13746=DIRECTION('',(-1.,0.,0.));
#13747=DIRECTION('',(0.,0.,1.));
#13748=DIRECTION('center_axis',(1.,0.,0.));
#13749=DIRECTION('ref_axis',(0.,1.,0.));
#13750=DIRECTION('',(0.,1.,0.));
#13751=DIRECTION('',(0.,1.,0.));
#13752=DIRECTION('',(0.,0.,1.));
#13753=DIRECTION('center_axis',(0.,-1.,0.));
#13754=DIRECTION('ref_axis',(1.,0.,0.));
#13755=DIRECTION('',(1.,0.,0.));
#13756=DIRECTION('',(1.,0.,0.));
#13757=DIRECTION('',(0.,0.,1.));
#13758=DIRECTION('center_axis',(-1.,0.,0.));
#13759=DIRECTION('ref_axis',(0.,-1.,0.));
#13760=DIRECTION('',(0.,-1.,0.));
#13761=DIRECTION('',(0.,-1.,0.));
#13762=DIRECTION('center_axis',(0.,0.,1.));
#13763=DIRECTION('ref_axis',(1.,0.,0.));
#13764=DIRECTION('center_axis',(0.,0.,1.));
#13765=DIRECTION('ref_axis',(1.,0.,0.));
#29855=CARTESIAN_POINT('',(0.,0.,0.));
#29856=CARTESIAN_POINT('Origin',(0.,0.,1.3));
#29857=CARTESIAN_POINT('',(0.166752921449725,-0.000121400228749406,1.61285196366098));
#29858=CARTESIAN_POINT('',(0.166796959880497,9.66735530056473E-5,1.63214803633902));
#29859=CARTESIAN_POINT('',(0.1666,2.04026156737949E-17,1.3));
#29860=CARTESIAN_POINT('',(0.163512932725146,-0.0319230454628286,1.7));
#29861=CARTESIAN_POINT('Ctrl Pts',(0.166796959880497,9.66735530056473E-5,
1.63214803633902));
#29862=CARTESIAN_POINT('Ctrl Pts',(0.166837734552074,0.00590520031683778,
1.63253777944574));
#29863=CARTESIAN_POINT('Ctrl Pts',(0.166560755157907,0.0117098399368759,
1.63292752255246));
#29864=CARTESIAN_POINT('Ctrl Pts',(0.165953190799148,0.0174796970799782,
1.63331726565918));
#29865=CARTESIAN_POINT('Ctrl Pts',(0.160178154195734,0.0723234938194388,
1.63702186201144));
#29866=CARTESIAN_POINT('Ctrl Pts',(0.124534989745148,0.12402471730472,1.64072645836371));
#29867=CARTESIAN_POINT('Ctrl Pts',(0.0753220427557469,0.148912116862319,
1.64443105471598));
#29868=CARTESIAN_POINT('Ctrl Pts',(0.0261090957663466,0.173799516419917,
1.64813565106825));
#29869=CARTESIAN_POINT('Ctrl Pts',(-0.0366736337618685,0.171873092049834,
1.65184024742052));
#29870=CARTESIAN_POINT('Ctrl Pts',(-0.0842665124811252,0.144033445936741,
1.65554484377278));
#29871=CARTESIAN_POINT('Ctrl Pts',(-0.131859391200383,0.116193799823647,
1.65924944012505));
#29872=CARTESIAN_POINT('Ctrl Pts',(-0.164262419110682,0.0624409319675427,
1.66295403647732));
#29873=CARTESIAN_POINT('Ctrl Pts',(-0.16669782361829,0.00733866012848643,
1.66665863282959));
#29874=CARTESIAN_POINT('Ctrl Pts',(-0.169133228125899,-0.0477636117105698,
1.67036322918185));
#29875=CARTESIAN_POINT('Ctrl Pts',(-0.141601009230818,-0.104215287532578,
1.67406782553412));
#29876=CARTESIAN_POINT('Ctrl Pts',(-0.0965988342506402,-0.136109501609562,
1.67777242188639));
#29877=CARTESIAN_POINT('Ctrl Pts',(-0.0515966592704642,-0.168003715686544,
1.68147701823866));
#29878=CARTESIAN_POINT('Ctrl Pts',(0.0108754717948065,-0.175340468018505,
1.68518161459093));
#29879=CARTESIAN_POINT('Ctrl Pts',(0.0619990767693629,-0.154913285529167,
1.6888862109432));
#29880=CARTESIAN_POINT('Ctrl Pts',(0.11312268174392,-0.134486103039829,
1.69259080729546));
#29881=CARTESIAN_POINT('Ctrl Pts',(0.152897760627763,-0.0862949857291919,
1.69629540364773));
#29882=CARTESIAN_POINT('Ctrl Pts',(0.163512932725146,-0.0319230454628286,
1.7));
#29883=CARTESIAN_POINT('',(0.0052623718904234,0.166820541544646,1.7));
#29884=CARTESIAN_POINT('Origin',(0.,0.,1.7));
#29885=CARTESIAN_POINT('',(0.166340825374871,-6.57396331519428E-5,1.68285196366098));
#29886=CARTESIAN_POINT('Ctrl Pts',(0.00526237188778958,0.16682061735739,
1.7));
#29887=CARTESIAN_POINT('Ctrl Pts',(0.059315846276127,0.165049198896683,
1.69636770818144));
#29888=CARTESIAN_POINT('Ctrl Pts',(0.112514618214038,0.134574177622605,
1.69273541636289));
#29889=CARTESIAN_POINT('Ctrl Pts',(0.141280425894631,0.0887797885328044,
1.68910312454433));
#29890=CARTESIAN_POINT('Ctrl Pts',(0.157782375695069,0.0625091300380853,
1.68701940424988));
#29891=CARTESIAN_POINT('Ctrl Pts',(0.166243631438541,0.0311969895334432,
1.68493568395543));
#29892=CARTESIAN_POINT('Ctrl Pts',(0.166340825374871,-6.57396331519428E-5,
1.68285196366098));
#29893=CARTESIAN_POINT('',(0.1666,-2.04026156737949E-17,1.8));
#29894=CARTESIAN_POINT('',(0.1666,2.04026156737949E-17,1.3));
#29895=CARTESIAN_POINT('Origin',(0.,0.,1.8));
#29896=CARTESIAN_POINT('Ctrl Pts',(0.166340825374871,-6.57396331519428E-5,
1.68285196366098));
#29897=CARTESIAN_POINT('Ctrl Pts',(0.166416430207622,-0.024384267097259,
1.68123108760316));
#29898=CARTESIAN_POINT('Ctrl Pts',(0.161431015607884,-0.0486728962000426,
1.67961021154535));
#29899=CARTESIAN_POINT('Ctrl Pts',(0.151232376946182,-0.070535415398117,
1.67798933548753));
#29900=CARTESIAN_POINT('Ctrl Pts',(0.12792285898394,-0.120503337672002,
1.67428473913526));
#29901=CARTESIAN_POINT('Ctrl Pts',(0.0773807749454364,-0.157797874435697,
1.67058014278299));
#29902=CARTESIAN_POINT('Ctrl Pts',(0.0227482513872868,-0.165320125260105,
1.66687554643073));
#29903=CARTESIAN_POINT('Ctrl Pts',(-0.0318842721708627,-0.172842376084512,
1.66317095007846));
#29904=CARTESIAN_POINT('Ctrl Pts',(-0.0906072352486578,-0.150592340969633,
1.65946635372619));
#29905=CARTESIAN_POINT('Ctrl Pts',(-0.126551605667113,-0.108768963100728,
1.65576175737392));
#29906=CARTESIAN_POINT('Ctrl Pts',(-0.162495976085569,-0.0669455852318239,
1.65205716102165));
#29907=CARTESIAN_POINT('Ctrl Pts',(-0.175661753844685,-0.00554886460889432,
1.64835256466938));
#29908=CARTESIAN_POINT('Ctrl Pts',(-0.160020484350268,0.0473310422055452,
1.64464796831712));
#29909=CARTESIAN_POINT('Ctrl Pts',(-0.144379214855851,0.100210949019985,
1.64094337196485));
#29910=CARTESIAN_POINT('Ctrl Pts',(-0.0999308981078997,0.144574042025934,
1.63723877561258));
#29911=CARTESIAN_POINT('Ctrl Pts',(-0.0470191573240233,0.160112912591645,
1.63353417926031));
#29912=CARTESIAN_POINT('Ctrl Pts',(0.00589258345985309,0.175651783157355,
1.62982958290805));
#29913=CARTESIAN_POINT('Ctrl Pts',(0.067267748279655,0.162366431282826,
1.62612498655578));
#29914=CARTESIAN_POINT('Ctrl Pts',(0.109018480103692,0.126339265236092,
1.62242039020351));
#29915=CARTESIAN_POINT('Ctrl Pts',(0.144963809686008,0.0953216446845623,
1.61923091468933));
#29916=CARTESIAN_POINT('Ctrl Pts',(0.166362794628908,0.0474469630018487,
1.61604143917516));
#29917=CARTESIAN_POINT('Ctrl Pts',(0.166752921449725,-0.000121400228749406,
1.61285196366098));
#29918=CARTESIAN_POINT('Origin',(0.,0.,1.3));
#29919=CARTESIAN_POINT('',(0.166721717270512,0.00013247748987999,1.54285196366098));
#29920=CARTESIAN_POINT('',(0.166368100504911,8.32215516180224E-5,1.56214803633902));
#29921=CARTESIAN_POINT('',(0.1666,2.04026156737949E-17,1.3));
#29922=CARTESIAN_POINT('Ctrl Pts',(0.166368100504911,8.32215516180223E-5,
1.56214803633902));
#29923=CARTESIAN_POINT('Ctrl Pts',(0.166469575983711,0.0225191704554514,
1.56364353466546));
#29924=CARTESIAN_POINT('Ctrl Pts',(0.162248711501603,0.0449185271683059,
1.56513903299191));
#29925=CARTESIAN_POINT('Ctrl Pts',(0.153524147106197,0.0653993692500711,
1.56663453131835));
#29926=CARTESIAN_POINT('Ctrl Pts',(0.131911960142923,0.116133797718439,
1.57033912767062));
#29927=CARTESIAN_POINT('Ctrl Pts',(0.0826635066749161,0.155095554237362,
1.57404372402289));
#29928=CARTESIAN_POINT('Ctrl Pts',(0.028317337914343,0.164453369456362,
1.57774832037515));
#29929=CARTESIAN_POINT('Ctrl Pts',(-0.026028830846231,0.173811184675361,
1.58145291672742));
#29930=CARTESIAN_POINT('Ctrl Pts',(-0.0854727148993724,0.153565058594437,
1.58515751307969));
#29931=CARTESIAN_POINT('Ctrl Pts',(-0.122808942133701,0.11298112966685,
1.58886210943196));
#29932=CARTESIAN_POINT('Ctrl Pts',(-0.160145169368031,0.0723972007392629,
1.59256670578423));
#29933=CARTESIAN_POINT('Ctrl Pts',(-0.175373739783547,0.0114754689650147,
1.59627130213649));
#29934=CARTESIAN_POINT('Ctrl Pts',(-0.161526248741115,-0.041903625100424,
1.59997589848876));
#29935=CARTESIAN_POINT('Ctrl Pts',(-0.147678757698683,-0.0952827191658612,
1.60368049484103));
#29936=CARTESIAN_POINT('Ctrl Pts',(-0.1047552051983,-0.14111917552249,1.6073850911933));
#29937=CARTESIAN_POINT('Ctrl Pts',(-0.0523978126792817,-0.158434271662077,
1.61108968754557));
#29938=CARTESIAN_POINT('Ctrl Pts',(-4.04201602626775E-5,-0.175749367801665,
1.61479428389783));
#29939=CARTESIAN_POINT('Ctrl Pts',(0.0617508123773913,-0.164543103724215,
1.6184988802501));
#29940=CARTESIAN_POINT('Ctrl Pts',(0.104692974268098,-0.12994678668867,
1.62220347660237));
#29941=CARTESIAN_POINT('Ctrl Pts',(0.143117393875163,-0.0989901849689851,
1.62551832984792));
#29942=CARTESIAN_POINT('Ctrl Pts',(0.166450162079376,-0.0493061599110598,
1.62883318309347));
#29943=CARTESIAN_POINT('Ctrl Pts',(0.166796959880497,9.66735530056473E-5,
1.63214803633902));
#29944=CARTESIAN_POINT('Ctrl Pts',(0.166752921449725,-0.000121400228749406,
1.61285196366098));
#29945=CARTESIAN_POINT('Ctrl Pts',(0.166815929443988,-0.00780399726549495,
1.61233684282289));
#29946=CARTESIAN_POINT('Ctrl Pts',(0.166330935441723,-0.0154786041905287,
1.6118217219848));
#29947=CARTESIAN_POINT('Ctrl Pts',(0.165270714247807,-0.0230729153352646,
1.61130660114671));
#29948=CARTESIAN_POINT('Ctrl Pts',(0.157645917739612,-0.0776889496409508,
1.60760200479444));
#29949=CARTESIAN_POINT('Ctrl Pts',(0.120270025894947,-0.128152038033383,
1.60389740844217));
#29950=CARTESIAN_POINT('Ctrl Pts',(0.0702485553938763,-0.151366836780329,
1.6001928120899));
#29951=CARTESIAN_POINT('Ctrl Pts',(0.0202270848928061,-0.174581635527273,
1.59648821573763));
#29952=CARTESIAN_POINT('Ctrl Pts',(-0.0424399642646696,-0.170548144628732,
1.59278361938537));
#29953=CARTESIAN_POINT('Ctrl Pts',(-0.0890727806898626,-0.141112640607554,
1.5890790230331));
#29954=CARTESIAN_POINT('Ctrl Pts',(-0.135705597115056,-0.111677136586376,
1.58537442668083));
#29955=CARTESIAN_POINT('Ctrl Pts',(-0.166304180807966,-0.0568396194425618,
1.58166983032856));
#29956=CARTESIAN_POINT('Ctrl Pts',(-0.16686485427816,-0.00169661928996206,
1.57796523397629));
#29957=CARTESIAN_POINT('Ctrl Pts',(-0.167425527748354,0.0534463808626376,
1.57426063762402));
#29958=CARTESIAN_POINT('Ctrl Pts',(-0.137948290995833,0.108894864024023,
1.57055604127176));
#29959=CARTESIAN_POINT('Ctrl Pts',(-0.0919236010333964,0.139272428377062,
1.56685144491949));
#29960=CARTESIAN_POINT('Ctrl Pts',(-0.0458989110709602,0.169649992730101,
1.56314684856722));
#29961=CARTESIAN_POINT('Ctrl Pts',(0.0166732321013904,0.174956638274794,
1.55944225221495));
#29962=CARTESIAN_POINT('Ctrl Pts',(0.0671563493099001,0.152763795116617,
1.55573765586268));
#29963=CARTESIAN_POINT('Ctrl Pts',(0.117639466518409,0.13057095195844,1.55203305951042));
#29964=CARTESIAN_POINT('Ctrl Pts',(0.156033557763077,0.0808786200973942,
1.54832846315815));
#29965=CARTESIAN_POINT('Ctrl Pts',(0.164767340619488,0.0264287526812992,
1.54462386680588));
#29966=CARTESIAN_POINT('Ctrl Pts',(0.166159792575437,0.0177476547388351,
1.54403323242425));
#29967=CARTESIAN_POINT('Ctrl Pts',(0.166798314017023,0.0089456257803759,
1.54344259804261));
#29968=CARTESIAN_POINT('Ctrl Pts',(0.166721717270512,0.00013247748987999,
1.54285196366098));
#29969=CARTESIAN_POINT('Origin',(0.,0.,1.3));
#29970=CARTESIAN_POINT('',(0.166334949033457,3.80241454671915E-5,1.47285196366098));
#29971=CARTESIAN_POINT('',(0.166495616539739,-0.000143126867227327,1.49214803633902));
#29972=CARTESIAN_POINT('',(0.1666,2.04026156737949E-17,1.3));
#29973=CARTESIAN_POINT('Ctrl Pts',(0.166495616539739,-0.000143126867227327,
1.49214803633902));
#29974=CARTESIAN_POINT('Ctrl Pts',(0.166176505544999,0.0388065957770001,
1.49474928988519));
#29975=CARTESIAN_POINT('Ctrl Pts',(0.15254095518154,0.0779576027494656,
1.49735054343136));
#29976=CARTESIAN_POINT('Ctrl Pts',(0.127581990737563,0.107562045989894,
1.49995179697752));
#29977=CARTESIAN_POINT('Ctrl Pts',(0.0920364789316288,0.149723454131357,
1.50365639332979));
#29978=CARTESIAN_POINT('Ctrl Pts',(0.0335245204022979,0.172522270232617,
1.50736098968206));
#29979=CARTESIAN_POINT('Ctrl Pts',(-0.0211755609783529,0.165524482759979,
1.51106558603433));
#29980=CARTESIAN_POINT('Ctrl Pts',(-0.0758756423590036,0.158526695287341,
1.5147701823866));
#29981=CARTESIAN_POINT('Ctrl Pts',(-0.126763846590974,0.121732304240806,
1.51847477873887));
#29982=CARTESIAN_POINT('Ctrl Pts',(-0.150550887470885,0.0719804791091254,
1.52217937509113));
#29983=CARTESIAN_POINT('Ctrl Pts',(-0.174337928350795,0.0222286539774451,
1.5258839714434));
#29984=CARTESIAN_POINT('Ctrl Pts',(-0.171023805878645,-0.0404806052393804,
1.52958856779567));
#29985=CARTESIAN_POINT('Ctrl Pts',(-0.142125268024159,-0.0874480653886775,
1.53329316414794));
#29986=CARTESIAN_POINT('Ctrl Pts',(-0.113226730169674,-0.134415525537975,
1.5369977605002));
#29987=CARTESIAN_POINT('Ctrl Pts',(-0.058743776932853,-0.165641186619743,
1.54070235685247));
#29988=CARTESIAN_POINT('Ctrl Pts',(-0.00361080053401195,-0.166834419219364,
1.54440695320474));
#29989=CARTESIAN_POINT('Ctrl Pts',(0.0515221758648292,-0.168027651818985,
1.54811154955701));
#29990=CARTESIAN_POINT('Ctrl Pts',(0.10730517542569,-0.139188455936458,
1.55181614590928));
#29991=CARTESIAN_POINT('Ctrl Pts',(0.138208714976851,-0.0935153077862871,
1.55552074226154));
#29992=CARTESIAN_POINT('Ctrl Pts',(0.15663688952593,-0.0662798273674848,
1.55772984028737));
#29993=CARTESIAN_POINT('Ctrl Pts',(0.166218204462953,-0.0330583805181475,
1.5599389383132));
#29994=CARTESIAN_POINT('Ctrl Pts',(0.166368100504911,8.32215516180223E-5,
1.56214803633902));
#29995=CARTESIAN_POINT('Ctrl Pts',(0.166721717270512,0.00013247748987999,
1.54285196366098));
#29996=CARTESIAN_POINT('Ctrl Pts',(0.16631788138976,-0.0463324921623522,
1.53973800169035));
#29997=CARTESIAN_POINT('Ctrl Pts',(0.146036306492028,-0.0931065396480778,
1.53662403971971));
#29998=CARTESIAN_POINT('Ctrl Pts',(0.111564911721182,-0.124096839839778,
1.53351007774908));
#29999=CARTESIAN_POINT('Ctrl Pts',(0.0705552254983152,-0.160965161973612,
1.52980548139681));
#30000=CARTESIAN_POINT('Ctrl Pts',(0.00946237858443097,-0.175494403270137,
1.52610088504454));
#30001=CARTESIAN_POINT('Ctrl Pts',(-0.043754143626611,-0.161035180693733,
1.52239628869227));
#30002=CARTESIAN_POINT('Ctrl Pts',(-0.0969706658376549,-0.146575958117328,
1.51869169234));
#30003=CARTESIAN_POINT('Ctrl Pts',(-0.142310863345855,-0.103128271667992,
1.51498709598774));
#30004=CARTESIAN_POINT('Ctrl Pts',(-0.159024536403123,-0.0505761979513979,
1.51128249963547));
#30005=CARTESIAN_POINT('Ctrl Pts',(-0.175738209460389,0.00197587576519482,
1.5075779032832));
#30006=CARTESIAN_POINT('Ctrl Pts',(-0.163825358066725,0.0636323367490458,
1.50387330693093));
#30007=CARTESIAN_POINT('Ctrl Pts',(-0.128737966872089,0.106175754206211,
1.50016871057866));
#30008=CARTESIAN_POINT('Ctrl Pts',(-0.0936505756774527,0.148719171663375,
1.4964641142264));
#30009=CARTESIAN_POINT('Ctrl Pts',(-0.035388644681846,0.172149545593854,
1.49275951787413));
#30010=CARTESIAN_POINT('Ctrl Pts',(0.0193839233712769,0.165743833453852,
1.48905492152186));
#30011=CARTESIAN_POINT('Ctrl Pts',(0.0741564914244009,0.159338121313851,
1.48535032516959));
#30012=CARTESIAN_POINT('Ctrl Pts',(0.125439696535041,0.123096323103367,
1.48164572881732));
#30013=CARTESIAN_POINT('Ctrl Pts',(0.149763488908927,0.07360470278495,1.47794113246505));
#30014=CARTESIAN_POINT('Ctrl Pts',(0.160901714109468,0.0509417559807338,
1.4762447428637));
#30015=CARTESIAN_POINT('Ctrl Pts',(0.166386928169176,0.0255005071147636,
1.47454835326234));
#30016=CARTESIAN_POINT('Ctrl Pts',(0.166334949033457,3.80241454671915E-5,
1.47285196366098));
#30017=CARTESIAN_POINT('Origin',(0.,0.,1.3));
#30018=CARTESIAN_POINT('',(0.166582270817784,-0.000152340582006284,1.40285196366098));
#30019=CARTESIAN_POINT('',(0.166873478424592,6.71112968702338E-7,1.42214803633902));
#30020=CARTESIAN_POINT('',(0.1666,2.04026156737949E-17,1.3));
#30021=CARTESIAN_POINT('Ctrl Pts',(0.166873476951752,6.71109354370205E-7,
1.42214803633902));
#30022=CARTESIAN_POINT('Ctrl Pts',(0.166876772816304,0.0551824619258391,
1.42585504510491));
#30023=CARTESIAN_POINT('Ctrl Pts',(0.136792549878611,0.110361163623334,
1.42956205387081));
#30024=CARTESIAN_POINT('Ctrl Pts',(0.0904117910907898,0.140258570073462,
1.4332690626367));
#30025=CARTESIAN_POINT('Ctrl Pts',(0.0440612155535343,0.170136520159922,
1.43697365898897));
#30026=CARTESIAN_POINT('Ctrl Pts',(-0.0185646804667758,0.174766068965047,
1.44067825534124));
#30027=CARTESIAN_POINT('Ctrl Pts',(-0.0688048006597445,0.152028477144375,
1.4443828516935));
#30028=CARTESIAN_POINT('Ctrl Pts',(-0.119044920852713,0.129290885323702,
1.44808744804577));
#30029=CARTESIAN_POINT('Ctrl Pts',(-0.15689926521834,0.0791861528772324,
1.45179204439804));
#30030=CARTESIAN_POINT('Ctrl Pts',(-0.165043578186289,0.0246449948801753,
1.45549664075031));
#30031=CARTESIAN_POINT('Ctrl Pts',(-0.173187891154238,-0.0298961631168814,
1.45920123710258));
#30032=CARTESIAN_POINT('Ctrl Pts',(-0.15162217272451,-0.088873746664526,
1.46290583345484));
#30033=CARTESIAN_POINT('Ctrl Pts',(-0.110216096648825,-0.125296330528958,
1.46661042980711));
#30034=CARTESIAN_POINT('Ctrl Pts',(-0.0688100205731403,-0.16171891439339,
1.47031502615938));
#30035=CARTESIAN_POINT('Ctrl Pts',(-0.00756358685149875,-0.17558649857461,
1.47401962251165));
#30036=CARTESIAN_POINT('Ctrl Pts',(0.0454934276490607,-0.160552503958399,
1.47772421886392));
#30037=CARTESIAN_POINT('Ctrl Pts',(0.0985504421496201,-0.145518509342189,
1.48142881521618));
#30038=CARTESIAN_POINT('Ctrl Pts',(0.143418037429097,-0.101582935928549,
1.48513341156845));
#30039=CARTESIAN_POINT('Ctrl Pts',(0.159562302527567,-0.0488531491308943,
1.48883800792072));
#30040=CARTESIAN_POINT('Ctrl Pts',(0.164370561528649,-0.0331485958143723,
1.48994135072682));
#30041=CARTESIAN_POINT('Ctrl Pts',(0.166630970058396,-0.0166639678834416,
1.49104469353292));
#30042=CARTESIAN_POINT('Ctrl Pts',(0.166495616539739,-0.000143126867227327,
1.49214803633902));
#30043=CARTESIAN_POINT('Ctrl Pts',(0.166334949033457,3.80241454671915E-5,
1.47285196366098));
#30044=CARTESIAN_POINT('Ctrl Pts',(0.166273415497072,-0.0301047745093415,
1.47084375691007));
#30045=CARTESIAN_POINT('Ctrl Pts',(0.158451996361882,-0.0602773308783548,
1.46883555015916));
#30046=CARTESIAN_POINT('Ctrl Pts',(0.143062834518306,-0.085905647341766,
1.46682734340825));
#30047=CARTESIAN_POINT('Ctrl Pts',(0.114674008116665,-0.133182934723717,
1.46312274705598));
#30048=CARTESIAN_POINT('Ctrl Pts',(0.060531975676251,-0.16499606706127,
1.45941815070371));
#30049=CARTESIAN_POINT('Ctrl Pts',(0.00541514530056254,-0.166785584082033,
1.45571355435145));
#30050=CARTESIAN_POINT('Ctrl Pts',(-0.0497016850751255,-0.168575101102797,
1.45200895799918));
#30051=CARTESIAN_POINT('Ctrl Pts',(-0.105793313386088,-0.14034100280677,
1.44830436164691));
#30052=CARTESIAN_POINT('Ctrl Pts',(-0.137189087849022,-0.0950047843070436,
1.44459976529464));
#30053=CARTESIAN_POINT('Ctrl Pts',(-0.168584862311956,-0.0496685658073169,
1.44089516894238));
#30054=CARTESIAN_POINT('Ctrl Pts',(-0.175284782926862,0.0127697728961095,
1.43719057259011));
#30055=CARTESIAN_POINT('Ctrl Pts',(-0.154222593046579,0.0637349720094271,
1.43348597623784));
#30056=CARTESIAN_POINT('Ctrl Pts',(-0.133160403166296,0.114700171122744,
1.42978137988557));
#30057=CARTESIAN_POINT('Ctrl Pts',(-0.0843361027908238,0.154192230645953,
1.4260767835333));
#30058=CARTESIAN_POINT('Ctrl Pts',(-0.0300944098326194,0.16413738562223,
1.42237218718103));
#30059=CARTESIAN_POINT('Ctrl Pts',(0.0241472831255854,0.174082540598506,
1.41866759082877));
#30060=CARTESIAN_POINT('Ctrl Pts',(0.0838063686665219,0.154480791027852,
1.4149629944765));
#30061=CARTESIAN_POINT('Ctrl Pts',(0.121579527998707,0.114302988740736,
1.41125839812423));
#30062=CARTESIAN_POINT('Ctrl Pts',(0.150151024791829,0.0839126277146479,
1.40845625330315));
#30063=CARTESIAN_POINT('Ctrl Pts',(0.166200792747313,0.0417499637845381,
1.40565410848206));
#30064=CARTESIAN_POINT('Ctrl Pts',(0.166582270817784,-0.000152340582006284,
1.40285196366098));
#30065=CARTESIAN_POINT('Origin',(0.,0.,1.3));
#30066=CARTESIAN_POINT('',(0.16685129292948,5.5034311338048E-5,1.33285196366098));
#30067=CARTESIAN_POINT('',(0.166493658714001,0.000142704933107348,1.35214803633902));
#30068=CARTESIAN_POINT('',(0.1666,2.04026156737949E-17,1.3));
#30069=CARTESIAN_POINT('Ctrl Pts',(0.166493658714001,0.000142704933107348,
1.35214803633902));
#30070=CARTESIAN_POINT('Ctrl Pts',(0.166629086818581,0.0167362841743647,
1.35325620397237));
#30071=CARTESIAN_POINT('Ctrl Pts',(0.164348470273229,0.0332934752509887,
1.35436437160572));
#30072=CARTESIAN_POINT('Ctrl Pts',(0.159498696116421,0.0490604157264683,
1.35547253923907));
#30073=CARTESIAN_POINT('Ctrl Pts',(0.143285936322738,0.101769183257714,
1.35917713559134));
#30074=CARTESIAN_POINT('Ctrl Pts',(0.0983612975566499,0.145646425810988,
1.36288173194361));
#30075=CARTESIAN_POINT('Ctrl Pts',(0.0452847954907157,0.16061147453177,
1.36658632829587));
#30076=CARTESIAN_POINT('Ctrl Pts',(-0.00779170657521921,0.175576523252552,
1.37029092464814));
#30077=CARTESIAN_POINT('Ctrl Pts',(-0.0690200719410003,0.161629378140841,
1.37399552100041));
#30078=CARTESIAN_POINT('Ctrl Pts',(-0.11037879201089,0.125153029241032,
1.37770011735268));
#30079=CARTESIAN_POINT('Ctrl Pts',(-0.151737512080778,0.0886766803412233,
1.38140471370495));
#30080=CARTESIAN_POINT('Ctrl Pts',(-0.173226586854776,0.0296711276533176,
1.38510931005721));
#30081=CARTESIAN_POINT('Ctrl Pts',(-0.165011419406707,-0.0248594030476235,
1.38881390640948));
#30082=CARTESIAN_POINT('Ctrl Pts',(-0.156796251958638,-0.0793899337485655,
1.39251850276175));
#30083=CARTESIAN_POINT('Ctrl Pts',(-0.1188768422885,-0.129445442462543,
1.39622309911402));
#30084=CARTESIAN_POINT('Ctrl Pts',(-0.0686072232581569,-0.152117741798697,
1.39992769546629));
#30085=CARTESIAN_POINT('Ctrl Pts',(-0.0183376042278136,-0.174790041134852,
1.40363229181856));
#30086=CARTESIAN_POINT('Ctrl Pts',(0.0442822241627354,-0.170079131093183,
1.40733688817082));
#30087=CARTESIAN_POINT('Ctrl Pts',(0.0905939423885369,-0.140140986355195,
1.41104148452309));
#30088=CARTESIAN_POINT('Ctrl Pts',(0.136875502667449,-0.110222337179314,
1.41474366846173));
#30089=CARTESIAN_POINT('Ctrl Pts',(0.166870185376906,-0.0551092982940088,
1.41844585240038));
#30090=CARTESIAN_POINT('Ctrl Pts',(0.166873476951752,6.71109354370205E-7,
1.42214803633902));
#30091=CARTESIAN_POINT('Ctrl Pts',(0.166582270817784,-0.000152340582006284,
1.40285196366098));
#30092=CARTESIAN_POINT('Ctrl Pts',(0.166705128660898,-0.0136472886129686,
1.4019495121298));
#30093=CARTESIAN_POINT('Ctrl Pts',(0.165202856095667,-0.0271152318944043,
1.40104706059861));
#30094=CARTESIAN_POINT('Ctrl Pts',(0.161970345045233,-0.0401542300245841,
1.40014460906743));
#30095=CARTESIAN_POINT('Ctrl Pts',(0.148700769636142,-0.0936797914992128,
1.39644001271516));
#30096=CARTESIAN_POINT('Ctrl Pts',(0.106274385694529,-0.139977059444894,
1.39273541636289));
#30097=CARTESIAN_POINT('Ctrl Pts',(0.054107868404235,-0.157857826665655,
1.38903082001062));
#30098=CARTESIAN_POINT('Ctrl Pts',(0.00194135111394122,-0.175738593886417,
1.38532622365835));
#30099=CARTESIAN_POINT('Ctrl Pts',(-0.0599652995250327,-0.165202860382259,
1.38162162730609));
#30100=CARTESIAN_POINT('Ctrl Pts',(-0.103280153812656,-0.131072364331603,
1.37791703095382));
#30101=CARTESIAN_POINT('Ctrl Pts',(-0.146595008100279,-0.0969418682809483,
1.37421243460155));
#30102=CARTESIAN_POINT('Ctrl Pts',(-0.171318066036552,-0.0392166096837955,
1.37050783824928));
#30103=CARTESIAN_POINT('Ctrl Pts',(-0.166134679967937,0.0156851195376423,
1.36680324189701));
#30104=CARTESIAN_POINT('Ctrl Pts',(-0.160951293899322,0.0705868487590808,
1.36309864554474));
#30105=CARTESIAN_POINT('Ctrl Pts',(-0.12586146382582,0.122665048604804,
1.35939404919248));
#30106=CARTESIAN_POINT('Ctrl Pts',(-0.0769242494532953,0.14808583561233,
1.35568945284021));
#30107=CARTESIAN_POINT('Ctrl Pts',(-0.0279870350807717,0.173506622619856,
1.35198485648794));
#30108=CARTESIAN_POINT('Ctrl Pts',(0.0347975635907744,0.172269996789183,
1.34828026013567));
#30109=CARTESIAN_POINT('Ctrl Pts',(0.0826958189663461,0.144941906943662,
1.3445756637834));
#30110=CARTESIAN_POINT('Ctrl Pts',(0.130594074341918,0.117613817098141,
1.34087106743114));
#30111=CARTESIAN_POINT('Ctrl Pts',(0.163605986421516,0.0641942632377707,
1.33716647107887));
#30112=CARTESIAN_POINT('Ctrl Pts',(0.166623466451679,0.00913100709632859,
1.3334618747266));
#30113=CARTESIAN_POINT('Ctrl Pts',(0.166789062042101,0.00610920336601207,
1.33325857103806));
#30114=CARTESIAN_POINT('Ctrl Pts',(0.16686432402183,0.00308244933152886,
1.33305526734952));
#30115=CARTESIAN_POINT('Ctrl Pts',(0.16685129292948,5.5034311338048E-5,
1.33285196366098));
#30116=CARTESIAN_POINT('Origin',(0.,0.,1.3));
#30117=CARTESIAN_POINT('',(0.166419792426106,0.000117644517947116,1.26285196366098));
#30118=CARTESIAN_POINT('',(0.166369239667266,-8.42498788368234E-5,1.28214803633902));
#30119=CARTESIAN_POINT('',(0.1666,2.04026156737949E-17,1.3));
#30120=CARTESIAN_POINT('Ctrl Pts',(0.166369239667266,-8.42498788368234E-5,
1.28214803633902));
#30121=CARTESIAN_POINT('Ctrl Pts',(0.166217137033255,0.0331292003521081,
1.2843619591921));
#30122=CARTESIAN_POINT('Ctrl Pts',(0.156590960021794,0.0664238537129591,
1.28657588204517));
#30123=CARTESIAN_POINT('Ctrl Pts',(0.138087078302622,0.093694809140457,
1.28878980489824));
#30124=CARTESIAN_POINT('Ctrl Pts',(0.107124205036991,0.139327782240334,
1.29249440125051));
#30125=CARTESIAN_POINT('Ctrl Pts',(0.051303827751912,0.168094448054701,
1.29619899760278));
#30126=CARTESIAN_POINT('Ctrl Pts',(-0.00382754136500674,0.166829578855541,
1.29990359395505));
#30127=CARTESIAN_POINT('Ctrl Pts',(-0.0589589104819255,0.16556470965638,
1.30360819030732));
#30128=CARTESIAN_POINT('Ctrl Pts',(-0.113401271430684,0.134268305443692,
1.30731278665959));
#30129=CARTESIAN_POINT('Ctrl Pts',(-0.142238769013948,0.0872633430680612,
1.31101738301185));
#30130=CARTESIAN_POINT('Ctrl Pts',(-0.171076266597211,0.0402583806924305,
1.31472197936412));
#30131=CARTESIAN_POINT('Ctrl Pts',(-0.17430890081498,-0.0224551398461431,
1.31842657571639));
#30132=CARTESIAN_POINT('Ctrl Pts',(-0.150457238287118,-0.0721760202632685,
1.32213117206866));
#30133=CARTESIAN_POINT('Ctrl Pts',(-0.126605575759256,-0.121896900680394,
1.32583576842093));
#30134=CARTESIAN_POINT('Ctrl Pts',(-0.0756696164857624,-0.158625140976071,
1.32954036477319));
#30135=CARTESIAN_POINT('Ctrl Pts',(-0.0209604910548609,-0.165551853715821,
1.33324496112546));
#30136=CARTESIAN_POINT('Ctrl Pts',(0.0337486343760406,-0.17247856645557,
1.33694955747773));
#30137=CARTESIAN_POINT('Ctrl Pts',(0.0922309259643503,-0.149603751639392,
1.34065415383));
#30138=CARTESIAN_POINT('Ctrl Pts',(0.127721631347866,-0.107396197976694,
1.34435875018227));
#30139=CARTESIAN_POINT('Ctrl Pts',(0.152595889688052,-0.0778143234445287,
1.34695517890118));
#30140=CARTESIAN_POINT('Ctrl Pts',(0.166176351648266,-0.038735930748939,
1.3495516076201));
#30141=CARTESIAN_POINT('Ctrl Pts',(0.166493658714001,0.000142704933107348,
1.35214803633902));
#30142=CARTESIAN_POINT('Ctrl Pts',(0.16685129292948,5.5034311338048E-5,
1.33285196366098));
#30143=CARTESIAN_POINT('Ctrl Pts',(0.16662687167882,-0.0520830556384961,
1.32935067099725));
#30144=CARTESIAN_POINT('Ctrl Pts',(0.140215016815216,-0.104417191766459,
1.32584937833352));
#30145=CARTESIAN_POINT('Ctrl Pts',(0.0980387654551791,-0.135037607098881,
1.3223480856698));
#30146=CARTESIAN_POINT('Ctrl Pts',(0.0534135364477915,-0.167436006730135,
1.31864348931753));
#30147=CARTESIAN_POINT('Ctrl Pts',(-0.00885996954770948,-0.175525847570128,
1.31493889296526));
#30148=CARTESIAN_POINT('Ctrl Pts',(-0.0602819293976768,-0.155604768085892,
1.31123429661299));
#30149=CARTESIAN_POINT('Ctrl Pts',(-0.111703889247644,-0.135683688601655,
1.30752970026073));
#30150=CARTESIAN_POINT('Ctrl Pts',(-0.152274302952078,-0.0877516887931891,
1.30382510390846));
#30151=CARTESIAN_POINT('Ctrl Pts',(-0.163425890629257,-0.0337451201657775,
1.30012050755619));
#30152=CARTESIAN_POINT('Ctrl Pts',(-0.174577478306436,0.0202614484616345,
1.29641591120392));
#30153=CARTESIAN_POINT('Ctrl Pts',(-0.15631023995636,0.0803425859079921,
1.29271131485165));
#30154=CARTESIAN_POINT('Ctrl Pts',(-0.116984280792225,0.119001818937757,
1.28900671849938));
#30155=CARTESIAN_POINT('Ctrl Pts',(-0.077658321628091,0.157661051967521,
1.28530212214712));
#30156=CARTESIAN_POINT('Ctrl Pts',(-0.0172736416498982,0.174898380580693,
1.28159752579485));
#30157=CARTESIAN_POINT('Ctrl Pts',(0.0365343679459083,0.162825043595149,
1.27789292944258));
#30158=CARTESIAN_POINT('Ctrl Pts',(0.090342377541716,0.150751706609605,
1.27418833309031));
#30159=CARTESIAN_POINT('Ctrl Pts',(0.137573716755137,0.109367704025345,
1.27048373673804));
#30160=CARTESIAN_POINT('Ctrl Pts',(0.15661269537524,0.0576126592883118,
1.26677914038578));
#30161=CARTESIAN_POINT('Ctrl Pts',(0.163340322948393,0.0393244583837232,
1.26547008147751));
#30162=CARTESIAN_POINT('Ctrl Pts',(0.166547744893355,0.0197412896159237,
1.26416102256925));
#30163=CARTESIAN_POINT('Ctrl Pts',(0.166419792426106,0.000117644517947116,
1.26285196366098));
#30164=CARTESIAN_POINT('Origin',(0.,0.,1.3));
#30165=CARTESIAN_POINT('',(0.166426142970557,-0.000120642765556289,1.19285196366098));
#30166=CARTESIAN_POINT('',(0.16680112293357,-9.74720745467285E-5,1.21214803633902));
#30167=CARTESIAN_POINT('',(0.1666,2.04026156737949E-17,1.3));
#30168=CARTESIAN_POINT('Ctrl Pts',(0.16680112293357,-9.74720745467285E-5,
1.21214803633902));
#30169=CARTESIAN_POINT('Ctrl Pts',(0.166457232615762,0.0493755335317627,
1.21546771441182));
#30170=CARTESIAN_POINT('Ctrl Pts',(0.143044424972525,0.0991312161213854,
1.21878739248462));
#30171=CARTESIAN_POINT('Ctrl Pts',(0.104522946124804,0.130083481608585,
1.22210707055742));
#30172=CARTESIAN_POINT('Ctrl Pts',(0.0615348831579396,0.164624677261814,
1.22581166690969));
#30173=CARTESIAN_POINT('Ctrl Pts',(-0.000268695245690821,0.175749122363903,
1.22951626326196));
#30174=CARTESIAN_POINT('Ctrl Pts',(-0.0526030309795398,0.15836565153399,
1.23322085961422));
#30175=CARTESIAN_POINT('Ctrl Pts',(-0.104937366713389,0.140982180704076,
1.23692545596649));
#30176=CARTESIAN_POINT('Ctrl Pts',(-0.147802459777456,0.0950907939421611,
1.24063005231876));
#30177=CARTESIAN_POINT('Ctrl Pts',(-0.161580857269364,0.0416939446216941,
1.24433464867103));
#30178=CARTESIAN_POINT('Ctrl Pts',(-0.175359254761272,-0.0117029046987729,
1.2480392450233));
#30179=CARTESIAN_POINT('Ctrl Pts',(-0.16005095668102,-0.0726052165777916,
1.25174384137556));
#30180=CARTESIAN_POINT('Ctrl Pts',(-0.122661892448987,-0.113140702644331,
1.25544843772783));
#30181=CARTESIAN_POINT('Ctrl Pts',(-0.0852728282169544,-0.15367618871087,
1.2591530340801));
#30182=CARTESIAN_POINT('Ctrl Pts',(-0.0258029978331414,-0.17384484896493,
1.26285763043237));
#30183=CARTESIAN_POINT('Ctrl Pts',(0.0285308936104228,-0.164416381677161,
1.26656222678464));
#30184=CARTESIAN_POINT('Ctrl Pts',(0.0828647850539866,-0.154987914389393,
1.2702668231369));
#30185=CARTESIAN_POINT('Ctrl Pts',(0.132062737557302,-0.115962319559795,
1.27397141948917));
#30186=CARTESIAN_POINT('Ctrl Pts',(0.153609029185868,-0.0651998819523026,
1.27767601584144));
#30187=CARTESIAN_POINT('Ctrl Pts',(0.162278930811433,-0.044773845401895,
1.27916668934063));
#30188=CARTESIAN_POINT('Ctrl Pts',(0.166471653066795,-0.022447454634266,
1.28065736283983));
#30189=CARTESIAN_POINT('Ctrl Pts',(0.166369239667266,-8.42498788368234E-5,
1.28214803633902));
#30190=CARTESIAN_POINT('Ctrl Pts',(0.166419792426106,0.000117644517947116,
1.26285196366098));
#30191=CARTESIAN_POINT('Ctrl Pts',(0.166185643355799,-0.0357930210168177,
1.26045642621698));
#30192=CARTESIAN_POINT('Ctrl Pts',(0.154782035268061,-0.0718392331665093,
1.25806088877297));
#30193=CARTESIAN_POINT('Ctrl Pts',(0.133341646618848,-0.100333245437109,
1.25566535132897));
#30194=CARTESIAN_POINT('Ctrl Pts',(0.100185001215565,-0.144398018535696,
1.2519607549767));
#30195=CARTESIAN_POINT('Ctrl Pts',(0.0430250923822119,-0.170401477843065,
1.24825615862443));
#30196=CARTESIAN_POINT('Ctrl Pts',(-0.0119785234848996,-0.166442992757554,
1.24455156227217));
#30197=CARTESIAN_POINT('Ctrl Pts',(-0.0669821393520106,-0.162484507672042,
1.2408469659199));
#30198=CARTESIAN_POINT('Ctrl Pts',(-0.11982946225288,-0.12856407819365,
1.23714236956763));
#30199=CARTESIAN_POINT('Ctrl Pts',(-0.146334615197223,-0.0802055812150856,
1.23343777321536));
#30200=CARTESIAN_POINT('Ctrl Pts',(-0.172839768141565,-0.0318470842365214,
1.22973317686309));
#30201=CARTESIAN_POINT('Ctrl Pts',(-0.17300275112938,0.0309494802422141,
1.22602858051083));
#30202=CARTESIAN_POINT('Ctrl Pts',(-0.14674897407212,0.0794449084066994,
1.22232398415856));
#30203=CARTESIAN_POINT('Ctrl Pts',(-0.12049519701486,0.127940336571185,
1.21861938780629));
#30204=CARTESIAN_POINT('Ctrl Pts',(-0.0678246599125219,0.162134628421419,
1.21491479145402));
#30205=CARTESIAN_POINT('Ctrl Pts',(-0.01284233273225,0.166378572397304,
1.21121019510176));
#30206=CARTESIAN_POINT('Ctrl Pts',(0.0421399944480223,0.170622516373188,
1.20750559874949));
#30207=CARTESIAN_POINT('Ctrl Pts',(0.0994341117062293,0.144916112474723,
1.20380100239722));
#30208=CARTESIAN_POINT('Ctrl Pts',(0.132819041399409,0.101024042211295,
1.20009640604495));
#30209=CARTESIAN_POINT('Ctrl Pts',(0.154580764464244,0.0724133161563545,
1.19768159191696));
#30210=CARTESIAN_POINT('Ctrl Pts',(0.166183499569454,0.0360755201147432,
1.19526677778897));
#30211=CARTESIAN_POINT('Ctrl Pts',(0.166426142970557,-0.000120642765556289,
1.19285196366098));
#30212=CARTESIAN_POINT('Origin',(0.,0.,1.3));
#30213=CARTESIAN_POINT('',(0.166855124306607,-5.00565220619177E-5,1.12285196366098));
#30214=CARTESIAN_POINT('',(0.166664543572935,0.000145872469707454,1.14214803633902));
#30215=CARTESIAN_POINT('',(0.1666,2.04026156737949E-17,1.3));
#30216=CARTESIAN_POINT('Ctrl Pts',(0.166664543572935,0.000145872469707454,
1.14214803633902));
#30217=CARTESIAN_POINT('Ctrl Pts',(0.166763206461382,0.0109113832732099,
1.14286887327928));
#30218=CARTESIAN_POINT('Ctrl Pts',(0.165809417829237,0.0216594859626649,
1.14358971021953));
#30219=CARTESIAN_POINT('Ctrl Pts',(0.163739663996808,0.0321882103916611,
1.14431054715979));
#30220=CARTESIAN_POINT('Ctrl Pts',(0.153102580809897,0.0862984701957669,
1.14801514351206));
#30221=CARTESIAN_POINT('Ctrl Pts',(0.112990188231545,0.134614425572516,
1.15171973986433));
#30222=CARTESIAN_POINT('Ctrl Pts',(0.0617601501778567,0.155024005573456,
1.1554243362166));
#30223=CARTESIAN_POINT('Ctrl Pts',(0.010530112124168,0.175433585574396,
1.15912893256886));
#30224=CARTESIAN_POINT('Ctrl Pts',(-0.0518175714048562,0.167936790199525,
1.16283352892113));
#30225=CARTESIAN_POINT('Ctrl Pts',(-0.0967491295066884,0.135964570361971,
1.1665381252734));
#30226=CARTESIAN_POINT('Ctrl Pts',(-0.14168068760852,0.103992350524416,
1.17024272162567));
#30227=CARTESIAN_POINT('Ctrl Pts',(-0.16919612028316,0.0475447062241783,
1.17394731797794));
#30228=CARTESIAN_POINT('Ctrl Pts',(-0.166702833743975,-0.00754477804487655,
1.1776519143302));
#30229=CARTESIAN_POINT('Ctrl Pts',(-0.16420954720479,-0.0626342623139314,
1.18135651068247));
#30230=CARTESIAN_POINT('Ctrl Pts',(-0.131707541451779,-0.116365586551803,
1.18506110703474));
#30231=CARTESIAN_POINT('Ctrl Pts',(-0.0840715437167003,-0.144148305543673,
1.18876570338701));
#30232=CARTESIAN_POINT('Ctrl Pts',(-0.0364355459816213,-0.171931024535542,
1.19247029973928));
#30233=CARTESIAN_POINT('Ctrl Pts',(0.0263344437355261,-0.17376513828141,
1.19617489609154));
#30234=CARTESIAN_POINT('Ctrl Pts',(0.0755113837106313,-0.148811254225361,
1.19987949244381));
#30235=CARTESIAN_POINT('Ctrl Pts',(0.124688323685737,-0.123857370169311,
1.20358408879608));
#30236=CARTESIAN_POINT('Ctrl Pts',(0.1602722139188,-0.0721154883113449,
1.20728868514835));
#30237=CARTESIAN_POINT('Ctrl Pts',(0.165977885270282,-0.0172655742801778,
1.21099328150062));
#30238=CARTESIAN_POINT('Ctrl Pts',(0.166570721031857,-0.011566509515692,
1.21137819978008));
#30239=CARTESIAN_POINT('Ctrl Pts',(0.166840997182384,-0.00583389102255577,
1.21176311805955));
#30240=CARTESIAN_POINT('Ctrl Pts',(0.16680112293357,-9.74720745467285E-5,
1.21214803633902));
#30241=CARTESIAN_POINT('Ctrl Pts',(0.166426142970557,-0.000120642765556289,
1.19285196366098));
#30242=CARTESIAN_POINT('Ctrl Pts',(0.166555741825373,-0.0194534630140944,
1.1915621814367));
#30243=CARTESIAN_POINT('Ctrl Pts',(0.163444578249431,-0.0387458787095636,
1.19027239921243));
#30244=CARTESIAN_POINT('Ctrl Pts',(0.156909640667809,-0.0567989395012422,
1.18898261698815));
#30245=CARTESIAN_POINT('Ctrl Pts',(0.138139568114877,-0.108652114321963,
1.18527802063588));
#30246=CARTESIAN_POINT('Ctrl Pts',(0.0911236808808596,-0.150280727335013,
1.18157342428361));
#30247=CARTESIAN_POINT('Ctrl Pts',(0.0373790663566119,-0.162633207744568,
1.17786882793134));
#30248=CARTESIAN_POINT('Ctrl Pts',(-0.0163655481676351,-0.174985688154123,
1.17416423157907));
#30249=CARTESIAN_POINT('Ctrl Pts',(-0.0768388899821125,-0.158062035960183,
1.17045963522681));
#30250=CARTESIAN_POINT('Ctrl Pts',(-0.116364991298242,-0.119607456553155,
1.16675503887454));
#30251=CARTESIAN_POINT('Ctrl Pts',(-0.155891092614372,-0.0811528771461272,
1.16305044252227));
#30252=CARTESIAN_POINT('Ctrl Pts',(-0.174469953432153,-0.0211673705260111,
1.15934584617));
#30253=CARTESIAN_POINT('Ctrl Pts',(-0.163598852749046,0.0328963560619538,
1.15564124981773));
#30254=CARTESIAN_POINT('Ctrl Pts',(-0.152727752065939,0.0869600826499182,
1.15193665346547));
#30255=CARTESIAN_POINT('Ctrl Pts',(-0.112406689881943,0.135102029205731,
1.1482320571132));
#30256=CARTESIAN_POINT('Ctrl Pts',(-0.061088828941493,0.155289760903929,
1.14452746076093));
#30257=CARTESIAN_POINT('Ctrl Pts',(-0.00977096800104246,0.175477492602127,
1.14082286440866));
#30258=CARTESIAN_POINT('Ctrl Pts',(0.0525436916958626,0.16771100944271,
1.13711826805639));
#30259=CARTESIAN_POINT('Ctrl Pts',(0.0973364927906947,0.135544686484056,
1.13341367170413));
#30260=CARTESIAN_POINT('Ctrl Pts',(0.139904197214479,0.10497623587064,1.12989310235641));
#30261=CARTESIAN_POINT('Ctrl Pts',(0.166647613265987,0.0523718751412305,
1.12637253300869));
#30262=CARTESIAN_POINT('Ctrl Pts',(0.166855124306607,-5.00565220619177E-5,
1.12285196366098));
#30263=CARTESIAN_POINT('Origin',(0.,0.,1.3));
#30264=CARTESIAN_POINT('',(0.166573628657937,0.000152187718365226,1.05285196366098));
#30265=CARTESIAN_POINT('',(0.166327182499917,6.33242585386815E-6,1.07214803633902));
#30266=CARTESIAN_POINT('',(0.1666,2.04026156737949E-17,1.3));
#30267=CARTESIAN_POINT('Ctrl Pts',(0.166327182499917,6.33242585386815E-6,
1.07214803633902));
#30268=CARTESIAN_POINT('Ctrl Pts',(0.166336479007403,0.0274263312352492,
1.073974628499));
#30269=CARTESIAN_POINT('Ctrl Pts',(0.159932481000657,0.0548422420648042,
1.07580122065898));
#30270=CARTESIAN_POINT('Ctrl Pts',(0.147091342637332,0.0788092340673142,
1.07762781281897));
#30271=CARTESIAN_POINT('Ctrl Pts',(0.121047633821556,0.127417803124253,
1.08133240917123));
#30272=CARTESIAN_POINT('Ctrl Pts',(0.0685255340861956,0.161839665678967,
1.0850370055235));
#30273=CARTESIAN_POINT('Ctrl Pts',(0.0135620801901698,0.166321461139012,
1.08874160187577));
#30274=CARTESIAN_POINT('Ctrl Pts',(-0.0414013737058552,0.170803256599056,
1.09244619822804));
#30275=CARTESIAN_POINT('Ctrl Pts',(-0.0988061817625453,0.145344984964431,
1.09615079458031));
#30276=CARTESIAN_POINT('Ctrl Pts',(-0.132380708062468,0.101597768611665,
1.09985539093257));
#30277=CARTESIAN_POINT('Ctrl Pts',(-0.165955234362392,0.0578505522588977,
1.10355998728484));
#30278=CARTESIAN_POINT('Ctrl Pts',(-0.175699478905547,-0.00418560881201081,
1.10726458363711));
#30279=CARTESIAN_POINT('Ctrl Pts',(-0.157153932924644,-0.0561195137204682,
1.11096917998938));
#30280=CARTESIAN_POINT('Ctrl Pts',(-0.13860838694374,-0.108053418628926,
1.11467377634165));
#30281=CARTESIAN_POINT('Ctrl Pts',(-0.0917730504387764,-0.149885067374932,
1.11837837269391));
#30282=CARTESIAN_POINT('Ctrl Pts',(-0.0380823807348833,-0.162469968707007,
1.12208296904618));
#30283=CARTESIAN_POINT('Ctrl Pts',(0.0156082889690095,-0.175054870039082,
1.12578756539845));
#30284=CARTESIAN_POINT('Ctrl Pts',(0.076154291871832,-0.158393023957226,
1.12949216175072));
#30285=CARTESIAN_POINT('Ctrl Pts',(0.115846406425509,-0.120109818800568,
1.13319675810299));
#30286=CARTESIAN_POINT('Ctrl Pts',(0.147815265950422,-0.0892757243821015,
1.136180517515));
#30287=CARTESIAN_POINT('Ctrl Pts',(0.16625614840673,-0.044415792438328,
1.13916427692701));
#30288=CARTESIAN_POINT('Ctrl Pts',(0.166664543572935,0.000145872469707454,
1.14214803633902));
#30289=CARTESIAN_POINT('Ctrl Pts',(0.166855124306607,-5.00565220619177E-5,
1.12285196366098));
#30290=CARTESIAN_POINT('Ctrl Pts',(0.166865971312146,-0.00279025280966625,
1.12266793665643));
#30291=CARTESIAN_POINT('Ctrl Pts',(0.166804312774377,-0.00552995063608946,
1.12248390965187));
#30292=CARTESIAN_POINT('Ctrl Pts',(0.166668618800564,-0.00826597665440976,
1.12229988264732));
#30293=CARTESIAN_POINT('Ctrl Pts',(0.163937001222843,-0.0633441540763332,
1.11859528629505));
#30294=CARTESIAN_POINT('Ctrl Pts',(0.131202823574641,-0.116934346162291,
1.11489068994278));
#30295=CARTESIAN_POINT('Ctrl Pts',(0.0834470678717536,-0.144510697621526,
1.11118609359052));
#30296=CARTESIAN_POINT('Ctrl Pts',(0.035691312168866,-0.172087049080761,
1.10748149723825));
#30297=CARTESIAN_POINT('Ctrl Pts',(-0.0270860215887074,-0.173649559913274,
1.10377690088598));
#30298=CARTESIAN_POINT('Ctrl Pts',(-0.0761545306345133,-0.148483138187173,
1.10007230453371));
#30299=CARTESIAN_POINT('Ctrl Pts',(-0.125223039680319,-0.123316716461072,
1.09636770818145));
#30300=CARTESIAN_POINT('Ctrl Pts',(-0.160582724014357,-0.0714213621763564,
1.09266311182918));
#30301=CARTESIAN_POINT('Ctrl Pts',(-0.166051023599269,-0.0165472784677163,
1.08895851547691));
#30302=CARTESIAN_POINT('Ctrl Pts',(-0.171519323184182,0.0383268052409238,
1.08525391912464));
#30303=CARTESIAN_POINT('Ctrl Pts',(-0.147096238019968,0.0961796183734885,
1.08154932277237));
#30304=CARTESIAN_POINT('Ctrl Pts',(-0.103959131518119,0.130534492913072,
1.0778447264201));
#30305=CARTESIAN_POINT('Ctrl Pts',(-0.0608220250162706,0.164889367452656,
1.07414013006784));
#30306=CARTESIAN_POINT('Ctrl Pts',(0.0010291028232132,0.175746303399259,
1.07043553371557));
#30307=CARTESIAN_POINT('Ctrl Pts',(0.0532877326205867,0.15813656252862,
1.0667309373633));
#30308=CARTESIAN_POINT('Ctrl Pts',(0.10554636241796,0.140526821657981,1.06302634101103));
#30309=CARTESIAN_POINT('Ctrl Pts',(0.148212494173223,0.0944504039700999,
1.05932174465876));
#30310=CARTESIAN_POINT('Ctrl Pts',(0.161759730763308,0.0409944431478461,
1.0556171483065));
#30311=CARTESIAN_POINT('Ctrl Pts',(0.165130373342236,0.0276942445097812,
1.05469542009132));
#30312=CARTESIAN_POINT('Ctrl Pts',(0.16669841799434,0.0139372170985273,
1.05377369187615));
#30313=CARTESIAN_POINT('Ctrl Pts',(0.166573628657937,0.000152187718365227,
1.05285196366098));
#30314=CARTESIAN_POINT('Origin',(0.,0.,1.3));
#30315=CARTESIAN_POINT('',(0.16633703813182,-4.26131537097363E-5,0.982851963660979));
#30316=CARTESIAN_POINT('',(0.166641299058679,-0.000149160109009599,1.00214803633902));
#30317=CARTESIAN_POINT('',(0.1666,2.04026156737949E-17,1.3));
#30318=CARTESIAN_POINT('Ctrl Pts',(0.166641299058679,-0.000149160109009599,
1.00214803633902));
#30319=CARTESIAN_POINT('Ctrl Pts',(0.166236990763482,0.0436603970157784,
1.00508038371873));
#30320=CARTESIAN_POINT('Ctrl Pts',(0.148493576846311,0.0877597158867868,
1.00801273109843));
#30321=CARTESIAN_POINT('Ctrl Pts',(0.117498076053599,0.118494559065924,
1.01094507847814));
#30322=CARTESIAN_POINT('Ctrl Pts',(0.0783397485075339,0.157323583456734,
1.01464967483041));
#30323=CARTESIAN_POINT('Ctrl Pts',(0.0180302104029479,0.174822017275825,
1.01835427118268));
#30324=CARTESIAN_POINT('Ctrl Pts',(-0.0358295364409326,0.162981602616999,
1.02205886753494));
#30325=CARTESIAN_POINT('Ctrl Pts',(-0.089689283284813,0.151141187958173,
1.02576346388721));
#30326=CARTESIAN_POINT('Ctrl Pts',(-0.137099238867988,0.10996192482143,
1.02946806023948));
#30327=CARTESIAN_POINT('Ctrl Pts',(-0.156361968042692,0.0582897367165174,
1.03317265659175));
#30328=CARTESIAN_POINT('Ctrl Pts',(-0.175624697217396,0.00661754861160513,
1.03687725294402));
#30329=CARTESIAN_POINT('Ctrl Pts',(-0.166740199983629,-0.0555475644614757,
1.04058184929629));
#30330=CARTESIAN_POINT('Ctrl Pts',(-0.133774516953309,-0.0997553861262926,
1.04428644564855));
#30331=CARTESIAN_POINT('Ctrl Pts',(-0.100808833922988,-0.143963207791109,
1.04799104200082));
#30332=CARTESIAN_POINT('Ctrl Pts',(-0.0437619650961137,-0.170213738047662,
1.05169563835309));
#30333=CARTESIAN_POINT('Ctrl Pts',(0.0112582665697782,-0.166493272809894,
1.05540023470536));
#30334=CARTESIAN_POINT('Ctrl Pts',(0.0662784982356701,-0.162772807572126,
1.05910483105763));
#30335=CARTESIAN_POINT('Ctrl Pts',(0.11927209274058,-0.129081346840038,
1.06280942740989));
#30336=CARTESIAN_POINT('Ctrl Pts',(0.145986231044939,-0.0808379786944121,
1.06651402376216));
#30337=CARTESIAN_POINT('Ctrl Pts',(0.159528668319701,-0.0563815362072228,
1.06839202795445));
#30338=CARTESIAN_POINT('Ctrl Pts',(0.166317624329016,-0.0281854412194699,
1.07027003214673));
#30339=CARTESIAN_POINT('Ctrl Pts',(0.166327182499917,6.33242585386815E-6,
1.07214803633902));
#30340=CARTESIAN_POINT('Ctrl Pts',(0.166573628657937,0.000152187718365227,
1.05285196366098));
#30341=CARTESIAN_POINT('Ctrl Pts',(0.166196866546928,-0.0414673682413184,
1.05006909552388));
#30342=CARTESIAN_POINT('Ctrl Pts',(0.150389111841613,-0.0833421755592448,
1.04728622738679));
#30343=CARTESIAN_POINT('Ctrl Pts',(0.122171212866625,-0.113670355101641,
1.04450335924969));
#30344=CARTESIAN_POINT('Ctrl Pts',(0.0846071169549502,-0.154043688572246,
1.04079876289742));
#30345=CARTESIAN_POINT('Ctrl Pts',(0.0250505837066941,-0.173954851556829,
1.03709416654516));
#30346=CARTESIAN_POINT('Ctrl Pts',(-0.0292420016986911,-0.164291387935873,
1.03338957019289));
#30347=CARTESIAN_POINT('Ctrl Pts',(-0.0835345871040766,-0.154627924314917,
1.02968497384062));
#30348=CARTESIAN_POINT('Ctrl Pts',(-0.132563224666591,-0.115389834088422,
1.02598037748835));
#30349=CARTESIAN_POINT('Ctrl Pts',(-0.153889680451665,-0.0645346507397467,
1.02227578113608));
#30350=CARTESIAN_POINT('Ctrl Pts',(-0.175216136236738,-0.0136794673910717,
1.01857118478382));
#30351=CARTESIAN_POINT('Ctrl Pts',(-0.16884041024437,0.0487928090797828,
1.01486658843155));
#30352=CARTESIAN_POINT('Ctrl Pts',(-0.137680389518285,0.0942913851820011,
1.01116199207928));
#30353=CARTESIAN_POINT('Ctrl Pts',(-0.106520368792199,0.139789961284219,
1.00745739572701));
#30354=CARTESIAN_POINT('Ctrl Pts',(-0.0505760533323975,0.168314837017802,
1.00375279937474));
#30355=CARTESIAN_POINT('Ctrl Pts',(0.00454932345543924,0.166811444936069,
1.00004820302248));
#30356=CARTESIAN_POINT('Ctrl Pts',(0.0596747002432758,0.165308052854335,
0.996343606670208));
#30357=CARTESIAN_POINT('Ctrl Pts',(0.113981138359147,0.133776392957287,
0.992639010317939));
#30358=CARTESIAN_POINT('Ctrl Pts',(0.142614988862282,0.0866471011481969,
0.988934413965671));
#30359=CARTESIAN_POINT('Ctrl Pts',(0.158285969463688,0.0608537759501981,
0.986906930530773));
#30360=CARTESIAN_POINT('Ctrl Pts',(0.166267372459907,0.0303885726052033,
0.984879447095876));
#30361=CARTESIAN_POINT('Ctrl Pts',(0.16633703813182,-4.26131537097363E-5,
0.982851963660979));
#30362=CARTESIAN_POINT('Origin',(0.,0.,1.3));
#30363=CARTESIAN_POINT('',(0.166729862742343,-0.000130123946020723,0.912851963660979));
#30364=CARTESIAN_POINT('',(0.16681765906064,8.64047405809373E-5,0.93214803633902));
#30365=CARTESIAN_POINT('',(0.1666,2.04026156737949E-17,1.3));
#30366=CARTESIAN_POINT('Ctrl Pts',(0.16681765906064,8.64047405809373E-5,
0.93214803633902));
#30367=CARTESIAN_POINT('Ctrl Pts',(0.166849023174239,0.00505533653555562,
0.932481542586184));
#30368=CARTESIAN_POINT('Ctrl Pts',(0.166646252238729,0.0100216728157887,
0.932815048833348));
#30369=CARTESIAN_POINT('Ctrl Pts',(0.166201007638075,0.0149661744225974,
0.933148555080512));
#30370=CARTESIAN_POINT('Ctrl Pts',(0.161255218653678,0.0698898310921401,
0.93685315143278));
#30371=CARTESIAN_POINT('Ctrl Pts',(0.126391025843356,0.122119345383236,
0.940557747785048));
#30372=CARTESIAN_POINT('Ctrl Pts',(0.0775642504900456,0.147751626038697,
0.944262344137316));
#30373=CARTESIAN_POINT('Ctrl Pts',(0.0287374751367354,0.173383906694158,
0.947966940489584));
#30374=CARTESIAN_POINT('Ctrl Pts',(-0.0340518827595631,0.172418953713984,
0.951671536841852));
#30375=CARTESIAN_POINT('Ctrl Pts',(-0.0820679309643883,0.145298361306226,
0.95537613319412));
#30376=CARTESIAN_POINT('Ctrl Pts',(-0.130083979169214,0.118177768898468,
0.959080729546388));
#30377=CARTESIAN_POINT('Ctrl Pts',(-0.163326717682566,0.0649015370631265,
0.962785325898656));
#30378=CARTESIAN_POINT('Ctrl Pts',(-0.166582411702781,0.00985184688226562,
0.966489922250924));
#30379=CARTESIAN_POINT('Ctrl Pts',(-0.169838105722997,-0.045197843298595,
0.970194518603192));
#30380=CARTESIAN_POINT('Ctrl Pts',(-0.143106755250076,-0.102020991824975,
0.97389911495546));
#30381=CARTESIAN_POINT('Ctrl Pts',(-0.0986221180718627,-0.134612168562546,
0.977603711307728));
#30382=CARTESIAN_POINT('Ctrl Pts',(-0.054137480893649,-0.167203345300117,
0.981308307659997));
#30383=CARTESIAN_POINT('Ctrl Pts',(0.00810044298985758,-0.175562550248879,
0.985012904012265));
#30384=CARTESIAN_POINT('Ctrl Pts',(0.0596081167151753,-0.155864142731977,
0.988717500364533));
#30385=CARTESIAN_POINT('Ctrl Pts',(0.111115790440493,-0.136165735215075,
0.992422096716801));
#30386=CARTESIAN_POINT('Ctrl Pts',(0.151893214007622,-0.0884097152325082,
0.996126693069068));
#30387=CARTESIAN_POINT('Ctrl Pts',(0.163278367297414,-0.0344518977599609,
0.999831289421336));
#30388=CARTESIAN_POINT('Ctrl Pts',(0.165651681983942,-0.0232040140116242,
1.0006035383939));
#30389=CARTESIAN_POINT('Ctrl Pts',(0.166747775756401,-0.0116866354136458,
1.00137578736646));
#30390=CARTESIAN_POINT('Ctrl Pts',(0.166641299058679,-0.000149160109009599,
1.00214803633902));
#30391=CARTESIAN_POINT('Ctrl Pts',(0.16633703813182,-4.26131537097363E-5,
0.982851963660979));
#30392=CARTESIAN_POINT('Ctrl Pts',(0.166394664840996,-0.0252149691141755,
0.981174850743608));
#30393=CARTESIAN_POINT('Ctrl Pts',(0.161038745460081,-0.0503640488000913,
0.979497737826238));
#30394=CARTESIAN_POINT('Ctrl Pts',(0.150143538011669,-0.0728263241997442,
0.977820624908867));
#30395=CARTESIAN_POINT('Ctrl Pts',(0.126076973767522,-0.122443534017465,
0.974116028556599));
#30396=CARTESIAN_POINT('Ctrl Pts',(0.0749825823888285,-0.158951029931774,
0.970411432204331));
#30397=CARTESIAN_POINT('Ctrl Pts',(0.0202440032863241,-0.165640975250716,
0.966706835852062));
#30398=CARTESIAN_POINT('Ctrl Pts',(-0.0344945758161804,-0.172330920569658,
0.963002239499794));
#30399=CARTESIAN_POINT('Ctrl Pts',(-0.0928773426424964,-0.149203315293232,
0.959297643147526));
#30400=CARTESIAN_POINT('Ctrl Pts',(-0.128185095718787,-0.106842589675449,
0.955593046795258));
#30401=CARTESIAN_POINT('Ctrl Pts',(-0.163492848795077,-0.064481864057666,
0.95188845044299));
#30402=CARTESIAN_POINT('Ctrl Pts',(-0.175725588121342,-0.00288801809852563,
0.948183854090722));
#30403=CARTESIAN_POINT('Ctrl Pts',(-0.159284925787188,0.0497500806758803,
0.944479257738454));
#30404=CARTESIAN_POINT('Ctrl Pts',(-0.142844263453034,0.102388179450286,
0.940774661386186));
#30405=CARTESIAN_POINT('Ctrl Pts',(-0.097730199458461,0.146070531039958,
0.937070065033918));
#30406=CARTESIAN_POINT('Ctrl Pts',(-0.0445894513306832,0.160805840780395,
0.93336546868165));
#30407=CARTESIAN_POINT('Ctrl Pts',(0.00855129679709463,0.175541150520831,
0.929660872329382));
#30408=CARTESIAN_POINT('Ctrl Pts',(0.0697187290580771,0.161329418412033,
0.925956275977114));
#30409=CARTESIAN_POINT('Ctrl Pts',(0.110919243004777,0.124674377251528,
0.922251679624846));
#30410=CARTESIAN_POINT('Ctrl Pts',(0.145765426127824,0.093672621343478,
0.919118440970224));
#30411=CARTESIAN_POINT('Ctrl Pts',(0.16632871557528,0.0466165403829395,
0.915985202315602));
#30412=CARTESIAN_POINT('Ctrl Pts',(0.166729862742343,-0.000130123946020723,
0.912851963660979));
#30413=CARTESIAN_POINT('Origin',(0.,0.,1.3));
#30414=CARTESIAN_POINT('',(0.166745353727506,0.000120148921586877,0.842851963660979));
#30415=CARTESIAN_POINT('',(0.166381444272219,9.40568719243839E-5,0.86214803633902));
#30416=CARTESIAN_POINT('',(0.1666,2.04026156737949E-17,1.3));
#30417=CARTESIAN_POINT('',(-0.126907087985236,0.107935865304853,0.8));
#30418=CARTESIAN_POINT('Ctrl Pts',(0.166745353727506,0.000120148921586877,
0.842851963660979));
#30419=CARTESIAN_POINT('Ctrl Pts',(0.166350216338014,-0.0471541035618327,
0.83968176483079));
#30420=CARTESIAN_POINT('Ctrl Pts',(0.14523873930488,-0.0947247812496833,
0.836511566000602));
#30421=CARTESIAN_POINT('Ctrl Pts',(0.109671969299941,-0.125754000901643,
0.833341367170413));
#30422=CARTESIAN_POINT('Ctrl Pts',(0.0681097413514803,-0.162013787777386,
0.829636770818145));
#30423=CARTESIAN_POINT('Ctrl Pts',(0.00680803444401046,-0.175685325249421,
0.825932174465876));
#30424=CARTESIAN_POINT('Ctrl Pts',(-0.0461862781086293,-0.160386912096395,
0.822227578113608));
#30425=CARTESIAN_POINT('Ctrl Pts',(-0.0991805906612692,-0.14508849894337,
0.81852298176134));
#30426=CARTESIAN_POINT('Ctrl Pts',(-0.143867508859079,-0.100820135165284,
0.814818385409072));
#30427=CARTESIAN_POINT('Ctrl Pts',(-0.159771943968926,-0.0481139506034528,
0.811113789056804));
#30428=CARTESIAN_POINT('Ctrl Pts',(-0.175676379078773,0.00459223395837816,
0.807409192704537));
#30429=CARTESIAN_POINT('Ctrl Pts',(-0.162798331100657,0.0657362393039545,
0.803704596352268));
#30430=CARTESIAN_POINT('Ctrl Pts',(-0.126907087985236,0.107935865304854,
0.8));
#30431=CARTESIAN_POINT('',(0.127144529223414,0.10812516429919,0.8));
#30432=CARTESIAN_POINT('Origin',(0.,0.,0.8));
#30433=CARTESIAN_POINT('Ctrl Pts',(0.127144588893496,0.108125211870903,
0.8));
#30434=CARTESIAN_POINT('Ctrl Pts',(0.0920578520263333,0.149281442964014,
0.803632291818556));
#30435=CARTESIAN_POINT('Ctrl Pts',(0.0350626176413565,0.171873117908773,
0.807264583637111));
#30436=CARTESIAN_POINT('Ctrl Pts',(-0.0186760721562392,0.165810809841732,
0.810896875455666));
#30437=CARTESIAN_POINT('Ctrl Pts',(-0.0734844862772781,0.159627825248711,
0.814601471807934));
#30438=CARTESIAN_POINT('Ctrl Pts',(-0.124905415613006,0.123638729028309,
0.818306068160202));
#30439=CARTESIAN_POINT('Ctrl Pts',(-0.14943866399484,0.0742601129650432,
0.82201066451247));
#30440=CARTESIAN_POINT('Ctrl Pts',(-0.173971912376674,0.0248814969017771,
0.825715260864738));
#30441=CARTESIAN_POINT('Ctrl Pts',(-0.171617479804614,-0.0378866390043534,
0.829419857217006));
#30442=CARTESIAN_POINT('Ctrl Pts',(-0.143435789399569,-0.0852901107552215,
0.833124453569274));
#30443=CARTESIAN_POINT('Ctrl Pts',(-0.115254098994523,-0.132693582506089,
0.836829049921542));
#30444=CARTESIAN_POINT('Ctrl Pts',(-0.0612451507564931,-0.164732390101695,
0.84053364627381));
#30445=CARTESIAN_POINT('Ctrl Pts',(-0.00613536544337925,-0.166758384009028,
0.844238242626078));
#30446=CARTESIAN_POINT('Ctrl Pts',(0.0489744198697346,-0.168784377916361,
0.847942838978346));
#30447=CARTESIAN_POINT('Ctrl Pts',(0.105185042257932,-0.140797558135422,
0.851647435330614));
#30448=CARTESIAN_POINT('Ctrl Pts',(0.136776048425978,-0.0955986339274043,
0.855352031682883));
#30449=CARTESIAN_POINT('Ctrl Pts',(0.156093728823978,-0.0679598063592257,
0.857617366568262));
#30450=CARTESIAN_POINT('Ctrl Pts',(0.166205550297931,-0.0338849643656092,
0.859882701453641));
#30451=CARTESIAN_POINT('Ctrl Pts',(0.166381444272219,9.40568719243839E-5,
0.86214803633902));
#30452=CARTESIAN_POINT('Origin',(0.,0.,0.645407471946233));
#30453=CARTESIAN_POINT('',(0.205717919156333,0.000119231682504745,1.65459252805377));
#30454=CARTESIAN_POINT('',(0.20515534870289,-8.10795385496472E-5,1.66040747194623));
#30455=CARTESIAN_POINT('',(0.205475,1.17874941047504E-14,0.645407471946233));
#30456=CARTESIAN_POINT('',(-0.188262750966373,-0.0823232180103128,1.7));
#30457=CARTESIAN_POINT('Ctrl Pts',(0.20515534870289,-8.1079538549661E-5,
1.66040747194623));
#30458=CARTESIAN_POINT('Ctrl Pts',(0.205035475209089,0.0384765991859779,
1.66249119224068));
#30459=CARTESIAN_POINT('Ctrl Pts',(0.176046579400947,0.14575433740106,1.6682795088874));
#30460=CARTESIAN_POINT('Ctrl Pts',(0.00300247275662535,0.243001989931863,
1.67777242188639));
#30461=CARTESIAN_POINT('Ctrl Pts',(-0.202554499717183,0.133854462473394,
1.6888862109432));
#30462=CARTESIAN_POINT('Ctrl Pts',(-0.215637179506013,-0.0197213743559566,
1.69629540364773));
#30463=CARTESIAN_POINT('Ctrl Pts',(-0.188262750966373,-0.0823232180103128,
1.7));
#30464=CARTESIAN_POINT('',(-0.122364587709818,-0.165532040449643,1.7));
#30465=CARTESIAN_POINT('Origin',(0.,0.,1.7));
#30466=CARTESIAN_POINT('Ctrl Pts',(0.205717919156333,0.000119231682504748,
1.65459252805377));
#30467=CARTESIAN_POINT('Ctrl Pts',(0.205768208325854,0.00728313946640584,
1.65498227116049));
#30468=CARTESIAN_POINT('Ctrl Pts',(0.202179510783538,0.0824912465572326,
1.65907661061947));
#30469=CARTESIAN_POINT('Ctrl Pts',(0.109634140470589,0.216730418270261,
1.66687554643072));
#30470=CARTESIAN_POINT('Ctrl Pts',(-0.122663843019391,0.209602590285094,
1.67798933548753));
#30471=CARTESIAN_POINT('Ctrl Pts',(-0.24177601945125,0.0120092944511596,
1.68903082001062));
#30472=CARTESIAN_POINT('Ctrl Pts',(-0.175954082167323,-0.125816077227026,
1.69636770818144));
#30473=CARTESIAN_POINT('Ctrl Pts',(-0.122364641233049,-0.165532117868825,
1.7));
#30474=CARTESIAN_POINT('Origin',(0.,0.,0.645407471946233));
#30475=CARTESIAN_POINT('',(0.2051889883028,0.000102640746213675,1.58459252805377));
#30476=CARTESIAN_POINT('',(0.205663604651154,-0.000149728163284854,1.59040747194623));
#30477=CARTESIAN_POINT('',(0.205475,1.17874941047504E-14,0.645407471946233));
#30478=CARTESIAN_POINT('Ctrl Pts',(0.205663604651154,-0.000149728163284867,
1.59040747194623));
#30479=CARTESIAN_POINT('Ctrl Pts',(0.205182444335985,0.0585183956951034,
1.59359694746041));
#30480=CARTESIAN_POINT('Ctrl Pts',(0.148135327616145,0.186146531383155,
1.60049101932685));
#30481=CARTESIAN_POINT('Ctrl Pts',(-0.0684290720584363,0.233024356666725,
1.61108968754557));
#30482=CARTESIAN_POINT('Ctrl Pts',(-0.23288917800895,0.0688795811193509,
1.62220347660237));
#30483=CARTESIAN_POINT('Ctrl Pts',(-0.184175405168835,-0.158290127824162,
1.63331726565918));
#30484=CARTESIAN_POINT('Ctrl Pts',(0.0331013206128567,-0.240615925517378,
1.64443105471598));
#30485=CARTESIAN_POINT('Ctrl Pts',(0.185046630854554,-0.128496885183325,
1.65346112347833));
#30486=CARTESIAN_POINT('Ctrl Pts',(0.205248595419634,-0.0300741733602017,
1.65878659588842));
#30487=CARTESIAN_POINT('Ctrl Pts',(0.20515534870289,-8.1079538549661E-5,
1.66040747194623));
#30488=CARTESIAN_POINT('Ctrl Pts',(0.2051889883028,0.000102640746213654,
1.58459252805377));
#30489=CARTESIAN_POINT('Ctrl Pts',(0.205314142408481,0.0277738688435417,
1.58608802638021));
#30490=CARTESIAN_POINT('Ctrl Pts',(0.187212802641802,0.123834372120327,
1.59128812105892));
#30491=CARTESIAN_POINT('Ctrl Pts',(0.041212233239435,0.2393392912824,1.6001928120899));
#30492=CARTESIAN_POINT('Ctrl Pts',(-0.178731921787321,0.164428017156146,
1.6113066011467));
#30493=CARTESIAN_POINT('Ctrl Pts',(-0.235078089364662,-0.0609842187918821,
1.62242039020351));
#30494=CARTESIAN_POINT('Ctrl Pts',(-0.0762596568913861,-0.230580482955351,
1.63353417926032));
#30495=CARTESIAN_POINT('Ctrl Pts',(0.144352083897931,-0.190571029763675,
1.6442582252104));
#30496=CARTESIAN_POINT('Ctrl Pts',(0.205290198398921,-0.0608114238158697,
1.65127767480822));
#30497=CARTESIAN_POINT('Ctrl Pts',(0.205717919156333,0.000119231682504748,
1.65459252805377));
#30498=CARTESIAN_POINT('Origin',(0.,0.,0.645407471946233));
#30499=CARTESIAN_POINT('',(0.205346259354759,-0.00017652456807675,1.51459252805377));
#30500=CARTESIAN_POINT('',(0.205625119184624,0.000163390229490382,1.52040747194623));
#30501=CARTESIAN_POINT('',(0.205475,1.17874941047504E-14,0.645407471946233));
#30502=CARTESIAN_POINT('Ctrl Pts',(0.205625119184624,0.000163390229490371,
1.52040747194623));
#30503=CARTESIAN_POINT('Ctrl Pts',(0.205719589271595,0.0110330279545173,
1.52099810632787));
#30504=CARTESIAN_POINT('Ctrl Pts',(0.199992588366042,0.0899798330776656,
1.52529333706177));
#30505=CARTESIAN_POINT('Ctrl Pts',(0.0977367556084749,0.222326520064881,
1.53329316414794));
#30506=CARTESIAN_POINT('Ctrl Pts',(-0.133782052044684,0.202691772286445,
1.54440695320474));
#30507=CARTESIAN_POINT('Ctrl Pts',(-0.242848712699985,-0.00246927953082339,
1.55552074226155));
#30508=CARTESIAN_POINT('Ctrl Pts',(-0.129633034711377,-0.205369738746763,
1.56663453131835));
#30509=CARTESIAN_POINT('Ctrl Pts',(0.102236927935064,-0.220293776124516,
1.57774832037515));
#30510=CARTESIAN_POINT('Ctrl Pts',(0.20084133199376,-0.0871629660671419,
1.58567263391778));
#30511=CARTESIAN_POINT('Ctrl Pts',(0.205741315141077,-0.00962500803198312,
1.58989235110814));
#30512=CARTESIAN_POINT('Ctrl Pts',(0.205663604651154,-0.000149728163284867,
1.59040747194623));
#30513=CARTESIAN_POINT('Ctrl Pts',(0.205346259354759,-0.000176524568076758,
1.51459252805377));
#30514=CARTESIAN_POINT('Ctrl Pts',(0.204952685935524,0.0478618563462208,
1.51719378159994));
#30515=CARTESIAN_POINT('Ctrl Pts',(0.164184854806731,0.1649162911311,1.52349963149837));
#30516=CARTESIAN_POINT('Ctrl Pts',(-0.0308180903310451,0.240897960470908,
1.53351007774908));
#30517=CARTESIAN_POINT('Ctrl Pts',(-0.219105973246366,0.104757609325286,
1.54462386680588));
#30518=CARTESIAN_POINT('Ctrl Pts',(-0.206843620635952,-0.127268531807556,
1.55573765586268));
#30519=CARTESIAN_POINT('Ctrl Pts',(-0.00525505851706014,-0.242804414954791,
1.56685144491949));
#30520=CARTESIAN_POINT('Ctrl Pts',(0.173370196153793,-0.15045712725832,
1.57646973564985));
#30521=CARTESIAN_POINT('Ctrl Pts',(0.20500411501816,-0.0407723333551383,
1.58238343002794));
#30522=CARTESIAN_POINT('Ctrl Pts',(0.2051889883028,0.000102640746213654,
1.58459252805377));
#30523=CARTESIAN_POINT('Origin',(0.,0.,0.645407471946233));
#30524=CARTESIAN_POINT('',(0.205812292792875,8.2771271442428E-7,1.44459252805377));
#30525=CARTESIAN_POINT('',(0.20514810115636,4.68968264668604E-5,1.45040747194623));
#30526=CARTESIAN_POINT('',(0.205475,1.17874941047504E-14,0.645407471946233));
#30527=CARTESIAN_POINT('Ctrl Pts',(0.20514810115636,4.68968264668648E-5,
1.45040747194623));
#30528=CARTESIAN_POINT('Ctrl Pts',(0.205212209277079,0.0314508805486537,
1.45210386154759));
#30529=CARTESIAN_POINT('Ctrl Pts',(0.183673234943095,0.131351887215635,
1.45750484750122));
#30530=CARTESIAN_POINT('Ctrl Pts',(0.028210615278035,0.241217190661839,
1.46661042980711));
#30531=CARTESIAN_POINT('Ctrl Pts',(-0.187360277963068,0.154524103926572,
1.47772421886392));
#30532=CARTESIAN_POINT('Ctrl Pts',(-0.23143818564818,-0.0736066521476796,
1.48883800792072));
#30533=CARTESIAN_POINT('Ctrl Pts',(-0.0636780941176189,-0.234364395962394,
1.49995179697753));
#30534=CARTESIAN_POINT('Ctrl Pts',(0.15035425339619,-0.183462731047792,
1.51047495165269));
#30535=CARTESIAN_POINT('Ctrl Pts',(0.205127050891722,-0.0571438705105598,
1.5172935099756));
#30536=CARTESIAN_POINT('Ctrl Pts',(0.205625119184624,0.000163390229490371,
1.52040747194623));
#30537=CARTESIAN_POINT('Ctrl Pts',(0.205812290976358,8.27708256686491E-7,
1.44459252805377));
#30538=CARTESIAN_POINT('Ctrl Pts',(0.205812293621698,4.5117938930396E-5,
1.44459494046739));
#30539=CARTESIAN_POINT('Ctrl Pts',(0.205792223959932,0.0681032095145843,
1.44830194923329));
#30540=CARTESIAN_POINT('Ctrl Pts',(0.13158183823911,0.204126920402922,1.45571355435144));
#30541=CARTESIAN_POINT('Ctrl Pts',(-0.10013585656473,0.221256389923926,
1.46682734340825));
#30542=CARTESIAN_POINT('Ctrl Pts',(-0.240198066802314,0.0358673761285168,
1.47794113246505));
#30543=CARTESIAN_POINT('Ctrl Pts',(-0.160404261381875,-0.182351453033287,
1.48905492152186));
#30544=CARTESIAN_POINT('Ctrl Pts',(0.0662093815164626,-0.233661930697804,
1.50016871057866));
#30545=CARTESIAN_POINT('Ctrl Pts',(0.193364787149743,-0.109147888339539,
1.5086812460893));
#30546=CARTESIAN_POINT('Ctrl Pts',(0.20551319671518,-0.0205523937625982,
1.51348918524767));
#30547=CARTESIAN_POINT('Ctrl Pts',(0.205346259354759,-0.000176524568076758,
1.51459252805377));
#30548=CARTESIAN_POINT('Origin',(0.,0.,0.645407471946233));
#30549=CARTESIAN_POINT('',(0.205343844683429,0.000176004178461642,1.37459252805377));
#30550=CARTESIAN_POINT('',(0.205453133831238,-0.000187888241826064,1.38040747194623));
#30551=CARTESIAN_POINT('',(0.205475,1.17874941047504E-14,0.645407471946233));
#30552=CARTESIAN_POINT('Ctrl Pts',(0.205453133831238,-0.000187888241826079,
1.38040747194623));
#30553=CARTESIAN_POINT('Ctrl Pts',(0.204982640394683,0.0514920396676331,
1.38320961676732));
#30554=CARTESIAN_POINT('Ctrl Pts',(0.159017805479884,0.172241441932577,
1.38971635794067));
#30555=CARTESIAN_POINT('Ctrl Pts',(-0.0437982449057285,0.238879228826581,
1.39992769546629));
#30556=CARTESIAN_POINT('Ctrl Pts',(-0.224449621610114,0.0927574233548304,
1.41104148452309));
#30557=CARTESIAN_POINT('Ctrl Pts',(-0.199659714256911,-0.13826630374757,
1.42215527357989));
#30558=CARTESIAN_POINT('Ctrl Pts',(0.00788099391586731,-0.242733314804761,
1.4332690626367));
#30559=CARTESIAN_POINT('Ctrl Pts',(0.177630548818419,-0.142990752308629,
1.44268646209214));
#30560=CARTESIAN_POINT('Ctrl Pts',(0.205072209179237,-0.037129523063069,
1.44839926519532));
#30561=CARTESIAN_POINT('Ctrl Pts',(0.20514810115636,4.68968264668648E-5,
1.45040747194623));
#30562=CARTESIAN_POINT('Ctrl Pts',(0.205343844683429,0.000176004178461609,
1.37459252805377));
#30563=CARTESIAN_POINT('Ctrl Pts',(0.2055108740339,0.0206415845782027,1.37570069568712));
#30564=CARTESIAN_POINT('Ctrl Pts',(0.193294976926761,0.109328542053589,
1.38051345967274));
#30565=CARTESIAN_POINT('Ctrl Pts',(0.0659057470887793,0.233747753644337,
1.38903082001062));
#30566=CARTESIAN_POINT('Ctrl Pts',(-0.160641042350602,0.182142898149225,
1.40014460906743));
#30567=CARTESIAN_POINT('Ctrl Pts',(-0.240151263944613,-0.0361794176709605,
1.41125839812423));
#30568=CARTESIAN_POINT('Ctrl Pts',(-0.0998483101275995,-0.221386302178844,
1.42237218718103));
#30569=CARTESIAN_POINT('Ctrl Pts',(0.131796641356581,-0.203959577192589,
1.43348356382421));
#30570=CARTESIAN_POINT('Ctrl Pts',(0.205808231334455,-0.0679686858761153,
1.44089034411512));
#30571=CARTESIAN_POINT('Ctrl Pts',(0.205812290976358,8.27708256686491E-7,
1.44459252805377));
#30572=CARTESIAN_POINT('Origin',(0.,0.,0.645407471946233));
#30573=CARTESIAN_POINT('',(0.205190393281102,-0.000103909026722956,1.30459252805377));
#30574=CARTESIAN_POINT('',(0.205784930460293,6.78762012092915E-5,1.31040747194623));
#30575=CARTESIAN_POINT('',(0.205475,1.17874941047504E-14,0.645407471946233));
#30576=CARTESIAN_POINT('Ctrl Pts',(0.205784930460293,6.78762012092937E-5,
1.31040747194623));
#30577=CARTESIAN_POINT('Ctrl Pts',(0.205801002271222,0.00380171834571078,
1.31061077563477));
#30578=CARTESIAN_POINT('Ctrl Pts',(0.204016743590097,0.0755578983061786,
1.31451867567558));
#30579=CARTESIAN_POINT('Ctrl Pts',(0.120352309668968,0.210942868533614,
1.32213117206866));
#30580=CARTESIAN_POINT('Ctrl Pts',(-0.111952589707427,0.215518421220722,
1.33324496112546));
#30581=CARTESIAN_POINT('Ctrl Pts',(-0.241786014095534,0.0228275188203595,
1.34435875018226));
#30582=CARTESIAN_POINT('Ctrl Pts',(-0.150309957742793,-0.190757670439842,
1.35547253923907));
#30583=CARTESIAN_POINT('Ctrl Pts',(0.0787465075641072,-0.229740200603712,
1.36658632829588));
#30584=CARTESIAN_POINT('Ctrl Pts',(0.196145957186436,-0.101629499882189,
1.37489797253159));
#30585=CARTESIAN_POINT('Ctrl Pts',(0.205604659733481,-0.0168317924834936,
1.37950502041505));
#30586=CARTESIAN_POINT('Ctrl Pts',(0.205453133831238,-0.000187888241826079,
1.38040747194623));
#30587=CARTESIAN_POINT('Ctrl Pts',(0.205190393281102,-0.000103909026722949,
1.30459252805377));
#30588=CARTESIAN_POINT('Ctrl Pts',(0.205002798510851,0.0408596785255145,
1.30680645090684));
#30589=CARTESIAN_POINT('Ctrl Pts',(0.173264151191812,0.15063609956695,1.31272497011219));
#30590=CARTESIAN_POINT('Ctrl Pts',(-0.00557045627447471,0.242797343170749,
1.3223480856698));
#30591=CARTESIAN_POINT('Ctrl Pts',(-0.207008825709279,0.126999708315969,
1.3334618747266));
#30592=CARTESIAN_POINT('Ctrl Pts',(-0.218969669332857,-0.105042199835232,
1.3445756637834));
#30593=CARTESIAN_POINT('Ctrl Pts',(-0.0305050913306782,-0.240937791217362,
1.35568945284021));
#30594=CARTESIAN_POINT('Ctrl Pts',(0.164305043004325,-0.164739584440547,
1.36569507426366));
#30595=CARTESIAN_POINT('Ctrl Pts',(0.204952496128017,-0.0477747021046654,
1.37199609933485));
#30596=CARTESIAN_POINT('Ctrl Pts',(0.205343844683429,0.000176004178461609,
1.37459252805377));
#30597=CARTESIAN_POINT('Origin',(0.,0.,0.645407471946233));
#30598=CARTESIAN_POINT('',(0.205723053630104,-0.00012021653370823,1.23459252805377));
#30599=CARTESIAN_POINT('',(0.2052527421894,0.000145096082381024,1.24040747194623));
#30600=CARTESIAN_POINT('',(0.205475,1.17874941047504E-14,0.645407471946233));
#30601=CARTESIAN_POINT('Ctrl Pts',(0.2052527421894,0.000145096082381054,
1.24040747194623));
#30602=CARTESIAN_POINT('Ctrl Pts',(0.205410551512377,0.0243477880181972,
1.2417165308545));
#30603=CARTESIAN_POINT('Ctrl Pts',(0.19025975845005,0.116852155262949,1.24673018611503));
#30604=CARTESIAN_POINT('Ctrl Pts',(0.053170711887795,0.236969296798376,
1.25544843772783));
#30605=CARTESIAN_POINT('Ctrl Pts',(-0.170254416296827,0.17319066360285,
1.26656222678464));
#30606=CARTESIAN_POINT('Ctrl Pts',(-0.237843746428552,-0.0491113481040567,
1.27767601584144));
#30607=CARTESIAN_POINT('Ctrl Pts',(-0.0877319981226961,-0.226461185930791,
1.28878980489824));
#30608=CARTESIAN_POINT('Ctrl Pts',(0.138466900336863,-0.197076087766382,
1.29970029026651));
#30609=CARTESIAN_POINT('Ctrl Pts',(0.205508142006035,-0.0642362896597867,
1.3069061792825));
#30610=CARTESIAN_POINT('Ctrl Pts',(0.205784930460293,6.78762012092937E-5,
1.31040747194623));
#30611=CARTESIAN_POINT('Ctrl Pts',(0.205723053630104,-0.000120216533708221,
1.23459252805377));
#30612=CARTESIAN_POINT('Ctrl Pts',(0.205298918797858,0.0608969853087639,
1.23791220612657));
#30613=CARTESIAN_POINT('Ctrl Pts',(0.144198668474879,0.190744063350028,
1.24493648055164));
#30614=CARTESIAN_POINT('Ctrl Pts',(-0.0765564251386213,0.230479269358191,
1.25566535132897));
#30615=CARTESIAN_POINT('Ctrl Pts',(-0.23515855594305,0.0606797610465845,
1.26677914038578));
#30616=CARTESIAN_POINT('Ctrl Pts',(-0.178517393613401,-0.164660620706261,
1.27789292944258));
#30617=CARTESIAN_POINT('Ctrl Pts',(0.0415227636155418,-0.239285268948212,
1.28900671849938));
#30618=CARTESIAN_POINT('Ctrl Pts',(0.187294592944535,-0.123653783093607,
1.29790658470311));
#30619=CARTESIAN_POINT('Ctrl Pts',(0.205316704165066,-0.0276854186132918,
1.30310185455457));
#30620=CARTESIAN_POINT('Ctrl Pts',(0.205190393281102,-0.000103909026722949,
1.30459252805377));
#30621=CARTESIAN_POINT('Origin',(0.,0.,0.645407471946233));
#30622=CARTESIAN_POINT('',(0.205554604385647,0.000179910838621594,1.16459252805377));
#30623=CARTESIAN_POINT('',(0.205260574591088,-0.000148793951100861,1.17040747194623));
#30624=CARTESIAN_POINT('',(0.205475,1.17874941047504E-14,0.645407471946233));
#30625=CARTESIAN_POINT('Ctrl Pts',(0.205260574591088,-0.000148793951100864,
1.17040747194623));
#30626=CARTESIAN_POINT('Ctrl Pts',(0.204961311968991,0.044493502374408,
1.17282228607422));
#30627=CARTESIAN_POINT('Ctrl Pts',(0.168697767785137,0.158064764697474,
1.17894169655448));
#30628=CARTESIAN_POINT('Ctrl Pts',(-0.0186902364010947,0.242140965743205,
1.18876570338701));
#30629=CARTESIAN_POINT('Ctrl Pts',(-0.213572804428157,0.115621059658089,
1.19987949244381));
#30630=CARTESIAN_POINT('Ctrl Pts',(-0.212969762481792,-0.116728113564033,
1.21099328150062));
#30631=CARTESIAN_POINT('Ctrl Pts',(-0.0174330816944656,-0.242234720654174,
1.22210707055742));
#30632=CARTESIAN_POINT('Ctrl Pts',(0.169149144270981,-0.157353841391122,
1.23191180070596));
#30633=CARTESIAN_POINT('Ctrl Pts',(0.204963955993594,-0.0441450839941835,
1.23801193450223));
#30634=CARTESIAN_POINT('Ctrl Pts',(0.2052527421894,0.000145096082381054,
1.24040747194623));
#30635=CARTESIAN_POINT('Ctrl Pts',(0.205554604385647,0.00017991083862162,
1.16459252805377));
#30636=CARTESIAN_POINT('Ctrl Pts',(0.205676289601756,0.0134574818611262,
1.16531336499402));
#30637=CARTESIAN_POINT('Ctrl Pts',(0.198454332603713,0.094840644563722,
1.16973879828655));
#30638=CARTESIAN_POINT('Ctrl Pts',(0.0898833437085198,0.225615966539919,
1.17786882793134));
#30639=CARTESIAN_POINT('Ctrl Pts',(-0.140804956527845,0.197877598659039,
1.18898261698814));
#30640=CARTESIAN_POINT('Ctrl Pts',(-0.242612883217311,-0.0109803793588139,
1.20009640604495));
#30641=CARTESIAN_POINT('Ctrl Pts',(-0.12235448648082,-0.2097878916237,1.21121019510175));
#30642=CARTESIAN_POINT('Ctrl Pts',(0.109896359325859,-0.21657416752884,
1.22232398415856));
#30643=CARTESIAN_POINT('Ctrl Pts',(0.202230669468777,-0.082312541395209,
1.23011809514256));
#30644=CARTESIAN_POINT('Ctrl Pts',(0.20577223226921,-0.00719519062340044,
1.2342076097743));
#30645=CARTESIAN_POINT('Ctrl Pts',(0.205723053630104,-0.000120216533708221,
1.23459252805377));
#30646=CARTESIAN_POINT('Origin',(0.,0.,0.645407471946233));
#30647=CARTESIAN_POINT('',(0.205138522353965,7.81005524626288E-6,1.09459252805377));
#30648=CARTESIAN_POINT('',(0.205789655863746,-6.17368779781373E-5,1.10040747194623));
#30649=CARTESIAN_POINT('',(0.205475,1.17874941047504E-14,0.645407471946233));
#30650=CARTESIAN_POINT('Ctrl Pts',(0.205789655863746,-6.17368779781361E-5,
1.10040747194623));
#30651=CARTESIAN_POINT('Ctrl Pts',(0.205533723504375,0.0645925032691717,
1.10392804129395));
#30652=CARTESIAN_POINT('Ctrl Pts',(0.137841967409279,0.197742342810066,
1.11115320699393));
#30653=CARTESIAN_POINT('Ctrl Pts',(-0.0889063286388705,0.226002736612265,
1.12208296904618));
#30654=CARTESIAN_POINT('Ctrl Pts',(-0.238095468835566,0.0478760895194249,
1.13319675810299));
#30655=CARTESIAN_POINT('Ctrl Pts',(-0.169353126220915,-0.174072085260317,
1.14431054715979));
#30656=CARTESIAN_POINT('Ctrl Pts',(0.0544000534188783,-0.236690106290626,
1.1554243362166));
#30657=CARTESIAN_POINT('Ctrl Pts',(0.190562019135808,-0.116130140045317,
1.16412331114541));
#30658=CARTESIAN_POINT('Ctrl Pts',(0.2054204144752,-0.0239927989965278,
1.16911768972195));
#30659=CARTESIAN_POINT('Ctrl Pts',(0.205260574591088,-0.000148793951100864,
1.17040747194623));
#30660=CARTESIAN_POINT('Ctrl Pts',(0.205138522353965,7.81005524630105E-6,
1.09459252805377));
#30661=CARTESIAN_POINT('Ctrl Pts',(0.205149988139531,0.033826082896543,
1.09641912021375));
#30662=CARTESIAN_POINT('Ctrl Pts',(0.181232693643337,0.1362174972132,1.101950308726));
#30663=CARTESIAN_POINT('Ctrl Pts',(0.019737729131079,0.242057848222183,
1.11118609359052));
#30664=CARTESIAN_POINT('Ctrl Pts',(-0.192661783512051,0.147861479120299,
1.12229988264732));
#30665=CARTESIAN_POINT('Ctrl Pts',(-0.228715780766039,-0.0816741786716276,
1.13341367170413));
#30666=CARTESIAN_POINT('Ctrl Pts',(-0.0554236300753314,-0.236452534483491,
1.14452746076093));
#30667=CARTESIAN_POINT('Ctrl Pts',(0.15406839794226,-0.178801760545413,
1.15492041287748));
#30668=CARTESIAN_POINT('Ctrl Pts',(0.205050912928411,-0.0547799216762583,
1.16160876864176));
#30669=CARTESIAN_POINT('Ctrl Pts',(0.205554604385647,0.00017991083862162,
1.16459252805377));
#30670=CARTESIAN_POINT('Origin',(0.,0.,0.645407471946233));
#30671=CARTESIAN_POINT('',(0.20552593591886,-0.000183965626637278,1.02459252805377));
#30672=CARTESIAN_POINT('',(0.20544247508097,0.000187699708462681,1.03040747194623));
#30673=CARTESIAN_POINT('',(0.205475,1.17874941047504E-14,0.645407471946233));
#30674=CARTESIAN_POINT('Ctrl Pts',(0.20544247508097,0.000187699708462687,
1.03040747194623));
#30675=CARTESIAN_POINT('Ctrl Pts',(0.205596383177594,0.0171893738494543,
1.0313292001614));
#30676=CARTESIAN_POINT('Ctrl Pts',(0.195889593181661,0.102350581389175,
1.03595552472885));
#30677=CARTESIAN_POINT('Ctrl Pts',(0.0775529135379212,0.230145861972334,
1.04428644564855));
#30678=CARTESIAN_POINT('Ctrl Pts',(-0.151298115744515,0.18997487313149,
1.05540023470536));
#30679=CARTESIAN_POINT('Ctrl Pts',(-0.241664263837854,-0.0240822717379046,
1.06651402376216));
#30680=CARTESIAN_POINT('Ctrl Pts',(-0.110832370586897,-0.216096640074974,
1.07762781281897));
#30681=CARTESIAN_POINT('Ctrl Pts',(0.121445648389767,-0.210315303100593,
1.08874160187577));
#30682=CARTESIAN_POINT('Ctrl Pts',(0.204196124007957,-0.074841794914668,
1.09633482158486));
#30683=CARTESIAN_POINT('Ctrl Pts',(0.205803033945758,-0.00344133971228389,
1.10022344494168));
#30684=CARTESIAN_POINT('Ctrl Pts',(0.205789655863746,-6.17368779781361E-5,
1.10040747194623));
#30685=CARTESIAN_POINT('Ctrl Pts',(0.20552593591886,-0.000183965626637285,
1.02459252805377));
#30686=CARTESIAN_POINT('Ctrl Pts',(0.205027284976747,0.0538482597648122,
1.02752487543347));
#30687=CARTESIAN_POINT('Ctrl Pts',(0.155496650182077,0.176951247041673,
1.03416181916545));
#30688=CARTESIAN_POINT('Ctrl Pts',(-0.0521449271278155,0.237197146991165,
1.04450335924969));
#30689=CARTESIAN_POINT('Ctrl Pts',(-0.227563185653378,0.0848326375129703,
1.0556171483065));
#30690=CARTESIAN_POINT('Ctrl Pts',(-0.194690279246867,-0.145180146557101,
1.0667309373633));
#30691=CARTESIAN_POINT('Ctrl Pts',(0.0163848475034698,-0.242307896337387,
1.0778447264201));
#30692=CARTESIAN_POINT('Ctrl Pts',(0.180236614284166,-0.138136714556845,
1.08713192331693));
#30693=CARTESIAN_POINT('Ctrl Pts',(0.205126733847568,-0.0347623261378718,
1.09271452386148));
#30694=CARTESIAN_POINT('Ctrl Pts',(0.205138522353965,7.81005524630105E-6,
1.09459252805377));
#30695=CARTESIAN_POINT('Origin',(0.,0.,0.645407471946233));
#30696=CARTESIAN_POINT('',(0.205743448352251,0.000106566711118361,0.954592528053768));
#30697=CARTESIAN_POINT('',(0.205150677731907,-5.25566492129599E-5,0.960407471946232));
#30698=CARTESIAN_POINT('',(0.205475,1.17874941047504E-14,0.645407471946233));
#30699=CARTESIAN_POINT('Ctrl Pts',(0.205150677731907,-5.25566492129668E-5,
0.960407471946232));
#30700=CARTESIAN_POINT('Ctrl Pts',(0.205064756039612,0.0374795435537448,
0.962434955381129));
#30701=CARTESIAN_POINT('Ctrl Pts',(0.177234439623409,0.143708517228788,
0.968167035168295));
#30702=CARTESIAN_POINT('Ctrl Pts',(0.00662091032790181,0.242770948244842,
0.977603711307729));
#30703=CARTESIAN_POINT('Ctrl Pts',(-0.200374735874429,0.13722805194188,
0.988717500364533));
#30704=CARTESIAN_POINT('Ctrl Pts',(-0.223965113394512,-0.0939212459185429,
0.999831289421336));
#30705=CARTESIAN_POINT('Ctrl Pts',(-0.0425576829655005,-0.239103357370329,
1.01094507847814));
#30706=CARTESIAN_POINT('Ctrl Pts',(0.159527519870246,-0.171541476398135,
1.02113713931977));
#30707=CARTESIAN_POINT('Ctrl Pts',(0.204977798041595,-0.0511435023372491,
1.02762460380914));
#30708=CARTESIAN_POINT('Ctrl Pts',(0.20544247508097,0.000187699708462687,
1.03040747194623));
#30709=CARTESIAN_POINT('Ctrl Pts',(0.205743448352251,0.000106566711118368,
0.954592528053768));
#30710=CARTESIAN_POINT('Ctrl Pts',(0.205782131072789,0.00623496563411944,
0.954926034300931));
#30711=CARTESIAN_POINT('Ctrl Pts',(0.202754080859383,0.0803990246761448,
0.958964136900363));
#30712=CARTESIAN_POINT('Ctrl Pts',(0.112884009708659,0.215032004451281,
0.966706835852063));
#30713=CARTESIAN_POINT('Ctrl Pts',(-0.119438498942156,0.211461649464463,
0.977820624908867));
#30714=CARTESIAN_POINT('Ctrl Pts',(-0.242437629122786,0.0143379927471741,
0.988934413965671));
#30715=CARTESIAN_POINT('Ctrl Pts',(-0.143530830111561,-0.195909362177039,
1.00004820302247));
#30716=CARTESIAN_POINT('Ctrl Pts',(0.086751356142284,-0.226838671363958,
1.01116199207928));
#30717=CARTESIAN_POINT('Ctrl Pts',(0.19782031948766,-0.0967615068704032,
1.01934343375638));
#30718=CARTESIAN_POINT('Ctrl Pts',(0.205657258244577,-0.0144136339232786,
1.02382027908121));
#30719=CARTESIAN_POINT('Ctrl Pts',(0.20552593591886,-0.000183965626637285,
1.02459252805377));
#30720=CARTESIAN_POINT('Origin',(0.,0.,0.645407471946233));
#30721=CARTESIAN_POINT('',(0.205205445749305,0.000116004416325019,0.884592528053768));
#30722=CARTESIAN_POINT('',(0.205635165348036,-0.000160487501855341,0.890407471946233));
#30723=CARTESIAN_POINT('',(0.205475,1.17874941047504E-14,0.645407471946233));
#30724=CARTESIAN_POINT('Ctrl Pts',(0.205635165348036,-0.000160487501855345,
0.890407471946233));
#30725=CARTESIAN_POINT('Ctrl Pts',(0.20514041316225,0.0574941994909011,
0.893540710600855));
#30726=CARTESIAN_POINT('Ctrl Pts',(0.149792439928844,0.184149942781777,
0.900378545607745));
#30727=CARTESIAN_POINT('Ctrl Pts',(-0.0648937601106981,0.234030453531351,
0.910920976966904));
#30728=CARTESIAN_POINT('Ctrl Pts',(-0.231817150854124,0.0724044416546206,
0.922034766023707));
#30729=CARTESIAN_POINT('Ctrl Pts',(-0.186555648217912,-0.155494636948999,
0.933148555080512));
#30730=CARTESIAN_POINT('Ctrl Pts',(0.029462341223335,-0.241067470577576,
0.944262344137316));
#30731=CARTESIAN_POINT('Ctrl Pts',(0.184024675492061,-0.130631009068519,
0.953348649759223));
#30732=CARTESIAN_POINT('Ctrl Pts',(0.205221751249722,-0.031098714158076,
0.958730359028861));
#30733=CARTESIAN_POINT('Ctrl Pts',(0.205150677731907,-5.25566492129668E-5,
0.960407471946232));
#30734=CARTESIAN_POINT('Ctrl Pts',(0.205205445749305,0.000116004416325009,
0.884592528053768));
#30735=CARTESIAN_POINT('Ctrl Pts',(0.205343275267841,0.0267417723340512,
0.886031789520656));
#30736=CARTESIAN_POINT('Ctrl Pts',(0.188156931475396,0.121730614284078,
0.891175647339813));
#30737=CARTESIAN_POINT('Ctrl Pts',(0.0448304764247631,0.238686010114805,
0.900024101511237));
#30738=CARTESIAN_POINT('Ctrl Pts',(-0.176220286722883,0.167116974718297,
0.911137890568042));
#30739=CARTESIAN_POINT('Ctrl Pts',(-0.235976306336092,-0.0574188764093974,
0.922251679624847));
#30740=CARTESIAN_POINT('Ctrl Pts',(-0.0797396575425977,-0.229397140881452,
0.933365468681649));
#30741=CARTESIAN_POINT('Ctrl Pts',(0.142604551604849,-0.192546391773689,
0.944145751491291));
#30742=CARTESIAN_POINT('Ctrl Pts',(0.205352442373934,-0.0618394542260256,
0.951221437948663));
#30743=CARTESIAN_POINT('Ctrl Pts',(0.205743448352251,0.000106566711118368,
0.954592528053768));
#30744=CARTESIAN_POINT('Origin',(0.,0.,0.645407471946233));
#30745=CARTESIAN_POINT('',(0.205269394176581,-0.000252214316689744,0.814592528053768));
#30746=CARTESIAN_POINT('',(0.205654271051376,0.000148184871923512,0.820407471946232));
#30747=CARTESIAN_POINT('',(0.205475,1.17874941047504E-14,0.645407471946233));
#30748=CARTESIAN_POINT('',(0.0530170217188605,-0.198517432567172,0.8));
#30749=CARTESIAN_POINT('Ctrl Pts',(0.0530170217188587,-0.198517432567173,
0.8));
#30750=CARTESIAN_POINT('Ctrl Pts',(0.119028790974553,-0.18088801151799,
0.803704596352268));
#30751=CARTESIAN_POINT('Ctrl Pts',(0.192500600447326,-0.111310459456284,
0.80856877237019));
#30752=CARTESIAN_POINT('Ctrl Pts',(0.205431969941924,-0.0216798251681207,
0.813432948388113));
#30753=CARTESIAN_POINT('Ctrl Pts',(0.205269394176581,-0.000252214316689755,
0.814592528053767));
#30754=CARTESIAN_POINT('',(-0.0531250535940746,-0.19887604744663,0.8));
#30755=CARTESIAN_POINT('Origin',(0.,0.,0.8));
#30756=CARTESIAN_POINT('Ctrl Pts',(-0.053125080564462,-0.198876136975597,
0.8));
#30757=CARTESIAN_POINT('Ctrl Pts',(0.0113386551506616,-0.21601151578625,
0.803632291818556));
#30758=CARTESIAN_POINT('Ctrl Pts',(0.149296237339328,-0.184051126983177,
0.810434782467299));
#30759=CARTESIAN_POINT('Ctrl Pts',(0.205166930984713,-0.0581571994559903,
0.817237273116043));
#30760=CARTESIAN_POINT('Ctrl Pts',(0.205654271051376,0.000148184871923506,
0.820407471946232));
#30761=CARTESIAN_POINT('Origin',(0.,0.,3.1));
#30762=CARTESIAN_POINT('',(-0.126245549239308,1.45328325776573E-5,2.71934196736194));
#30763=CARTESIAN_POINT('',(-0.126374981062586,-0.000161346902988299,2.70565803263806));
#30764=CARTESIAN_POINT('',(-0.12645,1.54856587752183E-17,3.1));
#30765=CARTESIAN_POINT('',(-0.0958116152722464,0.0825211298936403,2.7));
#30766=CARTESIAN_POINT('Ctrl Pts',(-0.126374981062586,-0.000161346902988299,
2.70565803263806));
#30767=CARTESIAN_POINT('Ctrl Pts',(-0.126107573254536,0.0297492098111863,
2.70377202175871));
#30768=CARTESIAN_POINT('Ctrl Pts',(-0.115369380269341,0.0598134784363487,
2.70188601087935));
#30769=CARTESIAN_POINT('Ctrl Pts',(-0.0958116152722464,0.0825211298936403,
2.7));
#30770=CARTESIAN_POINT('',(-0.12645,1.54856587752183E-17,2.7));
#30771=CARTESIAN_POINT('Origin',(0.,0.,2.7));
#30772=CARTESIAN_POINT('',(-0.12645,-1.54856587752183E-17,2.6));
#30773=CARTESIAN_POINT('',(-0.12645,1.54856587752183E-17,3.1));
#30774=CARTESIAN_POINT('Origin',(0.,0.,2.6));
#30775=CARTESIAN_POINT('',(0.095991445127536,0.0826500758460347,2.7));
#30776=CARTESIAN_POINT('Origin',(0.,0.,2.7));
#30777=CARTESIAN_POINT('Ctrl Pts',(0.0959918005672157,0.0826503307119909,
2.7));
#30778=CARTESIAN_POINT('Ctrl Pts',(0.0697118516972522,0.11301027640157,
2.70253749952686));
#30779=CARTESIAN_POINT('Ctrl Pts',(0.0277082938822606,0.129939474688335,
2.70507499905372));
#30780=CARTESIAN_POINT('Ctrl Pts',(-0.0122513412479025,0.126048724837631,
2.70761249858058));
#30781=CARTESIAN_POINT('Ctrl Pts',(-0.0537056163258554,0.122012446376998,
2.71024491008919));
#30782=CARTESIAN_POINT('Ctrl Pts',(-0.092960208469122,0.0955696038330054,
2.7128773215978));
#30783=CARTESIAN_POINT('Ctrl Pts',(-0.1122448026076,0.0586681233168463,
2.71550973310641));
#30784=CARTESIAN_POINT('Ctrl Pts',(-0.121602899042457,0.0407612070094829,
2.71678714452492));
#30785=CARTESIAN_POINT('Ctrl Pts',(-0.126258460357629,0.0203914906379236,
2.71806455594343));
#30786=CARTESIAN_POINT('Ctrl Pts',(-0.126245549239308,1.45328325776573E-5,
2.71934196736194));
#30787=CARTESIAN_POINT('Origin',(0.,0.,3.1));
#30788=CARTESIAN_POINT('',(-0.126511755116174,-0.000105182036976022,2.76934196736194));
#30789=CARTESIAN_POINT('',(-0.12664039552615,3.66938896950461E-5,2.75565803263806));
#30790=CARTESIAN_POINT('',(-0.12645,1.54856587752183E-17,3.1));
#30791=CARTESIAN_POINT('Ctrl Pts',(-0.12664039552615,3.66938896950461E-5,
2.75565803263806));
#30792=CARTESIAN_POINT('Ctrl Pts',(-0.126647890342436,0.00202721792373194,
2.75553223565232));
#30793=CARTESIAN_POINT('Ctrl Pts',(-0.126604975133189,0.00401740611511355,
2.75540643866659));
#30794=CARTESIAN_POINT('Ctrl Pts',(-0.126510633504476,0.00600514734308786,
2.75528064168085));
#30795=CARTESIAN_POINT('Ctrl Pts',(-0.124536452742414,0.0476003640650105,
2.75264823017224));
#30796=CARTESIAN_POINT('Ctrl Pts',(-0.10004305012127,0.0881240748873803,
2.75001581866363));
#30797=CARTESIAN_POINT('Ctrl Pts',(-0.064133889095878,0.109212690295602,
2.74738340715501));
#30798=CARTESIAN_POINT('Ctrl Pts',(-0.0282247280704852,0.130301305703824,
2.7447509956464));
#30799=CARTESIAN_POINT('Ctrl Pts',(0.0191001913591554,0.131954825697897,
2.74211858413779));
#30800=CARTESIAN_POINT('Ctrl Pts',(0.0563882647159258,0.113411365221879,
2.73948617262918));
#30801=CARTESIAN_POINT('Ctrl Pts',(0.0936763380726957,0.0948679047458623,
2.73685376112057));
#30802=CARTESIAN_POINT('Ctrl Pts',(0.120927565356595,0.0561274637997562,
2.73422134961196));
#30803=CARTESIAN_POINT('Ctrl Pts',(0.125787645771127,0.0147753877020813,
2.73158893810334));
#30804=CARTESIAN_POINT('Ctrl Pts',(0.13064772618566,-0.0265766883955932,
2.72895652659473));
#30805=CARTESIAN_POINT('Ctrl Pts',(0.113116659730824,-0.0705403996448371,
2.72632411508612));
#30806=CARTESIAN_POINT('Ctrl Pts',(0.0811433928446468,-0.0972323182667412,
2.72369170357751));
#30807=CARTESIAN_POINT('Ctrl Pts',(0.0491701259584694,-0.123924236888645,
2.7210592920689));
#30808=CARTESIAN_POINT('Ctrl Pts',(0.00275465864095025,-0.133344362883211,
2.71842688056028));
#30809=CARTESIAN_POINT('Ctrl Pts',(-0.0370665720412133,-0.121131225367919,
2.71579446905167));
#30810=CARTESIAN_POINT('Ctrl Pts',(-0.0768878027233769,-0.108918087852628,
2.71316205754306));
#30811=CARTESIAN_POINT('Ctrl Pts',(-0.110114796770184,-0.0750716868274789,
2.71052964603445));
#30812=CARTESIAN_POINT('Ctrl Pts',(-0.121670218183899,-0.0351354691109218,
2.70789723452584));
#30813=CARTESIAN_POINT('Ctrl Pts',(-0.124946671651124,-0.023811852747613,
2.70715083389658));
#30814=CARTESIAN_POINT('Ctrl Pts',(-0.126480809379052,-0.0119986372375087,
2.70640443326732));
#30815=CARTESIAN_POINT('Ctrl Pts',(-0.126374981062586,-0.000161346902988299,
2.70565803263806));
#30816=CARTESIAN_POINT('Ctrl Pts',(-0.126245549239308,1.45328325776573E-5,
2.71934196736194));
#30817=CARTESIAN_POINT('Ctrl Pts',(-0.126231853912779,-0.0216001006849982,
2.72069696745204));
#30818=CARTESIAN_POINT('Ctrl Pts',(-0.120965346567412,-0.0432228820262939,
2.72205196754215));
#30819=CARTESIAN_POINT('Ctrl Pts',(-0.110486681315658,-0.0619230805928583,
2.72340696763225));
#30820=CARTESIAN_POINT('Ctrl Pts',(-0.0901293697515468,-0.0982526854980795,
2.72603937914086));
#30821=CARTESIAN_POINT('Ctrl Pts',(-0.0501001504896328,-0.123551776820195,
2.72867179064947));
#30822=CARTESIAN_POINT('Ctrl Pts',(-0.00855140384117574,-0.126362344661561,
2.73130420215808));
#30823=CARTESIAN_POINT('Ctrl Pts',(0.0329973428072813,-0.129172912502927,
2.7339366136667));
#30824=CARTESIAN_POINT('Ctrl Pts',(0.076065616842282,-0.109494956863544,
2.73656902517531));
#30825=CARTESIAN_POINT('Ctrl Pts',(0.10113334277539,-0.0762433600374486,
2.73920143668392));
#30826=CARTESIAN_POINT('Ctrl Pts',(0.126201068708497,-0.0429917632113539,
2.74183384819253));
#30827=CARTESIAN_POINT('Ctrl Pts',(0.133268246539712,0.00383347480145232,
2.74446625970114));
#30828=CARTESIAN_POINT('Ctrl Pts',(0.119129452671912,0.0430029706396828,
2.74709867120975));
#30829=CARTESIAN_POINT('Ctrl Pts',(0.104990658804112,0.0821724664779139,
2.74973108271837));
#30830=CARTESIAN_POINT('Ctrl Pts',(0.0696458932372969,0.113686220141568,
2.75236349422698));
#30831=CARTESIAN_POINT('Ctrl Pts',(0.0291183743037611,0.123260050517998,
2.75499590573559));
#30832=CARTESIAN_POINT('Ctrl Pts',(-0.0114091446297752,0.132833880894428,
2.7576283172442));
#30833=CARTESIAN_POINT('Ctrl Pts',(-0.0571194169300318,0.120467787983633,
2.76026072875281));
#30834=CARTESIAN_POINT('Ctrl Pts',(-0.0872917850925406,0.0917667415677358,
2.76289314026143));
#30835=CARTESIAN_POINT('Ctrl Pts',(-0.111930332277198,0.0683296655464438,
2.76504274929493));
#30836=CARTESIAN_POINT('Ctrl Pts',(-0.126207827945274,0.0340000461494869,
2.76719235832844));
#30837=CARTESIAN_POINT('Ctrl Pts',(-0.126511755116174,-0.000105182036976022,
2.76934196736194));
#30838=CARTESIAN_POINT('Origin',(0.,0.,3.1));
#30839=CARTESIAN_POINT('',(-0.126553655479795,9.34644642624216E-5,2.81934196736194));
#30840=CARTESIAN_POINT('',(-0.126295222915983,7.47437243418914E-5,2.80565803263806));
#30841=CARTESIAN_POINT('',(-0.12645,1.54856587752183E-17,3.1));
#30842=CARTESIAN_POINT('Ctrl Pts',(-0.126295222915983,7.47437243418914E-5,
2.80565803263806));
#30843=CARTESIAN_POINT('Ctrl Pts',(-0.126381902901803,0.0159778826374278,
2.80466003803733));
#30844=CARTESIAN_POINT('Ctrl Pts',(-0.12359488800886,0.0318517555514631,
2.8036620434366));
#30845=CARTESIAN_POINT('Ctrl Pts',(-0.117794192788123,0.0465350551086,2.80266404883586));
#30846=CARTESIAN_POINT('Ctrl Pts',(-0.102493692318657,0.0852652112740412,
2.80003163732725));
#30847=CARTESIAN_POINT('Ctrl Pts',(-0.0662256093040858,0.115711992156929,
2.79739922581864));
#30848=CARTESIAN_POINT('Ctrl Pts',(-0.0254308011719313,0.124073552736451,
2.79476681431003));
#30849=CARTESIAN_POINT('Ctrl Pts',(0.0153640069602226,0.132435113315973,
2.79213440280142));
#30850=CARTESIAN_POINT('Ctrl Pts',(0.0606855402099605,0.11871145359213,
2.78950199129281));
#30851=CARTESIAN_POINT('Ctrl Pts',(0.089988893871543,0.0891234665506248,
2.78686957978419));
#30852=CARTESIAN_POINT('Ctrl Pts',(0.119292247533126,0.0595354795091193,
2.78423716827558));
#30853=CARTESIAN_POINT('Ctrl Pts',(0.132577421606553,0.0140831651499525,
2.78160475676697));
#30854=CARTESIAN_POINT('Ctrl Pts',(0.123822034418855,-0.0266288104888323,
2.77897234525835));
#30855=CARTESIAN_POINT('Ctrl Pts',(0.115066647231157,-0.067340786127616,
2.77633993374974));
#30856=CARTESIAN_POINT('Ctrl Pts',(0.084270698782333,-0.103312423046018,
2.77370752224113));
#30857=CARTESIAN_POINT('Ctrl Pts',(0.045394477490254,-0.11823815061478,
2.77107511073252));
#30858=CARTESIAN_POINT('Ctrl Pts',(0.00651825619817509,-0.133163878183541,
2.76844269922391));
#30859=CARTESIAN_POINT('Ctrl Pts',(-0.0404382379371578,-0.127043696402664,
2.7658102877153));
#30860=CARTESIAN_POINT('Ctrl Pts',(-0.0741890055533361,-0.102650244201489,
2.76317787620668));
#30861=CARTESIAN_POINT('Ctrl Pts',(-0.106326900403039,-0.0794224998497761,
2.76067126168381));
#30862=CARTESIAN_POINT('Ctrl Pts',(-0.126491054782899,-0.0396262314391609,
2.75816464716093));
#30863=CARTESIAN_POINT('Ctrl Pts',(-0.12664039552615,3.66938896950461E-5,
2.75565803263806));
#30864=CARTESIAN_POINT('Ctrl Pts',(-0.126511755116174,-0.000105182036976022,
2.76934196736194));
#30865=CARTESIAN_POINT('Ctrl Pts',(-0.12658001719922,-0.00776522082814862,
2.76982476983705));
#30866=CARTESIAN_POINT('Ctrl Pts',(-0.125943379547996,-0.015413940155386,
2.77030757231215));
#30867=CARTESIAN_POINT('Ctrl Pts',(-0.124560912333973,-0.022925385115547,
2.77079037478726));
#30868=CARTESIAN_POINT('Ctrl Pts',(-0.117023207388135,-0.0638804654619373,
2.77342278629587));
#30869=CARTESIAN_POINT('Ctrl Pts',(-0.0873133334716985,-0.100754626233721,
2.77605519780449));
#30870=CARTESIAN_POINT('Ctrl Pts',(-0.0488993400374831,-0.116832476461904,
2.7786876093131));
#30871=CARTESIAN_POINT('Ctrl Pts',(-0.0104853466032667,-0.132910326690088,
2.78132002082171));
#30872=CARTESIAN_POINT('Ctrl Pts',(0.0366327663487292,-0.128191866374669,
2.78395243233032));
#30873=CARTESIAN_POINT('Ctrl Pts',(0.0710957359713387,-0.104815935790865,
2.78658484383893));
#30874=CARTESIAN_POINT('Ctrl Pts',(0.105558705593947,-0.0814400052070627,
2.78921725534754));
#30875=CARTESIAN_POINT('Ctrl Pts',(0.12736653188717,-0.0394066043548766,
2.79184966685616));
#30876=CARTESIAN_POINT('Ctrl Pts',(0.126633373335447,0.00222985575585417,
2.79448207836477));
#30877=CARTESIAN_POINT('Ctrl Pts',(0.125900214783723,0.0438663158665862,
2.79711448987338));
#30878=CARTESIAN_POINT('Ctrl Pts',(0.102626071387052,0.0851058352358628,
2.79974690138199));
#30879=CARTESIAN_POINT('Ctrl Pts',(0.067361470922124,0.107253965297467,
2.8023793128906));
#30880=CARTESIAN_POINT('Ctrl Pts',(0.032096870457197,0.12940209535907,2.80501172439922));
#30881=CARTESIAN_POINT('Ctrl Pts',(-0.0151581870759861,0.132458836113002,
2.80764413590783));
#30882=CARTESIAN_POINT('Ctrl Pts',(-0.052982302223486,0.115038507268346,
2.81027654741644));
#30883=CARTESIAN_POINT('Ctrl Pts',(-0.0908064173709864,0.0976181784236899,
2.81290895892505));
#30884=CARTESIAN_POINT('Ctrl Pts',(-0.119199590132803,0.059720779980445,
2.81554137043366));
#30885=CARTESIAN_POINT('Ctrl Pts',(-0.12529077505034,0.0185257648347912,
2.81817378194227));
#30886=CARTESIAN_POINT('Ctrl Pts',(-0.126191803554164,0.0124320600196876,
2.81856317708216));
#30887=CARTESIAN_POINT('Ctrl Pts',(-0.126604835154177,0.00626619900254654,
2.81895257222205));
#30888=CARTESIAN_POINT('Ctrl Pts',(-0.126553655479795,9.34644642624216E-5,
2.81934196736194));
#30889=CARTESIAN_POINT('Origin',(0.,0.,3.1));
#30890=CARTESIAN_POINT('',(-0.126249156657861,1.39511119994357E-5,2.86934196736194));
#30891=CARTESIAN_POINT('',(-0.126382098607383,-0.000107526861324363,2.85565803263806));
#30892=CARTESIAN_POINT('',(-0.12645,1.54856587752183E-17,3.1));
#30893=CARTESIAN_POINT('Ctrl Pts',(-0.126382098607383,-0.000107526861324363,
2.85565803263806));
#30894=CARTESIAN_POINT('Ctrl Pts',(-0.126136963881609,0.0296424659657165,
2.85378784042233));
#30895=CARTESIAN_POINT('Ctrl Pts',(-0.115629819550324,0.0595483512746711,
2.8519176482066));
#30896=CARTESIAN_POINT('Ctrl Pts',(-0.0964566207792818,0.0820798491866498,
2.85004745599088));
#30897=CARTESIAN_POINT('Ctrl Pts',(-0.0694691546368386,0.113794329607957,
2.84741504448226));
#30898=CARTESIAN_POINT('Ctrl Pts',(-0.0253122344935349,0.130898446561428,
2.84478263297365));
#30899=CARTESIAN_POINT('Ctrl Pts',(0.0159971616939493,0.125638656106515,
2.84215022146504));
#30900=CARTESIAN_POINT('Ctrl Pts',(0.0573065578814334,0.120378865651602,
2.83951780995643));
#30901=CARTESIAN_POINT('Ctrl Pts',(0.0957684301130981,0.0927551677883048,
2.83688539844782));
#30902=CARTESIAN_POINT('Ctrl Pts',(0.113947449240963,0.0552897840743664,
2.83425298693921));
#30903=CARTESIAN_POINT('Ctrl Pts',(0.132126468368828,0.017824400360428,
2.83162057543059));
#30904=CARTESIAN_POINT('Ctrl Pts',(0.130022634392893,-0.0294826692041511,
2.82898816392198));
#30905=CARTESIAN_POINT('Ctrl Pts',(0.108589645677727,-0.0651864287383833,
2.82635575241337));
#30906=CARTESIAN_POINT('Ctrl Pts',(0.0871566569625619,-0.100890188272616,
2.82372334090476));
#30907=CARTESIAN_POINT('Ctrl Pts',(0.0463945135081664,-0.124990637776501,
2.82109092939615));
#30908=CARTESIAN_POINT('Ctrl Pts',(0.00478129192095443,-0.126562708640517,
2.81845851788753));
#30909=CARTESIAN_POINT('Ctrl Pts',(-0.036831929666257,-0.128134779504533,
2.81582610637892));
#30910=CARTESIAN_POINT('Ctrl Pts',(-0.0792962293862848,-0.10717847172868,
2.81319369487031));
#30911=CARTESIAN_POINT('Ctrl Pts',(-0.103361920284118,-0.0731935521167569,
2.8105612833617));
#30912=CARTESIAN_POINT('Ctrl Pts',(-0.118303874448411,-0.0520929274442991,
2.80892686645382));
#30913=CARTESIAN_POINT('Ctrl Pts',(-0.126153267003299,-0.0259698452031535,
2.80729244954594));
#30914=CARTESIAN_POINT('Ctrl Pts',(-0.126295222915983,7.47437243418914E-5,
2.80565803263806));
#30915=CARTESIAN_POINT('Ctrl Pts',(-0.126553655479795,9.34644642624216E-5,
2.81934196736194));
#30916=CARTESIAN_POINT('Ctrl Pts',(-0.126258847364269,-0.0354630774409815,
2.82158498373066));
#30917=CARTESIAN_POINT('Ctrl Pts',(-0.110561244917173,-0.0712476866904275,
2.82382800009939));
#30918=CARTESIAN_POINT('Ctrl Pts',(-0.0840069629213228,-0.0947829738698732,
2.82607101646811));
#30919=CARTESIAN_POINT('Ctrl Pts',(-0.0528427688015115,-0.122404065580821,
2.82870342797672));
#30920=CARTESIAN_POINT('Ctrl Pts',(-0.00672518348863185,-0.133153617154654,
2.83133583948533));
#30921=CARTESIAN_POINT('Ctrl Pts',(0.0334400182730099,-0.122158697506542,
2.83396825099395));
#30922=CARTESIAN_POINT('Ctrl Pts',(0.0736052200346521,-0.111163777858429,
2.83660066250256));
#30923=CARTESIAN_POINT('Ctrl Pts',(0.107818038245057,-0.0784243869883676,
2.83923307401117));
#30924=CARTESIAN_POINT('Ctrl Pts',(0.120569301232658,-0.0387817708073496,
2.84186548551978));
#30925=CARTESIAN_POINT('Ctrl Pts',(0.13332056422026,0.000860845373668366,
2.84449789702839));
#30926=CARTESIAN_POINT('Ctrl Pts',(0.124610271985061,0.0474066868656423,
2.847130308537));
#30927=CARTESIAN_POINT('Ctrl Pts',(0.0983869277745218,0.0797558433812344,
2.84976272004562));
#30928=CARTESIAN_POINT('Ctrl Pts',(0.0721635835639831,0.112104999896826,
2.85239513155423));
#30929=CARTESIAN_POINT('Ctrl Pts',(0.0284271873781034,0.130257471436035,
2.85502754306284));
#30930=CARTESIAN_POINT('Ctrl Pts',(-0.0129959127687897,0.125984476806968,
2.85765995457145));
#30931=CARTESIAN_POINT('Ctrl Pts',(-0.0544190129156822,0.121711482177902,
2.86029236608007));
#30932=CARTESIAN_POINT('Ctrl Pts',(-0.0935288170235893,0.0950130213805616,
2.86292477758868));
#30933=CARTESIAN_POINT('Ctrl Pts',(-0.11259627866674,0.0579918974128127,
2.86555718909729));
#30934=CARTESIAN_POINT('Ctrl Pts',(-0.121734428756244,0.0402493895934286,
2.86681878185217));
#30935=CARTESIAN_POINT('Ctrl Pts',(-0.126269172738684,0.0201359308353815,
2.86808037460706));
#30936=CARTESIAN_POINT('Ctrl Pts',(-0.126249156657861,1.39511119994357E-5,
2.86934196736194));
#30937=CARTESIAN_POINT('Origin',(0.,0.,3.1));
#30938=CARTESIAN_POINT('',(-0.126504381589359,-0.000106615302056266,2.91934196736194));
#30939=CARTESIAN_POINT('',(-0.126643227510109,3.12951648517141E-5,2.90565803263806));
#30940=CARTESIAN_POINT('',(-0.12645,1.54856587752183E-17,3.1));
#30941=CARTESIAN_POINT('Ctrl Pts',(-0.126643227510109,3.12951648517141E-5,
2.90565803263806));
#30942=CARTESIAN_POINT('Ctrl Pts',(-0.126649060558016,0.00177143581201147,
2.90554805431595));
#30943=CARTESIAN_POINT('Ctrl Pts',(-0.126616264808321,0.00351135171962892,
2.90543807599384));
#30944=CARTESIAN_POINT('Ctrl Pts',(-0.126544152713349,0.00524963660346066,
2.90532809767173));
#30945=CARTESIAN_POINT('Ctrl Pts',(-0.124818097022822,0.0468567555849086,
2.90269568616312));
#30946=CARTESIAN_POINT('Ctrl Pts',(-0.100566951953931,0.0875294297116145,
2.9000632746545));
#30947=CARTESIAN_POINT('Ctrl Pts',(-0.0647841163292417,0.1088301407863,
2.89743086314589));
#30948=CARTESIAN_POINT('Ctrl Pts',(-0.0290012807045523,0.130130851860986,
2.89479845163728));
#30949=CARTESIAN_POINT('Ctrl Pts',(0.0183132454759347,0.13205959988365,
2.89216604012867));
#30950=CARTESIAN_POINT('Ctrl Pts',(0.0557110953405879,0.113742055209456,
2.88953362862006));
#30951=CARTESIAN_POINT('Ctrl Pts',(0.0931089452052417,0.0954245105352619,
2.88690121711144));
#30952=CARTESIAN_POINT('Ctrl Pts',(0.120590118754061,0.0568606731642085,
2.88426880560283));
#30953=CARTESIAN_POINT('Ctrl Pts',(0.125696998005905,0.0155320946228576,
2.88163639409422));
#30954=CARTESIAN_POINT('Ctrl Pts',(0.130803877257748,-0.025796483918492,
2.87900398258561));
#30955=CARTESIAN_POINT('Ctrl Pts',(0.113536462212617,-0.0698898036301388,
2.87637157107699));
#30956=CARTESIAN_POINT('Ctrl Pts',(0.081722324704119,-0.0967597174754642,
2.87373915956838));
#30957=CARTESIAN_POINT('Ctrl Pts',(0.0499081871956208,-0.12362963132079,
2.87110674805977));
#30958=CARTESIAN_POINT('Ctrl Pts',(0.0035473272237559,-0.133276139299794,
2.86847433655116));
#30959=CARTESIAN_POINT('Ctrl Pts',(-0.0363441991716402,-0.12132633857832,
2.86584192504255));
#30960=CARTESIAN_POINT('Ctrl Pts',(-0.0762357255670363,-0.109376537856846,
2.86320951353394));
#30961=CARTESIAN_POINT('Ctrl Pts',(-0.109657918385963,-0.0758304284348936,
2.86057710202533));
#30962=CARTESIAN_POINT('Ctrl Pts',(-0.121460008724635,-0.035894951779346,
2.85794469051671));
#30963=CARTESIAN_POINT('Ctrl Pts',(-0.124877324339263,-0.0243315656302484,
2.85718247122383));
#30964=CARTESIAN_POINT('Ctrl Pts',(-0.126482006208201,-0.0122324936456281,
2.85642025193094));
#30965=CARTESIAN_POINT('Ctrl Pts',(-0.126382098607383,-0.000107526861324363,
2.85565803263806));
#30966=CARTESIAN_POINT('Ctrl Pts',(-0.126249156657861,1.39511119994357E-5,
2.86934196736194));
#30967=CARTESIAN_POINT('Ctrl Pts',(-0.126227407627626,-0.0218501465218449,
2.87071278611567));
#30968=CARTESIAN_POINT('Ctrl Pts',(-0.120828074559444,-0.0437243044457016,
2.8720836048694));
#30969=CARTESIAN_POINT('Ctrl Pts',(-0.110113563989691,-0.0625778327914941,
2.87345442362312));
#30970=CARTESIAN_POINT('Ctrl Pts',(-0.0895382684910942,-0.0987826518898959,
2.87608683513174));
#30971=CARTESIAN_POINT('Ctrl Pts',(-0.049362558315506,-0.12384850294854,
2.87871924664035));
#30972=CARTESIAN_POINT('Ctrl Pts',(-0.00779867057972899,-0.126412668959158,
2.88135165814896));
#30973=CARTESIAN_POINT('Ctrl Pts',(0.0337652171560469,-0.128976834969775,
2.88398406965757));
#30974=CARTESIAN_POINT('Ctrl Pts',(0.0767172824520115,-0.109039315932365,
2.88661648116618));
#30975=CARTESIAN_POINT('Ctrl Pts',(0.101586725761179,-0.0756380809090063,
2.88924889267479));
#30976=CARTESIAN_POINT('Ctrl Pts',(0.126456169070347,-0.0422368458856463,
2.89188130418341));
#30977=CARTESIAN_POINT('Ctrl Pts',(0.133242990392717,0.00462810512366429,
2.89451371569202));
#30978=CARTESIAN_POINT('Ctrl Pts',(0.118870624347205,0.0437122042621813,
2.89714612720063));
#30979=CARTESIAN_POINT('Ctrl Pts',(0.104498258301693,0.0827963034006972,
2.89977853870924));
#30980=CARTESIAN_POINT('Ctrl Pts',(0.0689667048882996,0.11409955066842,
2.90241095021785));
#30981=CARTESIAN_POINT('Ctrl Pts',(0.0283829370476986,0.123431726145854,
2.90504336172646));
#30982=CARTESIAN_POINT('Ctrl Pts',(-0.0122008307929037,0.132763901623287,
2.90767577323508));
#30983=CARTESIAN_POINT('Ctrl Pts',(-0.0578368130607139,0.120125005310431,
2.91030818474369));
#30984=CARTESIAN_POINT('Ctrl Pts',(-0.0878375513946906,0.0912444338001155,
2.9129405962523));
#30985=CARTESIAN_POINT('Ctrl Pts',(-0.112155666680576,0.0678343076994951,
2.91507438662218));
#30986=CARTESIAN_POINT('Ctrl Pts',(-0.126200703597521,0.0337526498432798,
2.91720817699206));
#30987=CARTESIAN_POINT('Ctrl Pts',(-0.126504381589359,-0.000106615302056266,
2.91934196736194));
#30988=CARTESIAN_POINT('Origin',(0.,0.,3.1));
#30989=CARTESIAN_POINT('',(-0.126560384998288,9.09688539718206E-5,2.96934196736194));
#30990=CARTESIAN_POINT('',(-0.126299886768127,7.7729991388234E-5,2.95565803263806));
#30991=CARTESIAN_POINT('',(-0.12645,1.54856587752183E-17,3.1));
#30992=CARTESIAN_POINT('Ctrl Pts',(-0.126299886768127,7.7729991388234E-5,
2.95565803263806));
#30993=CARTESIAN_POINT('Ctrl Pts',(-0.126388830708229,0.0157273402429332,
2.95467585670095));
#30994=CARTESIAN_POINT('Ctrl Pts',(-0.123692081773928,0.0313473916688532,
2.95369368076385));
#30995=CARTESIAN_POINT('Ctrl Pts',(-0.118069607334697,0.0458317476680533,
2.95271150482674));
#30996=CARTESIAN_POINT('Ctrl Pts',(-0.103000345442256,0.0846524762021514,
2.95007909331813));
#30997=CARTESIAN_POINT('Ctrl Pts',(-0.066914478664464,0.115315070279254,
2.94744668180952));
#30998=CARTESIAN_POINT('Ctrl Pts',(-0.0261702583026162,0.123919727448441,
2.9448142703009));
#30999=CARTESIAN_POINT('Ctrl Pts',(0.0145739620592316,0.132524384617628,
2.94218185879229));
#31000=CARTESIAN_POINT('Ctrl Pts',(0.0599765360051347,0.119071104878899,
2.93954944728368));
#31001=CARTESIAN_POINT('Ctrl Pts',(0.0894558125827043,0.0896584567433833,
2.93691703577507));
#31002=CARTESIAN_POINT('Ctrl Pts',(0.118935089160275,0.0602458086078669,
2.93428462426646));
#31003=CARTESIAN_POINT('Ctrl Pts',(0.13249106836951,0.0148737920755634,
2.93165221275785));
#31004=CARTESIAN_POINT('Ctrl Pts',(0.123978626527973,-0.0258897940256335,
2.92901980124923));
#31005=CARTESIAN_POINT('Ctrl Pts',(0.115466184686436,-0.0666533801268299,
2.92638738974062));
#31006=CARTESIAN_POINT('Ctrl Pts',(0.0848853217941264,-0.10280853579692,
2.92375497823201));
#31007=CARTESIAN_POINT('Ctrl Pts',(0.0460987903596358,-0.117965600062524,
2.9211225667234));
#31008=CARTESIAN_POINT('Ctrl Pts',(0.00731225892514568,-0.133122664328129,
2.91849015521479));
#31009=CARTESIAN_POINT('Ctrl Pts',(-0.0396799410515272,-0.127281637189249,
2.91585774370617));
#31010=CARTESIAN_POINT('Ctrl Pts',(-0.0735755578837821,-0.103090341701714,
2.91322533219756));
#31011=CARTESIAN_POINT('Ctrl Pts',(-0.106055065170122,-0.0799097233361643,
2.91070289901106));
#31012=CARTESIAN_POINT('Ctrl Pts',(-0.126509442293762,-0.0398801022208299,
2.90818046582456));
#31013=CARTESIAN_POINT('Ctrl Pts',(-0.126643227510109,3.12951648517141E-5,
2.90565803263806));
#31014=CARTESIAN_POINT('Ctrl Pts',(-0.126504381589359,-0.000106615302056266,
2.91934196736194));
#31015=CARTESIAN_POINT('Ctrl Pts',(-0.126575344636262,-0.00801880085773389,
2.91984058850067));
#31016=CARTESIAN_POINT('Ctrl Pts',(-0.125895951346516,-0.0159188425067759,
2.9203392096394));
#31017=CARTESIAN_POINT('Ctrl Pts',(-0.124421945835367,-0.0236677318103004,
2.92083783077814));
#31018=CARTESIAN_POINT('Ctrl Pts',(-0.116640107541925,-0.0645770792026294,
2.92347024228675));
#31019=CARTESIAN_POINT('Ctrl Pts',(-0.0867109365548968,-0.101273527279515,
2.92610265379536));
#31020=CARTESIAN_POINT('Ctrl Pts',(-0.0482017639084,-0.117122039303909,
2.92873506530397));
#31021=CARTESIAN_POINT('Ctrl Pts',(-0.0096925912619021,-0.132970551328304,
2.93136747681259));
#31022=CARTESIAN_POINT('Ctrl Pts',(0.0373965830440653,-0.127971127300206,
2.9339998883212));
#31023=CARTESIAN_POINT('Ctrl Pts',(0.071719547440819,-0.104390079267275,
2.93663229982981));
#31024=CARTESIAN_POINT('Ctrl Pts',(0.106042511837572,-0.0808090312343449,
2.93926471133842));
#31025=CARTESIAN_POINT('Ctrl Pts',(0.127599266325111,-0.0386463591965834,
2.94189712284703));
#31026=CARTESIAN_POINT('Ctrl Pts',(0.126617818746111,0.00298498082453686,
2.94452953435564));
#31027=CARTESIAN_POINT('Ctrl Pts',(0.125636371167111,0.0446163208456583,
2.94716194586426));
#31028=CARTESIAN_POINT('Ctrl Pts',(0.10211672152157,0.0857163288501385,
2.94979435737287));
#31029=CARTESIAN_POINT('Ctrl Pts',(0.0667206710566959,0.107653769967896,
2.95242676888148));
#31030=CARTESIAN_POINT('Ctrl Pts',(0.0313246205918224,0.129591211085654,
2.95505918039009));
#31031=CARTESIAN_POINT('Ctrl Pts',(-0.0159478306923833,0.13236608531669,
2.9576915918987));
#31032=CARTESIAN_POINT('Ctrl Pts',(-0.0536673890921198,0.114720501579208,
2.96032400340732));
#31033=CARTESIAN_POINT('Ctrl Pts',(-0.0913869474918552,0.0970749178417258,
2.96295641491593));
#31034=CARTESIAN_POINT('Ctrl Pts',(-0.119553613007122,0.059008876135727,
2.96558882642454));
#31035=CARTESIAN_POINT('Ctrl Pts',(-0.125399024116903,0.0177782700249248,
2.96822123793315));
#31036=CARTESIAN_POINT('Ctrl Pts',(-0.12622857074271,0.0119270630632909,
2.96859481440941));
#31037=CARTESIAN_POINT('Ctrl Pts',(-0.126608575570408,0.00601212294639071,
2.96896839088568));
#31038=CARTESIAN_POINT('Ctrl Pts',(-0.126560384998288,9.09688539718206E-5,
2.96934196736194));
#31039=CARTESIAN_POINT('Origin',(0.,0.,3.1));
#31040=CARTESIAN_POINT('',(-0.126250113253048,1.79623087654263E-5,3.01934196736194));
#31041=CARTESIAN_POINT('',(-0.126375290424941,-0.000106230050797054,3.00565803263806));
#31042=CARTESIAN_POINT('',(-0.12645,1.54856587752183E-17,3.1));
#31043=CARTESIAN_POINT('Ctrl Pts',(-0.126375290424941,-0.000106230050797054,
3.00565803263806));
#31044=CARTESIAN_POINT('Ctrl Pts',(-0.126136144258534,0.0293961593132966,
3.00380365908596));
#31045=CARTESIAN_POINT('Ctrl Pts',(-0.115821844223656,0.0590492800488679,
3.00194928553385));
#31046=CARTESIAN_POINT('Ctrl Pts',(-0.0969443855366137,0.0815031740695626,
3.00009491198175));
#31047=CARTESIAN_POINT('Ctrl Pts',(-0.0701465273355013,0.11337802957871,
2.99746250047314));
#31048=CARTESIAN_POINT('Ctrl Pts',(-0.0260923921578653,0.130745171841498,
2.99483008896453));
#31049=CARTESIAN_POINT('Ctrl Pts',(0.0152476360635642,0.125731821210699,
2.99219767745592));
#31050=CARTESIAN_POINT('Ctrl Pts',(0.0565876642849942,0.120718470579899,
2.98956526594731));
#31051=CARTESIAN_POINT('Ctrl Pts',(0.0952135855502181,0.0933246270555131,
2.98693285443869));
#31052=CARTESIAN_POINT('Ctrl Pts',(0.113615704700958,0.0559683206447137,
2.98430044293008));
#31053=CARTESIAN_POINT('Ctrl Pts',(0.132017823851697,0.0186120142339143,
2.98166803142147));
#31054=CARTESIAN_POINT('Ctrl Pts',(0.130196140887953,-0.0287067550632971,
2.97903561991286));
#31055=CARTESIAN_POINT('Ctrl Pts',(0.108976451346127,-0.0645376969103253,
2.97640320840425));
#31056=CARTESIAN_POINT('Ctrl Pts',(0.0877567618043009,-0.100368638757354,
2.97377079689564));
#31057=CARTESIAN_POINT('Ctrl Pts',(0.0471390656843917,-0.124711753154198,
2.97113838538702));
#31058=CARTESIAN_POINT('Ctrl Pts',(0.00553595882347027,-0.126531950235485,
2.96850597387841));
#31059=CARTESIAN_POINT('Ctrl Pts',(-0.03606714803745,-0.128352147316772,
2.9658735623698));
#31060=CARTESIAN_POINT('Ctrl Pts',(-0.078655665639383,-0.107649427082503,
2.96324115086119));
#31061=CARTESIAN_POINT('Ctrl Pts',(-0.102923595936805,-0.0738086354698221,
2.96060873935258));
#31062=CARTESIAN_POINT('Ctrl Pts',(-0.118136947531953,-0.0525941414955858,
2.95895850378107));
#31063=CARTESIAN_POINT('Ctrl Pts',(-0.126150444648563,-0.0262164832362216,
2.95730826820956));
#31064=CARTESIAN_POINT('Ctrl Pts',(-0.126299886768127,7.7729991388234E-5,
2.95565803263806));
#31065=CARTESIAN_POINT('Ctrl Pts',(-0.126560384998288,9.09688539718206E-5,
2.96934196736194));
#31066=CARTESIAN_POINT('Ctrl Pts',(-0.126269000075926,-0.0357113665330736,
2.97160080239429));
#31067=CARTESIAN_POINT('Ctrl Pts',(-0.110322654377183,-0.0717408868526332,
2.97385963742664));
#31068=CARTESIAN_POINT('Ctrl Pts',(-0.0834402350166293,-0.0952822612815302,
2.97611847245899));
#31069=CARTESIAN_POINT('Ctrl Pts',(-0.0521118781022804,-0.122717015961572,
2.9787508839676));
#31070=CARTESIAN_POINT('Ctrl Pts',(-0.00593100756928766,-0.133191354806051,
2.98138329547621));
#31071=CARTESIAN_POINT('Ctrl Pts',(0.0341679124015605,-0.12195710679034,
2.98401570698482));
#31072=CARTESIAN_POINT('Ctrl Pts',(0.0742668323724097,-0.110722858774629,
2.98664811849343));
#31073=CARTESIAN_POINT('Ctrl Pts',(0.108283801781115,-0.0777800238987277,
2.98928053000205));
#31074=CARTESIAN_POINT('Ctrl Pts',(0.120798430769142,-0.038062071124208,
2.99191294151066));
#31075=CARTESIAN_POINT('Ctrl Pts',(0.133313059757168,0.00165588165031116,
2.99454535301927));
#31076=CARTESIAN_POINT('Ctrl Pts',(0.124325348324518,0.0481489523234473,
2.99717776452788));
#31077=CARTESIAN_POINT('Ctrl Pts',(0.0979095575425482,0.0803411518237943,
2.9998101760365));
#31078=CARTESIAN_POINT('Ctrl Pts',(0.0714937667605778,0.112533351324142,
3.00244258754511));
#31079=CARTESIAN_POINT('Ctrl Pts',(0.0276498966292865,0.130424679651699,
3.00507499905372));
#31080=CARTESIAN_POINT('Ctrl Pts',(-0.0137469851400152,0.125904735947905,
3.00770741056233));
#31081=CARTESIAN_POINT('Ctrl Pts',(-0.0551438669093158,0.121384792244111,
3.01033982207094));
#31082=CARTESIAN_POINT('Ctrl Pts',(-0.0940937603166274,0.0944535765089676,
3.01297223357955));
#31083=CARTESIAN_POINT('Ctrl Pts',(-0.112940108892359,0.0573194028051013,
3.01560464508816));
#31084=CARTESIAN_POINT('Ctrl Pts',(-0.121859038434214,0.039745861833548,
3.01685041917942));
#31085=CARTESIAN_POINT('Ctrl Pts',(-0.126275572181929,0.0198872634041666,
3.01809619327068));
#31086=CARTESIAN_POINT('Ctrl Pts',(-0.126250113253048,1.79623087654263E-5,
3.01934196736194));
#31087=CARTESIAN_POINT('Origin',(0.,0.,3.1));
#31088=CARTESIAN_POINT('',(-0.126496969333234,-0.000107906771987382,3.06934196736194));
#31089=CARTESIAN_POINT('',(-0.126645757366777,2.69067085927681E-5,3.05565803263806));
#31090=CARTESIAN_POINT('',(-0.12645,1.54856587752183E-17,3.1));
#31091=CARTESIAN_POINT('Ctrl Pts',(-0.126645757366777,2.69067085927681E-5,
3.05565803263806));
#31092=CARTESIAN_POINT('Ctrl Pts',(-0.126650109530876,0.00151667558283516,
3.05556387297957));
#31093=CARTESIAN_POINT('Ctrl Pts',(-0.126626072178,0.00300630074643505,
3.05546971332109));
#31094=CARTESIAN_POINT('Ctrl Pts',(-0.126573208557277,0.0044949022237674,
3.0553755536626));
#31095=CARTESIAN_POINT('Ctrl Pts',(-0.125095305962741,0.0461115746257868,
3.05274314215399));
#31096=CARTESIAN_POINT('Ctrl Pts',(-0.10108714199637,0.0869281462553232,
3.05011073064538));
#31097=CARTESIAN_POINT('Ctrl Pts',(-0.0654319685934297,0.108441868097491,
3.04747831913677));
#31098=CARTESIAN_POINT('Ctrl Pts',(-0.0297767951904896,0.129955589939659,
3.04484590762816));
#31099=CARTESIAN_POINT('Ctrl Pts',(0.0175253876490204,0.132166461994459,
3.04221349611954));
#31100=CARTESIAN_POINT('Ctrl Pts',(0.0550318084723819,0.114072263617167,
3.03958108461093));
#31101=CARTESIAN_POINT('Ctrl Pts',(0.092538229295744,0.095978065239874,
3.03694867310232));
#31102=CARTESIAN_POINT('Ctrl Pts',(0.120248888102957,0.0575787964304887,
3.03431626159371));
#31103=CARTESIAN_POINT('Ctrl Pts',(0.125602137884551,0.0162814074734155,
3.0316838500851));
#31104=CARTESIAN_POINT('Ctrl Pts',(0.130955387666146,-0.0250159814836577,
3.02905143857648));
#31105=CARTESIAN_POINT('Ctrl Pts',(0.113951228422121,-0.0692114905884188,
3.02641902706787));
#31106=CARTESIAN_POINT('Ctrl Pts',(0.0822978942873024,-0.0962706490388489,
3.02378661555926));
#31107=CARTESIAN_POINT('Ctrl Pts',(0.0506445601524839,-0.123329807489279,
3.02115420405065));
#31108=CARTESIAN_POINT('Ctrl Pts',(0.00434205112687179,-0.133252615285378,
3.01852179254204));
#31109=CARTESIAN_POINT('Ctrl Pts',(-0.0356200281006283,-0.121540918494949,
3.01588938103343));
#31110=CARTESIAN_POINT('Ctrl Pts',(-0.0755821073281284,-0.10982922170452,
3.01325696952481));
#31111=CARTESIAN_POINT('Ctrl Pts',(-0.109203756757516,-0.0764830203275614,
3.0106245580162));
#31112=CARTESIAN_POINT('Ctrl Pts',(-0.121243790859916,-0.0366186352613279,
3.00799214650759));
#31113=CARTESIAN_POINT('Ctrl Pts',(-0.124802354366684,-0.0248362810993748,
3.00721410855108));
#31114=CARTESIAN_POINT('Ctrl Pts',(-0.126475628781476,-0.012484522820876,
3.00643607059457));
#31115=CARTESIAN_POINT('Ctrl Pts',(-0.126375290424941,-0.000106230050797054,
3.00565803263806));
#31116=CARTESIAN_POINT('Ctrl Pts',(-0.126250113253048,1.79623087654263E-5,
3.01934196736194));
#31117=CARTESIAN_POINT('Ctrl Pts',(-0.126221775608494,-0.0220980188702133,
3.0207286047793));
#31118=CARTESIAN_POINT('Ctrl Pts',(-0.120690113995694,-0.0442272599176159,
3.02211524219665));
#31119=CARTESIAN_POINT('Ctrl Pts',(-0.109738425578795,-0.063233377942656,
3.023501879614));
#31120=CARTESIAN_POINT('Ctrl Pts',(-0.0889475899453455,-0.0993148533139586,
3.02613429112261));
#31121=CARTESIAN_POINT('Ctrl Pts',(-0.0486231149342947,-0.124140672383972,
3.02876670263122));
#31122=CARTESIAN_POINT('Ctrl Pts',(-0.00704467496461261,-0.126456928197685,
3.03139911413984));
#31123=CARTESIAN_POINT('Ctrl Pts',(0.0345337650050683,-0.128773184011397,
3.03403152564845));
#31124=CARTESIAN_POINT('Ctrl Pts',(0.0773661699333803,-0.108579876568808,
3.03666393715706));
#31125=CARTESIAN_POINT('Ctrl Pts',(0.102035984081992,-0.0750309275363891,
3.03929634866567));
#31126=CARTESIAN_POINT('Ctrl Pts',(0.126705798230605,-0.0414819785039689,
3.04192876017428));
#31127=CARTESIAN_POINT('Ctrl Pts',(0.133213021599516,0.00542261211828284,
3.0445611716829));
#31128=CARTESIAN_POINT('Ctrl Pts',(0.118607834643087,0.0444203072460051,
3.04719358319151));
#31129=CARTESIAN_POINT('Ctrl Pts',(0.104002647686659,0.0834180023737263,
3.04982599470012));
#31130=CARTESIAN_POINT('Ctrl Pts',(0.0682850504048921,0.114508802006919,
3.05245840620873));
#31131=CARTESIAN_POINT('Ctrl Pts',(0.0276463521492325,0.123598791852477,
3.05509081771734));
#31132=CARTESIAN_POINT('Ctrl Pts',(-0.0129923461064282,0.132688781698037,
3.05772322922596));
#31133=CARTESIAN_POINT('Ctrl Pts',(-0.0585521453359818,0.119777961755961,
3.06035564073457));
#31134=CARTESIAN_POINT('Ctrl Pts',(-0.0883801220659878,0.0907189955750862,
3.06298805224318));
#31135=CARTESIAN_POINT('Ctrl Pts',(-0.112378957568068,0.0673388865067503,
3.06510602394943));
#31136=CARTESIAN_POINT('Ctrl Pts',(-0.126193947985427,0.0335054291562246,
3.06722399565569));
#31137=CARTESIAN_POINT('Ctrl Pts',(-0.126496969333234,-0.000107906771987382,
3.06934196736194));
#31138=CARTESIAN_POINT('Origin',(0.,0.,3.1));
#31139=CARTESIAN_POINT('',(-0.126566979141993,8.83287276302464E-5,3.11934196736194));
#31140=CARTESIAN_POINT('',(-0.126304742691185,8.06358209441624E-5,3.10565803263806));
#31141=CARTESIAN_POINT('',(-0.12645,1.54856587752183E-17,3.1));
#31142=CARTESIAN_POINT('Ctrl Pts',(-0.126304742691185,8.06358209441624E-5,
3.10565803263806));
#31143=CARTESIAN_POINT('Ctrl Pts',(-0.12639574781383,0.0154767095828029,
3.10469167536458));
#31144=CARTESIAN_POINT('Ctrl Pts',(-0.123787659959305,0.0308430184790688,
3.1037253180911));
#31145=CARTESIAN_POINT('Ctrl Pts',(-0.118340823679398,0.0451268292855474,
3.10275896081762));
#31146=CARTESIAN_POINT('Ctrl Pts',(-0.103503335617549,0.0840367324711176,
3.10012654930901));
#31147=CARTESIAN_POINT('Ctrl Pts',(-0.0676009656676162,0.114913977953889,
3.09749413780039));
#31148=CARTESIAN_POINT('Ctrl Pts',(-0.0269087833345171,0.123761458661173,
3.09486172629178));
#31149=CARTESIAN_POINT('Ctrl Pts',(0.0137833989985814,0.132608939368457,
3.09222931478317));
#31150=CARTESIAN_POINT('Ctrl Pts',(0.0592653937148459,0.119426655300253,
3.08959690327456));
#31151=CARTESIAN_POINT('Ctrl Pts',(0.0889195472648929,0.0901903286649502,
3.08696449176595));
#31152=CARTESIAN_POINT('Ctrl Pts',(0.11857370081494,0.0609540020296468,
3.08433208025733));
#31153=CARTESIAN_POINT('Ctrl Pts',(0.13240001319877,0.015663632827244,3.08169966874872));
#31154=CARTESIAN_POINT('Ctrl Pts',(0.124130814751194,-0.0251499920415489,
3.07906725724011));
#31155=CARTESIAN_POINT('Ctrl Pts',(0.115861616303618,-0.0659636169103418,
3.0764348457315));
#31156=CARTESIAN_POINT('Ctrl Pts',(0.085496907024637,-0.102300497445525,
3.07380243422289));
#31157=CARTESIAN_POINT('Ctrl Pts',(0.0468014538280004,-0.117688594137541,
3.07117002271428));
#31158=CARTESIAN_POINT('Ctrl Pts',(0.0081060006313637,-0.133076690829557,
3.06853761120566));
#31159=CARTESIAN_POINT('Ctrl Pts',(-0.0389201964829282,-0.127516003678407,
3.06590519969705));
#31160=CARTESIAN_POINT('Ctrl Pts',(-0.0729594744287227,-0.103527273515581,
3.06327278818844));
#31161=CARTESIAN_POINT('Ctrl Pts',(-0.105781189400045,-0.0803966047281269,
3.06073453633831));
#31162=CARTESIAN_POINT('Ctrl Pts',(-0.12652843654431,-0.0401326336098284,
3.05819628448819));
#31163=CARTESIAN_POINT('Ctrl Pts',(-0.126645757366777,2.69067085927681E-5,
3.05565803263806));
#31164=CARTESIAN_POINT('Ctrl Pts',(-0.126496969333234,-0.000107906771987382,
3.06934196736194));
#31165=CARTESIAN_POINT('Ctrl Pts',(-0.126570570997419,-0.00827233967750279,
3.0698564071643));
#31166=CARTESIAN_POINT('Ctrl Pts',(-0.125847009061939,-0.0164237861126916,
3.07037084696666));
#31167=CARTESIAN_POINT('Ctrl Pts',(-0.124278591835651,-0.0244092963007763,
3.07088528676901));
#31168=CARTESIAN_POINT('Ctrl Pts',(-0.116252930644851,-0.0652715095760922,
3.07351769827763));
#31169=CARTESIAN_POINT('Ctrl Pts',(-0.0861054540327919,-0.101788823707051,
3.07615010978624));
#31170=CARTESIAN_POINT('Ctrl Pts',(-0.0475024541674668,-0.117407405995615,
3.07878252129485));
#31171=CARTESIAN_POINT('Ctrl Pts',(-0.00889945430214065,-0.133025988284179,
3.08141493280346));
#31172=CARTESIAN_POINT('Ctrl Pts',(0.0381590688164514,-0.127745838730347,
3.08404734431207));
#31173=CARTESIAN_POINT('Ctrl Pts',(0.072340798251519,-0.103960526368831,
3.08667975582068));
#31174=CARTESIAN_POINT('Ctrl Pts',(0.106522527686585,-0.0801752140073166,
3.0893121673293));
#31175=CARTESIAN_POINT('Ctrl Pts',(0.127827463438127,-0.0378847388381192,
3.09194457883791));
#31176=CARTESIAN_POINT('Ctrl Pts',(0.1265977664655,0.00374000808798695,
3.09457699034652));
#31177=CARTESIAN_POINT('Ctrl Pts',(0.125368069492872,0.0453647550140949,
3.09720940185513));
#31178=CARTESIAN_POINT('Ctrl Pts',(0.101603739796073,0.0863237736971122,
3.09984181336374));
#31179=CARTESIAN_POINT('Ctrl Pts',(0.066077495668981,0.108049741788989,
3.10247422487236));
#31180=CARTESIAN_POINT('Ctrl Pts',(0.0305512515418895,0.129775709880865,
3.10510663638097));
#31181=CARTESIAN_POINT('Ctrl Pts',(-0.0167369070154944,0.132268627381602,
3.10773904788958));
#31182=CARTESIAN_POINT('Ctrl Pts',(-0.0543505659626984,0.114398418319861,
3.11037145939819));
#31183=CARTESIAN_POINT('Ctrl Pts',(-0.0919642249099026,0.096528209258119,
3.1130038709068));
#31184=CARTESIAN_POINT('Ctrl Pts',(-0.119903384246927,0.0582948736338987,
3.11563628241541));
#31185=CARTESIAN_POINT('Ctrl Pts',(-0.125502814331461,0.0170301417913753,
3.11826869392403));
#31186=CARTESIAN_POINT('Ctrl Pts',(-0.126263804720884,0.011422059561536,
3.11862645173666));
#31187=CARTESIAN_POINT('Ctrl Pts',(-0.126612176704445,0.00575798695415024,
3.1189842095493));
#31188=CARTESIAN_POINT('Ctrl Pts',(-0.126566979141993,8.83287276302464E-5,
3.11934196736194));
#31189=CARTESIAN_POINT('Origin',(0.,0.,3.1));
#31190=CARTESIAN_POINT('',(-0.126251310180948,2.19509288584552E-5,3.16934196736194));
#31191=CARTESIAN_POINT('',(-0.126368593930883,-0.000104790611567188,3.15565803263806));
#31192=CARTESIAN_POINT('',(-0.12645,1.54856587752183E-17,3.1));
#31193=CARTESIAN_POINT('Ctrl Pts',(-0.126368593930883,-0.000104790611567188,
3.15565803263806));
#31194=CARTESIAN_POINT('Ctrl Pts',(-0.126135626550864,0.029149858613393,
3.15381947774958));
#31195=CARTESIAN_POINT('Ctrl Pts',(-0.116012034435359,0.0585500300902377,
3.15198092286111));
#31196=CARTESIAN_POINT('Ctrl Pts',(-0.0974287026581059,0.0809236008148654,
3.15014236797263));
#31197=CARTESIAN_POINT('Ctrl Pts',(-0.0708214054023045,0.112957697503196,
3.14750995646402));
#31198=CARTESIAN_POINT('Ctrl Pts',(-0.0268716218413343,0.130587246038798,
3.1448775449554));
#31199=CARTESIAN_POINT('Ctrl Pts',(0.014497568206441,0.125820514172312,
3.14224513344679));
#31200=CARTESIAN_POINT('Ctrl Pts',(0.0558667582542159,0.121053782305825,
3.13961272193818));
#31201=CARTESIAN_POINT('Ctrl Pts',(0.0946553547887964,0.0938907700372525,
3.13698031042957));
#31202=CARTESIAN_POINT('Ctrl Pts',(0.113279919572572,0.0566448681887155,
3.13434789892096));
#31203=CARTESIAN_POINT('Ctrl Pts',(0.131904484356347,0.0193989663401779,
3.13171548741235));
#31204=CARTESIAN_POINT('Ctrl Pts',(0.130365017389317,-0.0279298250883239,
3.12908307590374));
#31205=CARTESIAN_POINT('Ctrl Pts',(0.109359381568105,-0.0638866725814309,
3.12645066439512));
#31206=CARTESIAN_POINT('Ctrl Pts',(0.0883537457468925,-0.0998435200745383,
3.12381825288651));
#31207=CARTESIAN_POINT('Ctrl Pts',(0.0478819410714995,-0.12442842363225,
3.1211858413779));
#31208=CARTESIAN_POINT('Ctrl Pts',(0.00629042865298903,-0.126496686825572,
3.11855342986929));
#31209=CARTESIAN_POINT('Ctrl Pts',(-0.0353010837655206,-0.128564950018895,
3.11592101836068));
#31210=CARTESIAN_POINT('Ctrl Pts',(-0.0780123039271484,-0.108116572847827,
3.11328860685206));
#31211=CARTESIAN_POINT('Ctrl Pts',(-0.102481610921079,-0.0744211038181091,
3.11065619534345));
#31212=CARTESIAN_POINT('Ctrl Pts',(-0.117968244532349,-0.0530952287799418,
3.10899014110832));
#31213=CARTESIAN_POINT('Ctrl Pts',(-0.12614784474654,-0.0264630603867145,
3.10732408687319));
#31214=CARTESIAN_POINT('Ctrl Pts',(-0.126304742691185,8.06358209441624E-5,
3.10565803263806));
#31215=CARTESIAN_POINT('Ctrl Pts',(-0.126566979141993,8.83287276302464E-5,
3.11934196736194));
#31216=CARTESIAN_POINT('Ctrl Pts',(-0.126279609310085,-0.0359598261533815,
3.12161662105791));
#31217=CARTESIAN_POINT('Ctrl Pts',(-0.110082106605306,-0.0722337808796859,
3.12389127475389));
#31218=CARTESIAN_POINT('Ctrl Pts',(-0.0828705393299942,-0.0957781595443726,
3.12616592844986));
#31219=CARTESIAN_POINT('Ctrl Pts',(-0.0513791334119502,-0.12302560097677,
3.12879833995848));
#31220=CARTESIAN_POINT('Ctrl Pts',(-0.00513662074381884,-0.133224355780737,
3.13143075146709));
#31221=CARTESIAN_POINT('Ctrl Pts',(0.034894591212013,-0.121751179208655,
3.1340631629757));
#31222=CARTESIAN_POINT('Ctrl Pts',(0.0749258031678458,-0.110278002636571,
3.13669557448431));
#31223=CARTESIAN_POINT('Ctrl Pts',(0.108745714411378,-0.0771328946884361,
3.13932798599292));
#31224=CARTESIAN_POINT('Ctrl Pts',(0.12102326443306,-0.0373410176684702,
3.14196039750153));
#31225=CARTESIAN_POINT('Ctrl Pts',(0.133300814454742,0.00245085935149471,
3.14459280901015));
#31226=CARTESIAN_POINT('Ctrl Pts',(0.124036003254574,0.0488895054432904,
3.14722522051876));
#31227=CARTESIAN_POINT('Ctrl Pts',(0.097428705282154,0.0809236029943958,
3.14985763202737));
#31228=CARTESIAN_POINT('Ctrl Pts',(0.0708214073097326,0.112957700545502,
3.15249004353598));
#31229=CARTESIAN_POINT('Ctrl Pts',(0.0268716225650577,0.130587249555918,
3.15512245504459));
#31230=CARTESIAN_POINT('Ctrl Pts',(-0.0144975685969178,0.125820517561044,
3.15775486655321));
#31231=CARTESIAN_POINT('Ctrl Pts',(-0.0558667597588919,0.121053785566171,
3.16038727806182));
#31232=CARTESIAN_POINT('Ctrl Pts',(-0.0946553573381664,0.0938907725660106,
3.16301968957043));
#31233=CARTESIAN_POINT('Ctrl Pts',(-0.113279922623555,0.0566448697143249,
3.16565210107904));
#31234=CARTESIAN_POINT('Ctrl Pts',(-0.121981975887314,0.039242271290916,
3.16688205650667));
#31235=CARTESIAN_POINT('Ctrl Pts',(-0.126282044039751,0.0196384895744722,
3.16811201193431));
#31236=CARTESIAN_POINT('Ctrl Pts',(-0.126251310180948,2.19509288584552E-5,
3.16934196736194));
#31237=CARTESIAN_POINT('Origin',(0.,0.,3.1));
#31238=CARTESIAN_POINT('',(-0.126489518850073,-0.000109039769437509,3.21934196736194));
#31239=CARTESIAN_POINT('',(-0.126647930997008,2.24668189870201E-5,3.20565803263806));
#31240=CARTESIAN_POINT('',(-0.12645,1.54856587752183E-17,3.1));
#31241=CARTESIAN_POINT('Ctrl Pts',(-0.126647930997008,2.24668189870201E-5,
3.20565803263806));
#31242=CARTESIAN_POINT('Ctrl Pts',(-0.126650996831423,0.00126189995630808,
3.2055796916432));
#31243=CARTESIAN_POINT('Ctrl Pts',(-0.126634359036856,0.00250124877863209,
3.20550135064834));
#31244=CARTESIAN_POINT('Ctrl Pts',(-0.126597763055832,0.00374000798724603,
3.20542300965348));
#31245=CARTESIAN_POINT('Ctrl Pts',(-0.125368066116328,0.0453647537922705,
3.20279059814487));
#31246=CARTESIAN_POINT('Ctrl Pts',(-0.10160373705958,0.0863237713721372,
3.20015818663626));
#31247=CARTESIAN_POINT('Ctrl Pts',(-0.0660774938893213,0.10804973887887,
3.19752577512764));
#31248=CARTESIAN_POINT('Ctrl Pts',(-0.0305512507190632,0.129775706385603,
3.19489336361903));
#31249=CARTESIAN_POINT('Ctrl Pts',(0.0167369065647044,0.132268623819202,
3.19226095211042));
#31250=CARTESIAN_POINT('Ctrl Pts',(0.0543505644988585,0.114398415238764,
3.18962854060181));
#31251=CARTESIAN_POINT('Ctrl Pts',(0.091964222433013,0.0965282066583261,
3.1869961290932));
#31252=CARTESIAN_POINT('Ctrl Pts',(0.119903381017553,0.0582948720638503,
3.18436371758459));
#31253=CARTESIAN_POINT('Ctrl Pts',(0.125502810951281,0.0170301413327138,
3.18173130607597));
#31254=CARTESIAN_POINT('Ctrl Pts',(0.13110224088501,-0.0242345893984227,
3.17909889456736));
#31255=CARTESIAN_POINT('Ctrl Pts',(0.114361942167926,-0.0685307162662204,
3.17646648305875));
#31256=CARTESIAN_POINT('Ctrl Pts',(0.0828705370980449,-0.0957781569647633,
3.17383407155014));
#31257=CARTESIAN_POINT('Ctrl Pts',(0.0513791320281642,-0.123025597663306,
3.17120166004152));
#31258=CARTESIAN_POINT('Ctrl Pts',(0.00513662060548718,-0.133224352192594,
3.16856924853291));
#31259=CARTESIAN_POINT('Ctrl Pts',(-0.0348945902721819,-0.121751175929524,
3.1659368370243));
#31260=CARTESIAN_POINT('Ctrl Pts',(-0.0749258011498519,-0.110277999666453,
3.16330442551569));
#31261=CARTESIAN_POINT('Ctrl Pts',(-0.108745711482513,-0.0771328926110206,
3.16067201400708));
#31262=CARTESIAN_POINT('Ctrl Pts',(-0.121023261173527,-0.0373410166627737,
3.15803960249846));
#31263=CARTESIAN_POINT('Ctrl Pts',(-0.124725803146683,-0.0253409763781187,
3.15724574587833));
#31264=CARTESIAN_POINT('Ctrl Pts',(-0.126469185269255,-0.0127364488245176,
3.15645188925819));
#31265=CARTESIAN_POINT('Ctrl Pts',(-0.126368593930883,-0.000104790611567188,
3.15565803263806));
#31266=CARTESIAN_POINT('Ctrl Pts',(-0.126251310180948,2.19509288584552E-5,
3.16934196736194));
#31267=CARTESIAN_POINT('Ctrl Pts',(-0.126216265913324,-0.0223457977660937,
3.17074442344292));
#31268=CARTESIAN_POINT('Ctrl Pts',(-0.120550447304899,-0.0447301326243598,
3.1721468795239));
#31269=CARTESIAN_POINT('Ctrl Pts',(-0.109359384513483,-0.0638866743021069,
3.17354933560488));
#31270=CARTESIAN_POINT('Ctrl Pts',(-0.0883537481265213,-0.0998435227636405,
3.17618174711349));
#31271=CARTESIAN_POINT('Ctrl Pts',(-0.0478819423610949,-0.124428426983496,
3.1788141586221));
#31272=CARTESIAN_POINT('Ctrl Pts',(-0.00629042882239688,-0.126496690232519,
3.18144657013071));
#31273=CARTESIAN_POINT('Ctrl Pts',(0.0353010847163008,-0.128564953481541,
3.18407898163933));
#31274=CARTESIAN_POINT('Ctrl Pts',(0.0780123060282702,-0.108116575759732,
3.18671139314794));
#31275=CARTESIAN_POINT('Ctrl Pts',(0.102481613681232,-0.0744211058224891,
3.18934380465655));
#31276=CARTESIAN_POINT('Ctrl Pts',(0.126950921334194,-0.040725635885246,
3.19197621616516));
#31277=CARTESIAN_POINT('Ctrl Pts',(0.133178315328148,0.00621692626743081,
3.19460862767377));
#31278=CARTESIAN_POINT('Ctrl Pts',(0.118340826866677,0.0451268305009631,
3.19724103918239));
#31279=CARTESIAN_POINT('Ctrl Pts',(0.103503338405205,0.0840367347344954,
3.199873450691));
#31280=CARTESIAN_POINT('Ctrl Pts',(0.0676009674883078,0.114913981048883,
3.20250586219961));
#31281=CARTESIAN_POINT('Ctrl Pts',(0.026908784059242,0.123761461994453,
3.20513827370822));
#31282=CARTESIAN_POINT('Ctrl Pts',(-0.0137833993698235,0.132608942940023,
3.20777068521683));
#31283=CARTESIAN_POINT('Ctrl Pts',(-0.0592653953110574,0.119426658516775,
3.21040309672544));
#31284=CARTESIAN_POINT('Ctrl Pts',(-0.0889195496597795,0.0901903310940448,
3.21303550823405));
#31285=CARTESIAN_POINT('Ctrl Pts',(-0.11260033459284,0.0668432083338218,
3.21513766127668));
#31286=CARTESIAN_POINT('Ctrl Pts',(-0.126187596109782,0.0332583119648893,
3.21723981431931));
#31287=CARTESIAN_POINT('Ctrl Pts',(-0.126489518850073,-0.000109039769437509,
3.21934196736194));
#31288=CARTESIAN_POINT('Origin',(0.,0.,3.1));
#31289=CARTESIAN_POINT('',(-0.126573425356775,8.55484528903966E-5,3.26934196736194));
#31290=CARTESIAN_POINT('',(-0.126309785017077,8.34376343069358E-5,3.25565803263806));
#31291=CARTESIAN_POINT('',(-0.12645,1.54856587752183E-17,3.1));
#31292=CARTESIAN_POINT('Ctrl Pts',(-0.126309785017077,8.34376343069358E-5,
3.25565803263806));
#31293=CARTESIAN_POINT('Ctrl Pts',(-0.126402648710969,0.0152259667938181,
3.2547074940282));
#31294=CARTESIAN_POINT('Ctrl Pts',(-0.123881624579711,0.0303386118332616,
3.25375695541835));
#31295=CARTESIAN_POINT('Ctrl Pts',(-0.118607831448617,0.0444203060496175,
3.25280641680849));
#31296=CARTESIAN_POINT('Ctrl Pts',(-0.104002644885555,0.0834180001270126,
3.25017400529988));
#31297=CARTESIAN_POINT('Ctrl Pts',(-0.0682850485657758,0.114508798922838,
3.24754159379127));
#31298=CARTESIAN_POINT('Ctrl Pts',(-0.0276463514046418,0.123598788523579,
3.24490918228266));
#31299=CARTESIAN_POINT('Ctrl Pts',(0.0129923457564923,0.13268877812432,
3.24227677077404));
#31300=CARTESIAN_POINT('Ctrl Pts',(0.0585521437589804,0.119777958529977,
3.23964435926544));
#31301=CARTESIAN_POINT('Ctrl Pts',(0.0883801196856296,0.090718993131753,
3.23701194775682));
#31302=CARTESIAN_POINT('Ctrl Pts',(0.118208095612278,0.0616600277335293,
3.23437953624821));
#31303=CARTESIAN_POINT('Ctrl Pts',(0.132304249463088,0.0164529165314243,
3.2317471247396));
#31304=CARTESIAN_POINT('Ctrl Pts',(0.124278588488448,-0.024409295643347,
3.22911471323098));
#31305=CARTESIAN_POINT('Ctrl Pts',(0.116252927513807,-0.0652715078181186,
3.22648230172237));
#31306=CARTESIAN_POINT('Ctrl Pts',(0.0861054517137156,-0.101788820965557,
3.22384989021376));
#31307=CARTESIAN_POINT('Ctrl Pts',(0.0475024528880895,-0.117407402833467,
3.22121747870515));
#31308=CARTESIAN_POINT('Ctrl Pts',(0.00889945406246312,-0.133025984701378,
3.21858506719654));
#31309=CARTESIAN_POINT('Ctrl Pts',(-0.0381590677886978,-0.127745835289761,
3.21595265568793));
#31310=CARTESIAN_POINT('Ctrl Pts',(-0.0723407963031478,-0.103960523568861,
3.21332024417931));
#31311=CARTESIAN_POINT('Ctrl Pts',(-0.105505271014729,-0.0808830665952798,
3.21076617366556));
#31312=CARTESIAN_POINT('Ctrl Pts',(-0.126547978765194,-0.0403854911787608,
3.20821210315181));
#31313=CARTESIAN_POINT('Ctrl Pts',(-0.126647930997008,2.24668189870201E-5,
3.20565803263806));
#31314=CARTESIAN_POINT('Ctrl Pts',(-0.126489518850073,-0.000109039769437509,
3.21934196736194));
#31315=CARTESIAN_POINT('Ctrl Pts',(-0.126565677476903,-0.00852580124482262,
3.21987222582793));
#31316=CARTESIAN_POINT('Ctrl Pts',(-0.125796519899578,-0.0169287208447501,
3.22040248429391));
#31317=CARTESIAN_POINT('Ctrl Pts',(-0.124130818094417,-0.0251499927189283,
3.22093274275989));
#31318=CARTESIAN_POINT('Ctrl Pts',(-0.115861619424122,-0.065963618686957,
3.2235651542685));
#31319=CARTESIAN_POINT('Ctrl Pts',(-0.0854969093273219,-0.102300500200801,
3.22619756577711));
#31320=CARTESIAN_POINT('Ctrl Pts',(-0.0468014550884958,-0.117688597307262,
3.22882997728573));
#31321=CARTESIAN_POINT('Ctrl Pts',(-0.00810600084966979,-0.133076694413723,
3.23146238879434));
#31322=CARTESIAN_POINT('Ctrl Pts',(0.038920197531182,-0.127516007112802,
3.23409480030295));
#31323=CARTESIAN_POINT('Ctrl Pts',(0.0729594763937567,-0.103527276303882,
3.23672721181156));
#31324=CARTESIAN_POINT('Ctrl Pts',(0.106998755256331,-0.0795385454949616,
3.23935962332018));
#31325=CARTESIAN_POINT('Ctrl Pts',(0.128051114600629,-0.0371217711780427,
3.24199203482878));
#31326=CARTESIAN_POINT('Ctrl Pts',(0.126573211966284,0.00449490234484176,
3.2446244463374));
#31327=CARTESIAN_POINT('Ctrl Pts',(0.125095309331938,0.0461115758677259,
3.24725685784601));
#31328=CARTESIAN_POINT('Ctrl Pts',(0.10108714471895,0.0869281485965757,
3.24988926935462));
#31329=CARTESIAN_POINT('Ctrl Pts',(0.0654319703557041,0.108441871018171,
3.25252168086323));
#31330=CARTESIAN_POINT('Ctrl Pts',(0.0297767959924581,0.129955593439766,
3.25515409237185));
#31331=CARTESIAN_POINT('Ctrl Pts',(-0.0175253881210462,0.132166465554107,
3.25778650388046));
#31332=CARTESIAN_POINT('Ctrl Pts',(-0.0550318099545696,0.114072266689479,
3.26041891538907));
#31333=CARTESIAN_POINT('Ctrl Pts',(-0.0925382317880931,0.09597806782485,
3.26305132689768));
#31334=CARTESIAN_POINT('Ctrl Pts',(-0.120248891341636,0.0575787979812516,
3.26568373840629));
#31335=CARTESIAN_POINT('Ctrl Pts',(-0.125602141267406,0.0162814079119122,
3.26831614991491));
#31336=CARTESIAN_POINT('Ctrl Pts',(-0.126297505847784,0.0109170511726472,
3.26865808906392));
#31337=CARTESIAN_POINT('Ctrl Pts',(-0.126615635779588,0.00550379470022512,
3.26900002821293));
#31338=CARTESIAN_POINT('Ctrl Pts',(-0.126573425356775,8.55484528903966E-5,
3.26934196736194));
#31339=CARTESIAN_POINT('Origin',(0.,0.,3.1));
#31340=CARTESIAN_POINT('',(-0.126252746279467,2.59119664437757E-5,3.31934196736194));
#31341=CARTESIAN_POINT('',(-0.126362016509238,-0.00010321110317447,3.30565803263806));
#31342=CARTESIAN_POINT('',(-0.12645,1.54856587752183E-17,3.1));
#31343=CARTESIAN_POINT('Ctrl Pts',(-0.126362016509238,-0.00010321110317447,
3.30565803263806));
#31344=CARTESIAN_POINT('Ctrl Pts',(-0.126135404540093,0.0289035586789932,
3.30383529641321));
#31345=CARTESIAN_POINT('Ctrl Pts',(-0.116200394811108,0.0580506048820654,
3.30201256018836));
#31346=CARTESIAN_POINT('Ctrl Pts',(-0.0979095549055491,0.080341149659951,
3.30018982396351));
#31347=CARTESIAN_POINT('Ctrl Pts',(-0.0714937648350404,0.112533348293265,
3.2975574124549));
#31348=CARTESIAN_POINT('Ctrl Pts',(-0.0276498958846022,0.130424676138957,
3.29492500094628));
#31349=CARTESIAN_POINT('Ctrl Pts',(0.0137469847697539,0.125904732556904,
3.29229258943767));
#31350=CARTESIAN_POINT('Ctrl Pts',(0.05514386542411,0.12138478897485,3.28966017792906));
#31351=CARTESIAN_POINT('Ctrl Pts',(0.0940937577823839,0.0944535739650504,
3.28702776642045));
#31352=CARTESIAN_POINT('Ctrl Pts',(0.112940105850529,0.057319401261323,
3.28439535491184));
#31353=CARTESIAN_POINT('Ctrl Pts',(0.131786453918674,0.0201852285575958,
3.28176294340322));
#31354=CARTESIAN_POINT('Ctrl Pts',(0.13052925769669,-0.0271519018400594,
3.27913053189461));
#31355=CARTESIAN_POINT('Ctrl Pts',(0.109738422623206,-0.0632333762395775,
3.276498120386));
#31356=CARTESIAN_POINT('Ctrl Pts',(0.0889475875497212,-0.099314850639096,
3.27386570887739));
#31357=CARTESIAN_POINT('Ctrl Pts',(0.0486231136247353,-0.124140669040477,
3.27123329736878));
#31358=CARTESIAN_POINT('Ctrl Pts',(0.00704467477488957,-0.126456924791809,
3.26860088586016));
#31359=CARTESIAN_POINT('Ctrl Pts',(-0.0345337640749562,-0.128773180543141,
3.26596847435155));
#31360=CARTESIAN_POINT('Ctrl Pts',(-0.0773661678496626,-0.108579873644424,
3.26333606284294));
#31361=CARTESIAN_POINT('Ctrl Pts',(-0.102035981333843,-0.0750309255155824,
3.26070365133433));
#31362=CARTESIAN_POINT('Ctrl Pts',(-0.117797761200207,-0.0535961815725874,
3.25902177843557));
#31363=CARTESIAN_POINT('Ctrl Pts',(-0.126145472985543,-0.026709592283637,
3.25733990553681));
#31364=CARTESIAN_POINT('Ctrl Pts',(-0.126309785017077,8.34376343069358E-5,
3.25565803263806));
#31365=CARTESIAN_POINT('Ctrl Pts',(-0.126573425356775,8.55484528903966E-5,
3.26934196736194));
#31366=CARTESIAN_POINT('Ctrl Pts',(-0.126290679707385,-0.0362084626390545,
3.27163243972154));
#31367=CARTESIAN_POINT('Ctrl Pts',(-0.109839596819478,-0.0727263630692267,
3.27392291208114));
#31368=CARTESIAN_POINT('Ctrl Pts',(-0.0822978965038287,-0.0962706516317226,
3.27621338444074));
#31369=CARTESIAN_POINT('Ctrl Pts',(-0.0506445615164858,-0.123329810810936,
3.27884579594935));
#31370=CARTESIAN_POINT('Ctrl Pts',(-0.00434205124380389,-0.133252618874282,
3.28147820745796));
#31371=CARTESIAN_POINT('Ctrl Pts',(0.0356200290599969,-0.121540921768417,
3.28411061896657));
#31372=CARTESIAN_POINT('Ctrl Pts',(0.0755821093637979,-0.109829224662552,
3.28674303047519));
#31373=CARTESIAN_POINT('Ctrl Pts',(0.109203759698717,-0.0764830223874748,
3.2893754419838));
#31374=CARTESIAN_POINT('Ctrl Pts',(0.121243794125388,-0.0366186362475693,
3.29200785349241));
#31375=CARTESIAN_POINT('Ctrl Pts',(0.133283828552059,0.00324574989233616,
3.29464026500102));
#31376=CARTESIAN_POINT('Ctrl Pts',(0.123742247070482,0.0496283198970706,
3.29727267650964));
#31377=CARTESIAN_POINT('Ctrl Pts',(0.0969443881476166,0.0815031762647041,
3.29990508801825));
#31378=CARTESIAN_POINT('Ctrl Pts',(0.0701465292247518,0.113378032632337,
3.30253749952686));
#31379=CARTESIAN_POINT('Ctrl Pts',(0.0260923928606002,0.130745175362871,
3.30516991103547));
#31380=CARTESIAN_POINT('Ctrl Pts',(-0.0152476364742436,0.125731824597042,
3.30780232254408));
#31381=CARTESIAN_POINT('Ctrl Pts',(-0.0565876658090873,0.120718473831214,
3.31043473405269));
#31382=CARTESIAN_POINT('Ctrl Pts',(-0.095213588114623,0.0933246295690233,
3.31306714556131));
#31383=CARTESIAN_POINT('Ctrl Pts',(-0.113615707760984,0.0559683221521016,
3.31569955706992));
#31384=CARTESIAN_POINT('Ctrl Pts',(-0.122103244730499,0.0387386200124153,
3.31691369383393));
#31385=CARTESIAN_POINT('Ctrl Pts',(-0.12628858288157,0.0193896083672227,
3.31812783059793));
#31386=CARTESIAN_POINT('Ctrl Pts',(-0.126252746279467,2.59119664437757E-5,
3.31934196736194));
#31387=CARTESIAN_POINT('Origin',(0.,0.,3.1));
#31388=CARTESIAN_POINT('',(-0.126482040448775,-0.000110013702131137,3.36934196736194));
#31389=CARTESIAN_POINT('',(-0.126649735277799,1.79833793418055E-5,3.35565803263806));
#31390=CARTESIAN_POINT('',(-0.12645,1.54856587752183E-17,3.1));
#31391=CARTESIAN_POINT('Ctrl Pts',(-0.126649735277799,1.79833793418055E-5,
3.35565803263806));
#31392=CARTESIAN_POINT('Ctrl Pts',(-0.126651722007443,0.00100711151136191,
3.35559551030682));
#31393=CARTESIAN_POINT('Ctrl Pts',(-0.126641125668946,0.0019961959922384,
3.35553298797559));
#31394=CARTESIAN_POINT('Ctrl Pts',(-0.126617815335903,0.00298498074413288,
3.35547046564436));
#31395=CARTESIAN_POINT('Ctrl Pts',(-0.12563636778334,0.0446163196439928,
3.35283805413574));
#31396=CARTESIAN_POINT('Ctrl Pts',(-0.102116718771259,0.085716326541524,
3.35020564262713));
#31397=CARTESIAN_POINT('Ctrl Pts',(-0.0667206692597134,0.107653767068442,
3.34757323111852));
#31398=CARTESIAN_POINT('Ctrl Pts',(-0.0313246197481669,0.12959120759536,
3.34494081960991));
#31399=CARTESIAN_POINT('Ctrl Pts',(0.0159478302628458,0.132366081751665,
3.3423084081013));
#31400=CARTESIAN_POINT('Ctrl Pts',(0.0536673876466801,0.114720498489436,
3.33967599659268));
#31401=CARTESIAN_POINT('Ctrl Pts',(0.0913869450305144,0.0970749152272078,
3.33704358508407));
#31402=CARTESIAN_POINT('Ctrl Pts',(0.11955360978717,0.059008874546446,3.33441117357546));
#31403=CARTESIAN_POINT('Ctrl Pts',(0.12539902073952,0.0177782695461103,
3.33177876206685));
#31404=CARTESIAN_POINT('Ctrl Pts',(0.13124443169187,-0.0234523354542255,
3.32914635055824));
#31405=CARTESIAN_POINT('Ctrl Pts',(0.114768588839913,-0.0678475047741352,
3.32651393904963));
#31406=CARTESIAN_POINT('Ctrl Pts',(0.083440232769335,-0.0952822587152781,
3.32388152754101));
#31407=CARTESIAN_POINT('Ctrl Pts',(0.0521118766987572,-0.122717012656421,
3.3212491160324));
#31408=CARTESIAN_POINT('Ctrl Pts',(0.00593100740955835,-0.133191351218797,
3.31861670452379));
#31409=CARTESIAN_POINT('Ctrl Pts',(-0.0341679114813036,-0.121957103505662,
3.31598429301518));
#31410=CARTESIAN_POINT('Ctrl Pts',(-0.0742668303721658,-0.110722855792528,
3.31335188150657));
#31411=CARTESIAN_POINT('Ctrl Pts',(-0.108283798864691,-0.0777800218038817,
3.31071946999795));
#31412=CARTESIAN_POINT('Ctrl Pts',(-0.120798427515664,-0.0380620700990904,
3.30808705848934));
#31413=CARTESIAN_POINT('Ctrl Pts',(-0.124647668210362,-0.0258456503973156,
3.30727738320558));
#31414=CARTESIAN_POINT('Ctrl Pts',(-0.126462679516819,-0.0129882705177865,
3.30646770792182));
#31415=CARTESIAN_POINT('Ctrl Pts',(-0.126362016509238,-0.00010321110317447,
3.30565803263806));
#31416=CARTESIAN_POINT('Ctrl Pts',(-0.126252746279467,2.59119664437757E-5,
3.31934196736194));
#31417=CARTESIAN_POINT('Ctrl Pts',(-0.126210884316958,-0.0225934851076951,
3.32076024210655));
#31418=CARTESIAN_POINT('Ctrl Pts',(-0.120409070525885,-0.0452329200835406,
3.32217851685115));
#31419=CARTESIAN_POINT('Ctrl Pts',(-0.108976454281191,-0.064537698648537,
3.32359679159575));
#31420=CARTESIAN_POINT('Ctrl Pts',(-0.0877567641678496,-0.100368641460601,
3.32622920310437));
#31421=CARTESIAN_POINT('Ctrl Pts',(-0.047139066953979,-0.124711756513075,
3.32886161461298));
#31422=CARTESIAN_POINT('Ctrl Pts',(-0.00553595897255799,-0.126531953643381,
3.33149402612159));
#31423=CARTESIAN_POINT('Ctrl Pts',(0.0360671490088627,-0.128352150773687,
3.3341264376302));
#31424=CARTESIAN_POINT('Ctrl Pts',(0.0786556677578339,-0.107649429981826,
3.33675884913881));
#31425=CARTESIAN_POINT('Ctrl Pts',(0.102923598708863,-0.0738086374577052,
3.33939126064743));
#31426=CARTESIAN_POINT('Ctrl Pts',(0.127191529659892,-0.0399678449335842,
3.34202367215604));
#31427=CARTESIAN_POINT('Ctrl Pts',(0.133138872812978,0.00701101932279596,
3.34465608366465));
#31428=CARTESIAN_POINT('Ctrl Pts',(0.118069610514671,0.0458317489024548,
3.34728849517326));
#31429=CARTESIAN_POINT('Ctrl Pts',(0.103000348216365,0.0846524784821133,
3.34992090668187));
#31430=CARTESIAN_POINT('Ctrl Pts',(0.0669144804666656,0.11531507338505,
3.35255331819048));
#31431=CARTESIAN_POINT('Ctrl Pts',(0.0261702590074494,0.123919730785983,
3.3551857296991));
#31432=CARTESIAN_POINT('Ctrl Pts',(-0.0145739624517671,0.132524388186917,
3.35781814120771));
#31433=CARTESIAN_POINT('Ctrl Pts',(-0.059976537620501,0.119071108085846,
3.36045055271632));
#31434=CARTESIAN_POINT('Ctrl Pts',(-0.0894558149920353,0.0896584591581523,
3.36308296422493));
#31435=CARTESIAN_POINT('Ctrl Pts',(-0.112819802593213,0.0663472783512584,
3.36516929860394));
#31436=CARTESIAN_POINT('Ctrl Pts',(-0.126181642003826,0.033011291498231,
3.36725563298294));
#31437=CARTESIAN_POINT('Ctrl Pts',(-0.126482040448775,-0.000110013702131137,
3.36934196736194));
#31438=CARTESIAN_POINT('Origin',(0.,0.,3.1));
#31439=CARTESIAN_POINT('',(-0.126579711874066,8.26312290282544E-5,3.41934196736194));
#31440=CARTESIAN_POINT('',(-0.126315008613134,8.61315354740502E-5,3.40565803263806));
#31441=CARTESIAN_POINT('',(-0.12645,1.54856587752183E-17,3.1));
#31442=CARTESIAN_POINT('Ctrl Pts',(-0.126315008613134,8.61315354740502E-5,
3.40565803263806));
#31443=CARTESIAN_POINT('Ctrl Pts',(-0.12640952887744,0.0149751122618111,
3.40472331269183));
#31444=CARTESIAN_POINT('Ctrl Pts',(-0.123973978584825,0.029834173019371,
3.4037885927456));
#31445=CARTESIAN_POINT('Ctrl Pts',(-0.118870621145655,0.0437122030848606,
3.40285387279937));
#31446=CARTESIAN_POINT('Ctrl Pts',(-0.104498255487237,0.0827963011707195,
3.40022146129076));
#31447=CARTESIAN_POINT('Ctrl Pts',(-0.0689667030308244,0.114099547595362,
3.39758904978215));
#31448=CARTESIAN_POINT('Ctrl Pts',(-0.0283829362832705,0.123431722821457,
3.39495663827353));
#31449=CARTESIAN_POINT('Ctrl Pts',(0.0122008304642834,0.132763898047552,
3.39232422676492));
#31450=CARTESIAN_POINT('Ctrl Pts',(0.0578368115029788,0.120125002075099,
3.38969181525631));
#31451=CARTESIAN_POINT('Ctrl Pts',(0.0878375490289461,0.0912444313426293,
3.3870594037477));
#31452=CARTESIAN_POINT('Ctrl Pts',(0.117838286554913,0.0623638606101592,
3.38442699223909));
#31453=CARTESIAN_POINT('Ctrl Pts',(0.132203780568153,0.0172416151176717,
3.38179458073047));
#31454=CARTESIAN_POINT('Ctrl Pts',(0.124421942484303,-0.0236677311728431,
3.37916216922186));
#31455=CARTESIAN_POINT('Ctrl Pts',(0.116640104400452,-0.0645770774633583,
3.37652975771325));
#31456=CARTESIAN_POINT('Ctrl Pts',(0.0867109342195124,-0.1012735245519,
3.37389734620464));
#31457=CARTESIAN_POINT('Ctrl Pts',(0.0482017626101867,-0.117122036149449,
3.37126493469603));
#31458=CARTESIAN_POINT('Ctrl Pts',(0.00969259100086189,-0.132970547746997,
3.36863252318742));
#31459=CARTESIAN_POINT('Ctrl Pts',(-0.0373965820368482,-0.127971123853552,
3.3660001116788));
#31460=CARTESIAN_POINT('Ctrl Pts',(-0.0717195455091802,-0.104390076455735,
3.36336770017019));
#31461=CARTESIAN_POINT('Ctrl Pts',(-0.105227305247545,-0.0813691018472357,
3.36079781099281));
#31462=CARTESIAN_POINT('Ctrl Pts',(-0.126568073655319,-0.0406386849075436,
3.35822792181544));
#31463=CARTESIAN_POINT('Ctrl Pts',(-0.126649735277799,1.79833793418055E-5,
3.35565803263806));
#31464=CARTESIAN_POINT('Ctrl Pts',(-0.126482040448775,-0.000110013702131137,
3.36934196736194));
#31465=CARTESIAN_POINT('Ctrl Pts',(-0.126560666733329,-0.00877918363707953,
3.36988804449155));
#31466=CARTESIAN_POINT('Ctrl Pts',(-0.125744482172779,-0.0174336462000347,
3.37043412162116));
#31467=CARTESIAN_POINT('Ctrl Pts',(-0.123978629867097,-0.0258897947229394,
3.37098019875077));
#31468=CARTESIAN_POINT('Ctrl Pts',(-0.115466187796289,-0.0666533819220227,
3.37361261025938));
#31469=CARTESIAN_POINT('Ctrl Pts',(-0.0848853240803387,-0.102808538565874,
3.37624502176799));
#31470=CARTESIAN_POINT('Ctrl Pts',(-0.046098791601206,-0.117965603239704,
3.3788774332766));
#31471=CARTESIAN_POINT('Ctrl Pts',(-0.00731225912207339,-0.133122667913533,
3.38150984478522));
#31472=CARTESIAN_POINT('Ctrl Pts',(0.0396799421202415,-0.127281640617341,
3.38414225629383));
#31473=CARTESIAN_POINT('Ctrl Pts',(0.0735755598654084,-0.103090344478252,
3.38677466780244));
#31474=CARTESIAN_POINT('Ctrl Pts',(0.107471177610575,-0.0788990483391635,
3.38940707931105));
#31475=CARTESIAN_POINT('Ctrl Pts',(0.128270211858594,-0.0363574833571786,
3.39203949081966));
#31476=CARTESIAN_POINT('Ctrl Pts',(0.126544156121574,0.00524963674486975,
3.39467190232827));
#31477=CARTESIAN_POINT('Ctrl Pts',(0.124818100384554,0.0468567568469189,
3.39730431383689));
#31478=CARTESIAN_POINT('Ctrl Pts',(0.100566954662495,0.0875294320690312,
3.3999367253455));
#31479=CARTESIAN_POINT('Ctrl Pts',(0.0647841180740634,0.108830143717421,
3.40256913685411));
#31480=CARTESIAN_POINT('Ctrl Pts',(0.0290012814856321,0.13013085536581,
3.40520154836272));
#31481=CARTESIAN_POINT('Ctrl Pts',(-0.0183132459691715,0.132059603440478,
3.40783395987133));
#31482=CARTESIAN_POINT('Ctrl Pts',(-0.0557110968410662,0.113742058272906,
3.41046637137995));
#31483=CARTESIAN_POINT('Ctrl Pts',(-0.0931089477129611,0.0954245131053351,
3.41309878288856));
#31484=CARTESIAN_POINT('Ctrl Pts',(-0.120590122001947,0.056860674695525,
3.41573119439717));
#31485=CARTESIAN_POINT('Ctrl Pts',(-0.125697001391323,0.0155320950411155,
3.41836360590578));
#31486=CARTESIAN_POINT('Ctrl Pts',(-0.126329675264624,0.0104120382364903,
3.41868972639117));
#31487=CARTESIAN_POINT('Ctrl Pts',(-0.126618950983805,0.00524954849512788,
3.41901584687656));
#31488=CARTESIAN_POINT('Ctrl Pts',(-0.126579711874066,8.26312290282544E-5,
3.41934196736194));
#31489=CARTESIAN_POINT('Origin',(0.,0.,3.1));
#31490=CARTESIAN_POINT('',(-0.126254420230949,2.98387352259399E-5,3.46934196736194));
#31491=CARTESIAN_POINT('',(-0.126355565467006,-0.000101493988421879,3.45565803263806));
#31492=CARTESIAN_POINT('',(-0.12645,1.54856587752183E-17,3.1));
#31493=CARTESIAN_POINT('Ctrl Pts',(-0.126355565467006,-0.000101493988421879,
3.45565803263806));
#31494=CARTESIAN_POINT('Ctrl Pts',(-0.126135472102513,0.0286572548844595,
3.45385111507683));
#31495=CARTESIAN_POINT('Ctrl Pts',(-0.116386929963108,0.0575510084273647,
3.45204419751561));
#31496=CARTESIAN_POINT('Ctrl Pts',(-0.0983869251245805,0.079755841232973,
3.45023727995438));
#31497=CARTESIAN_POINT('Ctrl Pts',(-0.0721635816202546,0.112104996877157,
3.44760486844577));
#31498=CARTESIAN_POINT('Ctrl Pts',(-0.0284271866124946,0.130257467927816,
3.44497245693716));
#31499=CARTESIAN_POINT('Ctrl Pts',(0.0129959124187107,0.125984473413918,
3.44234004542855));
#31500=CARTESIAN_POINT('Ctrl Pts',(0.0544190114499162,0.121711478900021,
3.43970763391994));
#31501=CARTESIAN_POINT('Ctrl Pts',(0.0935288145045671,0.0950130188215667,
3.43707522241132));
#31502=CARTESIAN_POINT('Ctrl Pts',(0.112596275634196,0.0579918958508686,
3.43444281090271));
#31503=CARTESIAN_POINT('Ctrl Pts',(0.131663736763825,0.0209707728801704,
3.4318103993941));
#31504=CARTESIAN_POINT('Ctrl Pts',(0.130688855968432,-0.0263730129827715,
3.42917798788549));
#31505=CARTESIAN_POINT('Ctrl Pts',(0.110113561023984,-0.0625778311060434,
3.42654557637688));
#31506=CARTESIAN_POINT('Ctrl Pts',(0.0895382660795356,-0.0987826492293151,
3.42391316486827));
#31507=CARTESIAN_POINT('Ctrl Pts',(0.0493625569860325,-0.123848499612917,
3.42128075335965));
#31508=CARTESIAN_POINT('Ctrl Pts',(0.00779867036970612,-0.12641266555449,
3.41864834185104));
#31509=CARTESIAN_POINT('Ctrl Pts',(-0.0337652162466206,-0.128976831496062,
3.41601593034243));
#31510=CARTESIAN_POINT('Ctrl Pts',(-0.0767172803857706,-0.109039312995606,
3.41338351883382));
#31511=CARTESIAN_POINT('Ctrl Pts',(-0.101586723025134,-0.0756380788718395,
3.41075110732521));
#31512=CARTESIAN_POINT('Ctrl Pts',(-0.117625493100354,-0.0540969964234629,
3.40905341576282));
#31513=CARTESIAN_POINT('Ctrl Pts',(-0.126143335529839,-0.0269560826095475,
3.40735572420044));
#31514=CARTESIAN_POINT('Ctrl Pts',(-0.126315008613134,8.61315354740502E-5,
3.40565803263806));
#31515=CARTESIAN_POINT('Ctrl Pts',(-0.126579711874066,8.26312290282544E-5,
3.41934196736194));
#31516=CARTESIAN_POINT('Ctrl Pts',(-0.126302216866535,-0.0364572840554096,
3.42164825838517));
#31517=CARTESIAN_POINT('Ctrl Pts',(-0.109595120153288,-0.0732186276029635,
3.42395454940839));
#31518=CARTESIAN_POINT('Ctrl Pts',(-0.0817223269051259,-0.0967597200814019,
3.42626084043162));
#31519=CARTESIAN_POINT('Ctrl Pts',(-0.0499081885397876,-0.123629634650501,
3.42889325194023));
#31520=CARTESIAN_POINT('Ctrl Pts',(-0.00354732731934525,-0.133276142889689,
3.43152566344884));
#31521=CARTESIAN_POINT('Ctrl Pts',(0.0363442001504806,-0.121326341846207,
3.43415807495745));
#31522=CARTESIAN_POINT('Ctrl Pts',(0.0762357276203061,-0.109376540802726,
3.43679048646606));
#31523=CARTESIAN_POINT('Ctrl Pts',(0.109657921339515,-0.0758304304765741,
3.43942289797468));
#31524=CARTESIAN_POINT('Ctrl Pts',(0.121460011995994,-0.0358949527457304,
3.44205530948329));
#31525=CARTESIAN_POINT('Ctrl Pts',(0.133262102652474,0.00404052498511346,
3.4446877209919));
#31526=CARTESIAN_POINT('Ctrl Pts',(0.123444090246223,0.0503653701206494,
3.44732013250051));
#31527=CARTESIAN_POINT('Ctrl Pts',(0.0964566233770265,0.0820798513966518,
3.44995254400912));
#31528=CARTESIAN_POINT('Ctrl Pts',(0.0694691565078302,0.113794332672654,
3.45258495551774));
#31529=CARTESIAN_POINT('Ctrl Pts',(0.0253122351756883,0.130898450089123,
3.45521736702635));
#31530=CARTESIAN_POINT('Ctrl Pts',(-0.0159971621245858,0.12563865949158,
3.45784977853496));
#31531=CARTESIAN_POINT('Ctrl Pts',(-0.0573065594248602,0.120378868894038,
3.46048219004357));
#31532=CARTESIAN_POINT('Ctrl Pts',(-0.0957684326932668,0.0927551702824843,
3.46311460155218));
#31533=CARTESIAN_POINT('Ctrl Pts',(-0.113947452310361,0.0552897855612304,
3.46574701306079));
#31534=CARTESIAN_POINT('Ctrl Pts',(-0.122222848532838,0.0382349107810562,
3.46694533116118));
#31535=CARTESIAN_POINT('Ctrl Pts',(-0.126295183358791,0.0191406182899676,
3.46814364926156));
#31536=CARTESIAN_POINT('Ctrl Pts',(-0.126254420230949,2.98387352259399E-5,
3.46934196736194));
#31537=CARTESIAN_POINT('Origin',(0.,0.,3.1));
#31538=CARTESIAN_POINT('',(-0.126474550616365,-0.00011099430647141,3.51934196736194));
#31539=CARTESIAN_POINT('',(-0.12665116202208,1.34725138570783E-5,3.50565803263806));
#31540=CARTESIAN_POINT('',(-0.12645,1.54856587752183E-17,3.1));
#31541=CARTESIAN_POINT('Ctrl Pts',(-0.12665116202208,1.34725138570783E-5,
3.50565803263806));
#31542=CARTESIAN_POINT('Ctrl Pts',(-0.126652289762307,0.000752320916696393,
3.50561132897045));
#31543=CARTESIAN_POINT('Ctrl Pts',(-0.126646377467723,0.00149115078533116,
3.50556462530284));
#31544=CARTESIAN_POINT('Ctrl Pts',(-0.126633369929918,0.00222985570861129,
3.50551792163523));
#31545=CARTESIAN_POINT('Ctrl Pts',(-0.125900211401467,0.0438663147077999,
3.50288551012662));
#31546=CARTESIAN_POINT('Ctrl Pts',(-0.102626068622182,0.0851058329421116,
3.50025309861801));
#31547=CARTESIAN_POINT('Ctrl Pts',(-0.067361469104998,0.107253962401741,
3.4976206871094));
#31548=CARTESIAN_POINT('Ctrl Pts',(-0.0320968695878142,0.129402091861371,
3.49498827560079));
#31549=CARTESIAN_POINT('Ctrl Pts',(0.0151581866672683,0.132458832546319,
3.49235586409217));
#31550=CARTESIAN_POINT('Ctrl Pts',(0.0529823007948782,0.115038504173862,
3.48972345258356));
#31551=CARTESIAN_POINT('Ctrl Pts',(0.0908064149224882,0.0976181758014056,
3.48709104107495));
#31552=CARTESIAN_POINT('Ctrl Pts',(0.119199586922625,0.0597207783715444,
3.48445862956634));
#31553=CARTESIAN_POINT('Ctrl Pts',(0.125290771676778,0.0185257643337426,
3.48182621805773));
#31554=CARTESIAN_POINT('Ctrl Pts',(0.131381956430931,-0.0226692497040593,
3.47919380654911));
#31555=CARTESIAN_POINT('Ctrl Pts',(0.115171153939098,-0.0671618803498017,
3.4765613950405));
#31556=CARTESIAN_POINT('Ctrl Pts',(0.0840069606582608,-0.0947829713159226,
3.47392898353189));
#31557=CARTESIAN_POINT('Ctrl Pts',(0.0528427673774234,-0.122404062282043,
3.47129657202328));
#31558=CARTESIAN_POINT('Ctrl Pts',(0.00672518330758078,-0.133153613568543,
3.46866416051467));
#31559=CARTESIAN_POINT('Ctrl Pts',(-0.0334400173720784,-0.122158694217057,
3.46603174900606));
#31560=CARTESIAN_POINT('Ctrl Pts',(-0.0736052180517379,-0.111163774865571,
3.46339933749744));
#31561=CARTESIAN_POINT('Ctrl Pts',(-0.107818035341214,-0.0784243848761005,
3.46076692598883));
#31562=CARTESIAN_POINT('Ctrl Pts',(-0.120569297985506,-0.0387817697625104,
3.45813451448022));
#31563=CARTESIAN_POINT('Ctrl Pts',(-0.12456794717085,-0.0263503019894106,
3.45730902053283));
#31564=CARTESIAN_POINT('Ctrl Pts',(-0.126456115566329,-0.013239986655944,
3.45648352658544));
#31565=CARTESIAN_POINT('Ctrl Pts',(-0.126355565467006,-0.000101493988421879,
3.45565803263806));
#31566=CARTESIAN_POINT('Ctrl Pts',(-0.126254420230949,2.98387352259399E-5,
3.46934196736194));
#31567=CARTESIAN_POINT('Ctrl Pts',(-0.126205636746063,-0.0228410859189539,
3.47077606077017));
#31568=CARTESIAN_POINT('Ctrl Pts',(-0.120265979813939,-0.045735623724726,
3.4722101541784));
#31569=CARTESIAN_POINT('Ctrl Pts',(-0.108589648601543,-0.0651864304899691,
3.47364424758663));
#31570=CARTESIAN_POINT('Ctrl Pts',(-0.0871566593098471,-0.100890190988961,
3.47627665909524));
#31571=CARTESIAN_POINT('Ctrl Pts',(-0.0463945147606729,-0.124990641155991,
3.47890907060385));
#31572=CARTESIAN_POINT('Ctrl Pts',(-0.00478129205129982,-0.126562712056682,
3.48154148211247));
#31573=CARTESIAN_POINT('Ctrl Pts',(0.0368319306580732,-0.128134782957373,
3.48417389362108));
#31574=CARTESIAN_POINT('Ctrl Pts',(0.0792962315276452,-0.107178474591724,
3.48680630512969));
#31575=CARTESIAN_POINT('Ctrl Pts',(0.103361923070995,-0.0731935540746058,
3.4894387166383));
#31576=CARTESIAN_POINT('Ctrl Pts',(0.127427614614345,-0.0392086335574879,
3.49207112814691));
#31577=CARTESIAN_POINT('Ctrl Pts',(0.133094696831473,0.00780489911109889,
3.49470353965553));
#31578=CARTESIAN_POINT('Ctrl Pts',(0.117794195954941,0.0465350563376696,
3.49733595116414));
#31579=CARTESIAN_POINT('Ctrl Pts',(0.102493695078409,0.0852652135642405,
3.49996836267275));
#31580=CARTESIAN_POINT('Ctrl Pts',(0.0662256111082176,0.115711995348795,
3.50260077418136));
#31581=CARTESIAN_POINT('Ctrl Pts',(0.0254308018677658,0.124073556121702,
3.50523318568997));
#31582=CARTESIAN_POINT('Ctrl Pts',(-0.0153640073726858,0.13243511689461,
3.50786559719859));
#31583=CARTESIAN_POINT('Ctrl Pts',(-0.0606855418833975,0.118711456655871,
3.5104980087072));
#31584=CARTESIAN_POINT('Ctrl Pts',(-0.0899888963160071,0.0891234688732135,
3.51313042021581));
#31585=CARTESIAN_POINT('Ctrl Pts',(-0.113037365625426,0.0658511220193964,
3.51520093593118));
#31586=CARTESIAN_POINT('Ctrl Pts',(-0.12617608552629,0.032764207609907,
3.51727145164656));
#31587=CARTESIAN_POINT('Ctrl Pts',(-0.126474550616365,-0.00011099430647141,
3.51934196736194));
#31588=CARTESIAN_POINT('Origin',(0.,0.,3.1));
#31589=CARTESIAN_POINT('',(-0.126585968300139,7.56654190205152E-5,3.56934196736194));
#31590=CARTESIAN_POINT('',(-0.126320239448181,8.84447983197572E-5,3.55565803263806));
#31591=CARTESIAN_POINT('',(-0.12645,1.54856587752183E-17,3.1));
#31592=CARTESIAN_POINT('',(0.0958116152722374,0.0825211298936506,3.6));
#31593=CARTESIAN_POINT('Ctrl Pts',(-0.126585968300139,7.56654190205153E-5,
3.56934196736194));
#31594=CARTESIAN_POINT('Ctrl Pts',(-0.126314022279117,-0.0367013527487602,
3.57166407704879));
#31595=CARTESIAN_POINT('Ctrl Pts',(-0.109347743467702,-0.0736867832767084,
3.57398618673564));
#31596=CARTESIAN_POINT('Ctrl Pts',(-0.0811433985852254,-0.0972323262171825,
3.57630829642249));
#31597=CARTESIAN_POINT('Ctrl Pts',(-0.0491701276919849,-0.123924242866945,
3.57894070793111));
#31598=CARTESIAN_POINT('Ctrl Pts',(-0.00275464590947525,-0.133344354062013,
3.58157311943972));
#31599=CARTESIAN_POINT('Ctrl Pts',(0.0370665801591162,-0.121131220741312,
3.58420553094833));
#31600=CARTESIAN_POINT('Ctrl Pts',(0.0768878062277077,-0.108918087420612,
3.58683794245694));
#31601=CARTESIAN_POINT('Ctrl Pts',(0.110114776582381,-0.0750717095841421,
3.58947035396555));
#31602=CARTESIAN_POINT('Ctrl Pts',(0.121670197120012,-0.035135491975585,
3.59210276547417));
#31603=CARTESIAN_POINT('Ctrl Pts',(0.133225617657642,0.004800725632972,
3.59473517698278));
#31604=CARTESIAN_POINT('Ctrl Pts',(0.12310948837823,0.0508267830136165,
3.59736758849139));
#31605=CARTESIAN_POINT('Ctrl Pts',(0.0958116152722374,0.0825211298936506,
3.6));
#31606=CARTESIAN_POINT('',(-0.0959914412498779,0.0826500850312143,3.6));
#31607=CARTESIAN_POINT('Origin',(0.,0.,3.6));
#31608=CARTESIAN_POINT('Ctrl Pts',(-0.0959917963302685,0.0826503396631676,
3.6));
#31609=CARTESIAN_POINT('Ctrl Pts',(-0.0697118464080321,0.11301028941478,
3.59746250047314));
#31610=CARTESIAN_POINT('Ctrl Pts',(-0.0277082920252644,0.129939468632456,
3.59492500094628));
#31611=CARTESIAN_POINT('Ctrl Pts',(0.0122513409849536,0.126048715034846,
3.59238750141942));
#31612=CARTESIAN_POINT('Ctrl Pts',(0.0537056138636675,0.122012432687161,
3.58975508991081));
#31613=CARTESIAN_POINT('Ctrl Pts',(0.0929602052199782,0.095569602745952,
3.5871226784022));
#31614=CARTESIAN_POINT('Ctrl Pts',(0.112244799198078,0.058668125616663,
3.58449026689359));
#31615=CARTESIAN_POINT('Ctrl Pts',(0.131529393176178,0.0217666484873742,
3.58185785538498));
#31616=CARTESIAN_POINT('Ctrl Pts',(0.130843989776067,-0.0255934758299944,
3.57922544387636));
#31617=CARTESIAN_POINT('Ctrl Pts',(0.11048667870984,-0.0619230812123589,
3.57659303236775));
#31618=CARTESIAN_POINT('Ctrl Pts',(0.0901293676436137,-0.0982526865947235,
3.57396062085914));
#31619=CARTESIAN_POINT('Ctrl Pts',(0.0501001489112715,-0.123551773042084,
3.57132820935053));
#31620=CARTESIAN_POINT('Ctrl Pts',(0.00855140333287623,-0.126362339932449,
3.56869579784192));
#31621=CARTESIAN_POINT('Ctrl Pts',(-0.032997342245519,-0.129172906822815,
3.5660633863333));
#31622=CARTESIAN_POINT('Ctrl Pts',(-0.0760656146699672,-0.109494954156186,
3.56343097482469));
#31623=CARTESIAN_POINT('Ctrl Pts',(-0.101133339862815,-0.0762433587436205,
3.56079856331608));
#31624=CARTESIAN_POINT('Ctrl Pts',(-0.117450622825668,-0.0545989659182217,
3.55908505309007));
#31625=CARTESIAN_POINT('Ctrl Pts',(-0.126140944400475,-0.0272033229899018,
3.55737154286407));
#31626=CARTESIAN_POINT('Ctrl Pts',(-0.126320239448181,8.84447983197572E-5,
3.55565803263806));
#31627=CARTESIAN_POINT('Origin',(0.,0.,3.71042117235887));
#31628=CARTESIAN_POINT('',(-0.154532329218545,4.4775541170855E-5,2.73957882764113));
#31629=CARTESIAN_POINT('',(-0.154050519949587,1.7733618556367E-5,2.73542117235887));
#31630=CARTESIAN_POINT('',(-0.1543,1.43283619370552E-14,3.71042117235887));
#31631=CARTESIAN_POINT('',(0.03985138418574,-0.149064942821847,2.7));
#31632=CARTESIAN_POINT('Ctrl Pts',(-0.154050519949587,1.77336185563769E-5,
2.73542117235887));
#31633=CARTESIAN_POINT('Ctrl Pts',(-0.154066274679179,0.0248826176783822,
2.73414376094036));
#31634=CARTESIAN_POINT('Ctrl Pts',(-0.136678442565,0.100960491967761,2.73023393801324));
#31635=CARTESIAN_POINT('Ctrl Pts',(-0.0176337922607613,0.181151847216363,
2.72369170357751));
#31636=CARTESIAN_POINT('Ctrl Pts',(0.14217180017934,0.113903091069576,2.71579446905167));
#31637=CARTESIAN_POINT('Ctrl Pts',(0.172848115381474,-0.0569943527276058,
2.70789723452584));
#31638=CARTESIAN_POINT('Ctrl Pts',(0.0891618565332066,-0.135882161272415,
2.70263241150861));
#31639=CARTESIAN_POINT('Ctrl Pts',(0.0398513841857358,-0.149064942821848,
2.7));
#31640=CARTESIAN_POINT('',(-0.0398513841857137,-0.149064942821854,2.7));
#31641=CARTESIAN_POINT('Origin',(0.,0.,2.7));
#31642=CARTESIAN_POINT('Ctrl Pts',(-0.154532329218545,4.47755411708581E-5,
2.73957882764113));
#31643=CARTESIAN_POINT('Ctrl Pts',(-0.154541474731814,0.00247370285197769,
2.73945303065539));
#31644=CARTESIAN_POINT('Ctrl Pts',(-0.153393280968798,0.0557210645369631,
2.73669482216104));
#31645=CARTESIAN_POINT('Ctrl Pts',(-0.0921890914137533,0.156981837366664,
2.73130420215808));
#31646=CARTESIAN_POINT('Ctrl Pts',(0.081054919689294,0.163034936656946,
2.72340696763225));
#31647=CARTESIAN_POINT('Ctrl Pts',(0.180814453969382,0.0212164304176998,
2.71550973310641));
#31648=CARTESIAN_POINT('Ctrl Pts',(0.117409156055766,-0.137788854076994,
2.70770741056233));
#31649=CARTESIAN_POINT('Ctrl Pts',(0.00742265010309158,-0.161856516962739,
2.70253749952686));
#31650=CARTESIAN_POINT('Ctrl Pts',(-0.0399441884684105,-0.149319082708151,
2.7));
#31651=CARTESIAN_POINT('Origin',(0.,0.,3.71042117235887));
#31652=CARTESIAN_POINT('',(-0.154111134012939,9.12056675990702E-5,2.78957882764113));
#31653=CARTESIAN_POINT('',(-0.154375356381381,-0.000128347871137961,2.78542117235887));
#31654=CARTESIAN_POINT('',(-0.1543,1.43283619370552E-14,3.71042117235887));
#31655=CARTESIAN_POINT('Ctrl Pts',(-0.154375356381381,-0.000128347871137957,
2.78542117235887));
#31656=CARTESIAN_POINT('Ctrl Pts',(-0.154004490723256,0.0414883916240874,
2.78327156332537));
#31657=CARTESIAN_POINT('Ctrl Pts',(-0.115247407249284,0.134678118697344,
2.77848954278325));
#31658=CARTESIAN_POINT('Ctrl Pts',(0.0418557848916964,0.17717956471448,
2.77107511073252));
#31659=CARTESIAN_POINT('Ctrl Pts',(0.171243621830244,0.0618160489303277,
2.76317787620668));
#31660=CARTESIAN_POINT('Ctrl Pts',(0.145372553280857,-0.109598760687136,
2.75528064168085));
#31661=CARTESIAN_POINT('Ctrl Pts',(-0.0122890050489303,-0.181634550845065,
2.74738340715501));
#31662=CARTESIAN_POINT('Ctrl Pts',(-0.13512250192602,-0.104001863717814,
2.74076358404769));
#31663=CARTESIAN_POINT('Ctrl Pts',(-0.154033808293727,-0.0263574182340484,
2.73677617244897));
#31664=CARTESIAN_POINT('Ctrl Pts',(-0.154050519949587,1.77336185563769E-5,
2.73542117235887));
#31665=CARTESIAN_POINT('Ctrl Pts',(-0.154111134012939,9.12056675990824E-5,
2.78957882764113));
#31666=CARTESIAN_POINT('Ctrl Pts',(-0.154216904845773,0.0194969338944761,
2.7885808330404));
#31667=CARTESIAN_POINT('Ctrl Pts',(-0.141845660080373,0.0899592653630177,
2.78495042693105));
#31668=CARTESIAN_POINT('Ctrl Pts',(-0.0365555263461618,0.178349534836247,
2.7786876093131));
#31669=CARTESIAN_POINT('Ctrl Pts',(0.129354617910885,0.128110846926664,
2.77079037478726));
#31670=CARTESIAN_POINT('Ctrl Pts',(0.177988125847537,-0.0382780523762908,
2.76289314026143));
#31671=CARTESIAN_POINT('Ctrl Pts',(0.0652523050728403,-0.169960699505811,
2.75499590573559));
#31672=CARTESIAN_POINT('Ctrl Pts',(-0.10390483603623,-0.147913217635949,
2.74722446819549));
#31673=CARTESIAN_POINT('Ctrl Pts',(-0.154350096899974,-0.0483537169716228,
2.742085442164));
#31674=CARTESIAN_POINT('Ctrl Pts',(-0.154532329218545,4.47755411708581E-5,
2.73957882764113));
#31675=CARTESIAN_POINT('Origin',(0.,0.,3.71042117235887));
#31676=CARTESIAN_POINT('',(-0.154217143654561,-0.000131209131675823,2.83957882764113));
#31677=CARTESIAN_POINT('',(-0.154426485097132,0.00011404955978979,2.83542117235887));
#31678=CARTESIAN_POINT('',(-0.1543,1.43283619370552E-14,3.71042117235887));
#31679=CARTESIAN_POINT('Ctrl Pts',(-0.154426485097132,0.000114049559789811,
2.83542117235887));
#31680=CARTESIAN_POINT('Ctrl Pts',(-0.154488936846892,0.00764629898056818,
2.83503177721898));
#31681=CARTESIAN_POINT('Ctrl Pts',(-0.15057776842572,0.0660334076153961,
2.83200997057048));
#31682=CARTESIAN_POINT('Ctrl Pts',(-0.0761594594163292,0.165362226259928,
2.82635575241337));
#31683=CARTESIAN_POINT('Ctrl Pts',(0.0968288057644592,0.154172306963803,
2.81845851788754));
#31684=CARTESIAN_POINT('Ctrl Pts',(0.182029287997112,0.0032053357021354,
2.8105612833617));
#31685=CARTESIAN_POINT('Ctrl Pts',(0.102196604793212,-0.150667825661861,
2.80266404883587));
#31686=CARTESIAN_POINT('Ctrl Pts',(-0.0702903425019912,-0.167940860695529,
2.79476681431002));
#31687=CARTESIAN_POINT('Ctrl Pts',(-0.14944611336054,-0.069697339741445,
2.7890191888177));
#31688=CARTESIAN_POINT('Ctrl Pts',(-0.154458652857569,-0.00947547310228015,
2.78590397483398));
#31689=CARTESIAN_POINT('Ctrl Pts',(-0.154375356381381,-0.000128347871137957,
2.78542117235887));
#31690=CARTESIAN_POINT('Ctrl Pts',(-0.154217143654561,-0.000131209131675806,
2.83957882764113));
#31691=CARTESIAN_POINT('Ctrl Pts',(-0.153918019192818,0.0361710755121499,
2.8377086354254));
#31692=CARTESIAN_POINT('Ctrl Pts',(-0.123049963751881,0.124029060195803,
2.83320603170106));
#31693=CARTESIAN_POINT('Ctrl Pts',(0.0229951363840201,0.180599411232496,
2.82607101646811));
#31694=CARTESIAN_POINT('Ctrl Pts',(0.163793876249876,0.0794763606914083,
2.81817378194228));
#31695=CARTESIAN_POINT('Ctrl Pts',(0.1560922965942,-0.0937023067775016,
2.81027654741644));
#31696=CARTESIAN_POINT('Ctrl Pts',(0.00687287227597422,-0.181927677084725,
2.8023793128906));
#31697=CARTESIAN_POINT('Ctrl Pts',(-0.128932992743455,-0.114906920263654,
2.7954800729655));
#31698=CARTESIAN_POINT('Ctrl Pts',(-0.153937912998098,-0.0316895778160955,
2.79121324454901));
#31699=CARTESIAN_POINT('Ctrl Pts',(-0.154111134012939,9.12056675990824E-5,
2.78957882764113));
#31700=CARTESIAN_POINT('Origin',(0.,0.,3.71042117235887));
#31701=CARTESIAN_POINT('',(-0.154535784933253,3.81877733398595E-5,2.88957882764113));
#31702=CARTESIAN_POINT('',(-0.154054921884602,1.70237768407695E-5,2.88542117235887));
#31703=CARTESIAN_POINT('',(-0.1543,1.43283619370552E-14,3.71042117235887));
#31704=CARTESIAN_POINT('Ctrl Pts',(-0.154054921884602,1.70237768407841E-5,
2.88542117235887));
#31705=CARTESIAN_POINT('Ctrl Pts',(-0.154079346410273,0.0245707720672152,
2.88415957960399));
#31706=CARTESIAN_POINT('Ctrl Pts',(-0.1369997697474,0.100325734672348,2.88026557534049));
#31707=CARTESIAN_POINT('Ctrl Pts',(-0.0186809878927599,0.181096514045709,
2.87373915956839));
#31708=CARTESIAN_POINT('Ctrl Pts',(0.14142638889208,0.114645117640021,2.86584192504255));
#31709=CARTESIAN_POINT('Ctrl Pts',(0.173312464619039,-0.0557468952238434,
2.85794469051671));
#31710=CARTESIAN_POINT('Ctrl Pts',(0.0480683875166603,-0.175597144601074,
2.85004745599088));
#31711=CARTESIAN_POINT('Ctrl Pts',(-0.112431541495112,-0.138186203572753,
2.84253961660493));
#31712=CARTESIAN_POINT('Ctrl Pts',(-0.154066746922155,-0.0432736484708866,
2.8376641887276));
#31713=CARTESIAN_POINT('Ctrl Pts',(-0.154426485097132,0.000114049559789811,
2.83542117235887));
#31714=CARTESIAN_POINT('Ctrl Pts',(-0.154535784933253,3.8187773339879E-5,
2.88957882764113));
#31715=CARTESIAN_POINT('Ctrl Pts',(-0.154542902681706,0.00216158596911697,
2.88946884931902));
#31716=CARTESIAN_POINT('Ctrl Pts',(-0.153545003294962,0.0551032333888324,
2.8867264594883));
#31717=CARTESIAN_POINT('Ctrl Pts',(-0.0931239936920636,0.15643799622185,
2.88135165814895));
#31718=CARTESIAN_POINT('Ctrl Pts',(0.080081970475175,0.163498632518342,
2.87345442362313));
#31719=CARTESIAN_POINT('Ctrl Pts',(0.180683277203119,0.0223266252501708,
2.86555718909729));
#31720=CARTESIAN_POINT('Ctrl Pts',(0.11747183849698,-0.139087354145018,
2.85765995457145));
#31721=CARTESIAN_POINT('Ctrl Pts',(-0.0522430059551858,-0.174400668051551,
2.84976272004562));
#31722=CARTESIAN_POINT('Ctrl Pts',(-0.145618409602951,-0.0806790644135928,
2.84373567773551));
#31723=CARTESIAN_POINT('Ctrl Pts',(-0.154339055420526,-0.0149266411191706,
2.84034104693401));
#31724=CARTESIAN_POINT('Ctrl Pts',(-0.154217143654561,-0.000131209131675806,
2.83957882764113));
#31725=CARTESIAN_POINT('Origin',(0.,0.,3.71042117235887));
#31726=CARTESIAN_POINT('',(-0.154116825055928,9.48496454908493E-5,2.93957882764113));
#31727=CARTESIAN_POINT('',(-0.154366358871002,-0.000130096805920683,2.93542117235887));
#31728=CARTESIAN_POINT('',(-0.1543,1.43283619370552E-14,3.71042117235887));
#31729=CARTESIAN_POINT('Ctrl Pts',(-0.154366358871002,-0.000130096805920679,
2.93542117235887));
#31730=CARTESIAN_POINT('Ctrl Pts',(-0.153995797272422,0.0411865074797718,
2.93328738198899));
#31731=CARTESIAN_POINT('Ctrl Pts',(-0.115714146224304,0.134080683615333,
2.9285211801105));
#31732=CARTESIAN_POINT('Ctrl Pts',(0.0407990816336726,0.177427059877793,
2.9211225667234));
#31733=CARTESIAN_POINT('Ctrl Pts',(0.170870699467283,0.0628341523235889,
2.91322533219756));
#31734=CARTESIAN_POINT('Ctrl Pts',(0.146025941933673,-0.108726036068736,
2.90532809767173));
#31735=CARTESIAN_POINT('Ctrl Pts',(-0.0112102069433731,-0.181712019164164,
2.89743086314589));
#31736=CARTESIAN_POINT('Ctrl Pts',(-0.134787821110527,-0.104611252124613,
2.89079522137494));
#31737=CARTESIAN_POINT('Ctrl Pts',(-0.154028382735806,-0.026662535455284,
2.8867919911126));
#31738=CARTESIAN_POINT('Ctrl Pts',(-0.154054921884602,1.70237768407841E-5,
2.88542117235887));
#31739=CARTESIAN_POINT('Ctrl Pts',(-0.154116825055928,9.48496454908822E-5,
2.93957882764113));
#31740=CARTESIAN_POINT('Ctrl Pts',(-0.154225358468008,0.0191912107511692,
2.93859665170402));
#31741=CARTESIAN_POINT('Ctrl Pts',(-0.1421149984489,0.0893365787084054,
2.93498206425831));
#31742=CARTESIAN_POINT('Ctrl Pts',(-0.0376184643267171,0.178128537842515,
2.92873506530397));
#31743=CARTESIAN_POINT('Ctrl Pts',(0.128588348481182,0.128879639534425,
2.92083783077814));
#31744=CARTESIAN_POINT('Ctrl Pts',(0.178213202383553,-0.0372153106656781,
2.9129405962523));
#31745=CARTESIAN_POINT('Ctrl Pts',(0.0662647529343645,-0.169569771398652,
2.90504336172647));
#31746=CARTESIAN_POINT('Ctrl Pts',(-0.10336559476711,-0.148485092132862,
2.89725610552274));
#31747=CARTESIAN_POINT('Ctrl Pts',(-0.154372534171041,-0.0486635015632469,
2.89210126082763));
#31748=CARTESIAN_POINT('Ctrl Pts',(-0.154535784933253,3.8187773339879E-5,
2.88957882764113));
#31749=CARTESIAN_POINT('Origin',(0.,0.,3.71042117235887));
#31750=CARTESIAN_POINT('',(-0.154208836002914,-0.000129626704909153,2.98957882764113));
#31751=CARTESIAN_POINT('',(-0.154434696759477,0.000111004303427491,2.98542117235887));
#31752=CARTESIAN_POINT('',(-0.1543,1.43283619370552E-14,3.71042117235887));
#31753=CARTESIAN_POINT('Ctrl Pts',(-0.154434696759477,0.000111004303427509,
2.98542117235887));
#31754=CARTESIAN_POINT('Ctrl Pts',(-0.15449350107168,0.00733626390374423,
2.98504759588261));
#31755=CARTESIAN_POINT('Ctrl Pts',(-0.150762340620084,0.0654133961639385,
2.98204160789773));
#31756=CARTESIAN_POINT('Ctrl Pts',(-0.0771442428547834,0.164905101290741,
2.97640320840425));
#31757=CARTESIAN_POINT('Ctrl Pts',(0.0959076962473017,0.15474702077238,
2.96850597387841));
#31758=CARTESIAN_POINT('Ctrl Pts',(0.182006911912947,0.00429076371209153,
2.96060873935257));
#31759=CARTESIAN_POINT('Ctrl Pts',(0.103093336173269,-0.150055625266004,
2.95271150482674));
#31760=CARTESIAN_POINT('Ctrl Pts',(-0.069287674394006,-0.168357194128057,
2.9448142703009));
#31761=CARTESIAN_POINT('Ctrl Pts',(-0.14924717784082,-0.0703180680940833,
2.93905082614495));
#31762=CARTESIAN_POINT('Ctrl Pts',(-0.154452951185252,-0.00978490290509501,
2.9359197934976));
#31763=CARTESIAN_POINT('Ctrl Pts',(-0.154366358871002,-0.000130096805920679,
2.93542117235887));
#31764=CARTESIAN_POINT('Ctrl Pts',(-0.154208836002914,-0.00012962670490916,
2.98957882764113));
#31765=CARTESIAN_POINT('Ctrl Pts',(-0.15391701905173,0.0358705210125992,
2.98772445408903));
#31766=CARTESIAN_POINT('Ctrl Pts',(-0.123464382903156,0.123420397725162,
2.98323766902831));
#31767=CARTESIAN_POINT('Ctrl Pts',(0.0219177299165732,0.180733333857582,
2.97611847245899));
#31768=CARTESIAN_POINT('Ctrl Pts',(0.163317009898163,0.0804517192475515,
2.96822123793315));
#31769=CARTESIAN_POINT('Ctrl Pts',(0.156648310460303,-0.0927697778475837,
2.96032400340732));
#31770=CARTESIAN_POINT('Ctrl Pts',(0.00795766962277319,-0.181883480135435,
2.95242676888148));
#31771=CARTESIAN_POINT('Ctrl Pts',(-0.128557747147415,-0.11552191978543,
2.94551171029275));
#31772=CARTESIAN_POINT('Ctrl Pts',(-0.1539344690334,-0.0319905366812824,
2.94122906321263));
#31773=CARTESIAN_POINT('Ctrl Pts',(-0.154116825055928,9.48496454908822E-5,
2.93957882764113));
#31774=CARTESIAN_POINT('Origin',(0.,0.,3.71042117235887));
#31775=CARTESIAN_POINT('',(-0.154538871978598,3.2832780837988E-5,3.03957882764113));
#31776=CARTESIAN_POINT('',(-0.154056089165245,2.19184202627989E-5,3.03542117235887));
#31777=CARTESIAN_POINT('',(-0.1543,1.43283619370552E-14,3.71042117235887));
#31778=CARTESIAN_POINT('Ctrl Pts',(-0.154056089165245,2.19184202628134E-5,
3.03542117235887));
#31779=CARTESIAN_POINT('Ctrl Pts',(-0.154087155299894,0.0242673368387721,
3.03417539826761));
#31780=CARTESIAN_POINT('Ctrl Pts',(-0.137310014833352,0.0997044362362006,
3.03029721266774));
#31781=CARTESIAN_POINT('Ctrl Pts',(-0.0197606177252597,0.180981890321858,
3.02378661555926));
#31782=CARTESIAN_POINT('Ctrl Pts',(0.140740192743497,0.115486470133437,
3.01588938103343));
#31783=CARTESIAN_POINT('Ctrl Pts',(0.173641826766224,-0.0547123627222005,
3.00799214650759));
#31784=CARTESIAN_POINT('Ctrl Pts',(0.0491147003187017,-0.175307366787479,
3.00009491198175));
#31785=CARTESIAN_POINT('Ctrl Pts',(-0.11194410582055,-0.138777425062269,
2.99257125393218));
#31786=CARTESIAN_POINT('Ctrl Pts',(-0.15407913571938,-0.0435766220328422,
2.98768000739122));
#31787=CARTESIAN_POINT('Ctrl Pts',(-0.154434696759477,0.000111004303427509,
2.98542117235887));
#31788=CARTESIAN_POINT('Ctrl Pts',(-0.154538871978598,3.28327808380407E-5,
3.03957882764113));
#31789=CARTESIAN_POINT('Ctrl Pts',(-0.154544182685759,0.00185071603346938,
3.03948466798264));
#31790=CARTESIAN_POINT('Ctrl Pts',(-0.153694834634547,0.0544858891421056,
3.03675809681555));
#31791=CARTESIAN_POINT('Ctrl Pts',(-0.0940552495850459,0.15587987322763,
3.03139911413983));
#31792=CARTESIAN_POINT('Ctrl Pts',(0.0791055288760802,0.163973290975094,
3.02350187961401));
#31793=CARTESIAN_POINT('Ctrl Pts',(0.180546920428939,0.0234037256776295,
3.01560464508816));
#31794=CARTESIAN_POINT('Ctrl Pts',(0.118299191571216,-0.138384342053441,
3.00770741056233));
#31795=CARTESIAN_POINT('Ctrl Pts',(-0.0512020455023775,-0.174709116500372,
2.99981017603649));
#31796=CARTESIAN_POINT('Ctrl Pts',(-0.145381230907426,-0.0813015016053826,
2.99376731506276));
#31797=CARTESIAN_POINT('Ctrl Pts',(-0.154331273396456,-0.0152341784994835,
2.99035686559764));
#31798=CARTESIAN_POINT('Ctrl Pts',(-0.154208836002914,-0.00012962670490916,
2.98957882764113));
#31799=CARTESIAN_POINT('Origin',(0.,0.,3.71042117235887));
#31800=CARTESIAN_POINT('',(-0.154122750472518,9.83954699399631E-5,3.08957882764113));
#31801=CARTESIAN_POINT('',(-0.154357314101369,-0.000131672715837502,3.08542117235887));
#31802=CARTESIAN_POINT('',(-0.1543,1.43283619370552E-14,3.71042117235887));
#31803=CARTESIAN_POINT('Ctrl Pts',(-0.154357314101369,-0.000131672715837496,
3.08542117235887));
#31804=CARTESIAN_POINT('Ctrl Pts',(-0.153987553769485,0.0408848376338906,
3.08330320065262));
#31805=CARTESIAN_POINT('Ctrl Pts',(-0.11617759776856,0.133482913719063,
3.07855281743775));
#31806=CARTESIAN_POINT('Ctrl Pts',(0.039740276922879,0.17766720864428,3.07117002271427));
#31807=CARTESIAN_POINT('Ctrl Pts',(0.170492952144154,0.0638520156810144,
3.06327278818844));
#31808=CARTESIAN_POINT('Ctrl Pts',(0.146671728755708,-0.107853282848364,
3.0553755536626));
#31809=CARTESIAN_POINT('Ctrl Pts',(-0.0101263751692898,-0.181775639631079,
3.04747831913677));
#31810=CARTESIAN_POINT('Ctrl Pts',(-0.134457266065241,-0.105231153897523,
3.04082685870219));
#31811=CARTESIAN_POINT('Ctrl Pts',(-0.154021510291741,-0.026965000487735,
3.03680780977622));
#31812=CARTESIAN_POINT('Ctrl Pts',(-0.154056089165245,2.19184202628134E-5,
3.03542117235887));
#31813=CARTESIAN_POINT('Ctrl Pts',(-0.154122750472518,9.83954699399839E-5,
3.08957882764113));
#31814=CARTESIAN_POINT('Ctrl Pts',(-0.154233799032612,0.0188853799021587,
3.08861247036765));
#31815=CARTESIAN_POINT('Ctrl Pts',(-0.142381965748736,0.0887139061579003,
3.08501370158555));
#31816=CARTESIAN_POINT('Ctrl Pts',(-0.0386800578824722,0.177901034213339,
3.07878252129485));
#31817=CARTESIAN_POINT('Ctrl Pts',(0.127817493356429,0.129644179368171,
3.07088528676902));
#31818=CARTESIAN_POINT('Ctrl Pts',(0.178431965499368,-0.0361518815554529,
3.06298805224317));
#31819=CARTESIAN_POINT('Ctrl Pts',(0.0672747972491473,-0.169171588947593,
3.05509081771735));
#31820=CARTESIAN_POINT('Ctrl Pts',(-0.102823100152332,-0.149058093692613,
3.04728774284999));
#31821=CARTESIAN_POINT('Ctrl Pts',(-0.154395711813265,-0.0489716517674636,
3.04211707949126));
#31822=CARTESIAN_POINT('Ctrl Pts',(-0.154538871978598,3.28327808380407E-5,
3.03957882764113));
#31823=CARTESIAN_POINT('Origin',(0.,0.,3.71042117235887));
#31824=CARTESIAN_POINT('',(-0.154200664638475,-0.000127870236170058,3.13957882764113));
#31825=CARTESIAN_POINT('',(-0.154442743231392,0.000107782702043065,3.13542117235887));
#31826=CARTESIAN_POINT('',(-0.1543,1.43283619370552E-14,3.71042117235887));
#31827=CARTESIAN_POINT('Ctrl Pts',(-0.154442743231391,0.000107782702043087,
3.13542117235887));
#31828=CARTESIAN_POINT('Ctrl Pts',(-0.154497895338046,0.00702615569019676,
3.13506341454624));
#31829=CARTESIAN_POINT('Ctrl Pts',(-0.150944880930953,0.0647935208243374,
3.13207324522499));
#31830=CARTESIAN_POINT('Ctrl Pts',(-0.0781262761399388,0.164442122383114,
3.12645066439512));
#31831=CARTESIAN_POINT('Ctrl Pts',(0.0949831631341886,0.155316210867962,
3.11855342986929));
#31832=CARTESIAN_POINT('Ctrl Pts',(0.181978087741923,0.00537607841744088,
3.11065619534345));
#31833=CARTESIAN_POINT('Ctrl Pts',(0.10398635378076,-0.149438164016893,
3.10275896081762));
#31834=CARTESIAN_POINT('Ctrl Pts',(-0.0682824508977375,-0.168767394767933,
3.09486172629178));
#31835=CARTESIAN_POINT('Ctrl Pts',(-0.14904624696594,-0.0709390773474446,
3.0890824634722));
#31836=CARTESIAN_POINT('Ctrl Pts',(-0.154447126175577,-0.0100942824218163,
3.08593561216123));
#31837=CARTESIAN_POINT('Ctrl Pts',(-0.154357314101369,-0.000131672715837496,
3.08542117235887));
#31838=CARTESIAN_POINT('Ctrl Pts',(-0.154200664638475,-0.000127870236170063,
3.13957882764113));
#31839=CARTESIAN_POINT('Ctrl Pts',(-0.153916387321455,0.03556997377657,
3.13774027275265));
#31840=CARTESIAN_POINT('Ctrl Pts',(-0.123875930184563,0.122811200111113,
3.13326930635556));
#31841=CARTESIAN_POINT('Ctrl Pts',(0.0208395441149821,0.180860825645154,
3.12616592844986));
#31842=CARTESIAN_POINT('Ctrl Pts',(0.162834335224968,0.0814242232005321,
3.11826869392403));
#31843=CARTESIAN_POINT('Ctrl Pts',(0.157198753896076,-0.0918339622660831,
3.1103714593982));
#31844=CARTESIAN_POINT('Ctrl Pts',(0.00904218304404205,-0.181832790711041,
3.10247422487235));
#31845=CARTESIAN_POINT('Ctrl Pts',(-0.128179738775568,-0.116136573115574,
3.09554334762));
#31846=CARTESIAN_POINT('Ctrl Pts',(-0.153931296515552,-0.0322914212547928,
3.09124488187626));
#31847=CARTESIAN_POINT('Ctrl Pts',(-0.154122750472518,9.83954699399839E-5,
3.08957882764113));
#31848=CARTESIAN_POINT('Origin',(0.,0.,3.71042117235887));
#31849=CARTESIAN_POINT('',(-0.154541524340359,2.74150270591633E-5,3.18957882764113));
#31850=CARTESIAN_POINT('',(-0.154057549710717,2.67855146112065E-5,3.18542117235887));
#31851=CARTESIAN_POINT('',(-0.1543,1.43283619370552E-14,3.71042117235887));
#31852=CARTESIAN_POINT('Ctrl Pts',(-0.154057549710717,2.67855146112127E-5,
3.18542117235887));
#31853=CARTESIAN_POINT('Ctrl Pts',(-0.154095052553054,0.0239637717781011,
3.18419121693124));
#31854=CARTESIAN_POINT('Ctrl Pts',(-0.137617732079011,0.0990829983563936,
3.18032884999499));
#31855=CARTESIAN_POINT('Ctrl Pts',(-0.0208395446762738,0.180860830516292,
3.17383407155014));
#31856=CARTESIAN_POINT('Ctrl Pts',(0.140048991174337,0.116323715159066,
3.1659368370243));
#31857=CARTESIAN_POINT('Ctrl Pts',(0.173965014144346,-0.0536758837012937,
3.15803960249847));
#31858=CARTESIAN_POINT('Ctrl Pts',(0.050159265511441,-0.175011355976434,
3.15014236797263));
#31859=CARTESIAN_POINT('Ctrl Pts',(-0.111453603442084,-0.139367747346172,
3.14260289125943));
#31860=CARTESIAN_POINT('Ctrl Pts',(-0.154092081585972,-0.0438798036810342,
3.13769582605485));
#31861=CARTESIAN_POINT('Ctrl Pts',(-0.154442743231391,0.000107782702043087,
3.13542117235887));
#31862=CARTESIAN_POINT('Ctrl Pts',(-0.154541524340359,2.74150270592019E-5,
3.18957882764113));
#31863=CARTESIAN_POINT('Ctrl Pts',(-0.154545265409953,0.0015398273092893,
3.18950048664627));
#31864=CARTESIAN_POINT('Ctrl Pts',(-0.153842769766794,0.0538687068697594,
3.1867897341428));
#31865=CARTESIAN_POINT('Ctrl Pts',(-0.0949831605760139,0.155316206684809,
3.18144657013072));
#31866=CARTESIAN_POINT('Ctrl Pts',(0.0781262740357409,0.164442117954189,
3.17354933560488));
#31867=CARTESIAN_POINT('Ctrl Pts',(0.180404142828019,0.0244799939226929,
3.16565210107904));
#31868=CARTESIAN_POINT('Ctrl Pts',(0.119122337560023,-0.137676408822293,
3.15775486655321));
#31869=CARTESIAN_POINT('Ctrl Pts',(-0.0501592641604809,-0.175011351262844,
3.14985763202737));
#31870=CARTESIAN_POINT('Ctrl Pts',(-0.145141798308845,-0.081923988470417,
3.14379895239001));
#31871=CARTESIAN_POINT('Ctrl Pts',(-0.15432341073188,-0.0155415899851509,
3.14037268426126));
#31872=CARTESIAN_POINT('Ctrl Pts',(-0.154200664638475,-0.000127870236170063,
3.13957882764113));
#31873=CARTESIAN_POINT('Origin',(0.,0.,3.71042117235887));
#31874=CARTESIAN_POINT('',(-0.154128903346263,0.000101814369117867,3.23957882764113));
#31875=CARTESIAN_POINT('',(-0.15434822268538,-0.000133055250486845,3.23542117235887));
#31876=CARTESIAN_POINT('',(-0.1543,1.43283619370552E-14,3.71042117235887));
#31877=CARTESIAN_POINT('Ctrl Pts',(-0.15434822268538,-0.00013305525048684,
3.23542117235887));
#31878=CARTESIAN_POINT('Ctrl Pts',(-0.153979802923996,0.0405832940781535,
3.23331901931624));
#31879=CARTESIAN_POINT('Ctrl Pts',(-0.116638046803031,0.132884381239301,
3.228584454765));
#31880=CARTESIAN_POINT('Ctrl Pts',(0.0386800589242284,0.177901039004767,
3.22121747870515));
#31881=CARTESIAN_POINT('Ctrl Pts',(0.170109141545278,0.0648676082500797,
3.21332024417931));
#31882=CARTESIAN_POINT('Ctrl Pts',(0.147312299474883,-0.106976694007524,
3.20542300965349));
#31883=CARTESIAN_POINT('Ctrl Pts',(-0.00904218328755787,-0.18183279560836,
3.19752577512764));
#31884=CARTESIAN_POINT('Ctrl Pts',(-0.134124100441736,-0.105850839905797,
3.19085849602944));
#31885=CARTESIAN_POINT('Ctrl Pts',(-0.154014787112897,-0.0272673514852388,
3.18682362843985));
#31886=CARTESIAN_POINT('Ctrl Pts',(-0.154057549710717,2.67855146112127E-5,
3.18542117235887));
#31887=CARTESIAN_POINT('Ctrl Pts',(-0.154128903346263,0.000101814369117853,
3.23957882764113));
#31888=CARTESIAN_POINT('Ctrl Pts',(-0.15424221981892,0.0185794122284465,
3.23862828903127));
#31889=CARTESIAN_POINT('Ctrl Pts',(-0.142646569905461,0.0880912185498955,
3.23504533891281));
#31890=CARTESIAN_POINT('Ctrl Pts',(-0.0397402758525677,0.177667203859151,
3.22882997728572));
#31891=CARTESIAN_POINT('Ctrl Pts',(0.127042092635782,0.130404108641901,
3.22093274275989));
#31892=CARTESIAN_POINT('Ctrl Pts',(0.178644383007786,-0.0350871667669908,
3.21303550823405));
#31893=CARTESIAN_POINT('Ctrl Pts',(0.0682824490586963,-0.1687673902225,
3.20513827370822));
#31894=CARTESIAN_POINT('Ctrl Pts',(-0.102277435139451,-0.149629907004419,
3.19731938017724));
#31895=CARTESIAN_POINT('Ctrl Pts',(-0.154419558113643,-0.0492801999911546,
3.19213289815488));
#31896=CARTESIAN_POINT('Ctrl Pts',(-0.154541524340359,2.74150270592019E-5,
3.18957882764113));
#31897=CARTESIAN_POINT('Origin',(0.,0.,3.71042117235887));
#31898=CARTESIAN_POINT('',(-0.154192638571573,-0.000125942848695916,3.28957882764113));
#31899=CARTESIAN_POINT('',(-0.154450609193756,0.000104390085258889,3.28542117235887));
#31900=CARTESIAN_POINT('',(-0.1543,1.43283619370552E-14,3.71042117235887));
#31901=CARTESIAN_POINT('Ctrl Pts',(-0.154450609193756,0.000104390085258887,
3.28542117235887));
#31902=CARTESIAN_POINT('Ctrl Pts',(-0.154502116257734,0.0067159788236037,
3.28507923320986));
#31903=CARTESIAN_POINT('Ctrl Pts',(-0.151125396911172,0.064173784678776,
3.28210488255223));
#31904=CARTESIAN_POINT('Ctrl Pts',(-0.0791055310066521,0.163973295391393,
3.27649812038601));
#31905=CARTESIAN_POINT('Ctrl Pts',(0.0940552521182287,0.155879877425964,
3.26860088586016));
#31906=CARTESIAN_POINT('Ctrl Pts',(0.181942791852133,0.00646120193221371,
3.26070365133433));
#31907=CARTESIAN_POINT('Ctrl Pts',(0.104875673303493,-0.148815388271832,
3.25280641680849));
#31908=CARTESIAN_POINT('Ctrl Pts',(-0.067274799061048,-0.169171593503912,
3.24490918228266));
#31909=CARTESIAN_POINT('Ctrl Pts',(-0.148843209204449,-0.0715602003700874,
3.23911410079945));
#31910=CARTESIAN_POINT('Ctrl Pts',(-0.154441154880871,-0.0104035676716175,
3.23595143082485));
#31911=CARTESIAN_POINT('Ctrl Pts',(-0.15434822268538,-0.00013305525048684,
3.23542117235887));
#31912=CARTESIAN_POINT('Ctrl Pts',(-0.154192638571573,-0.000125942848695916,
3.28957882764113));
#31913=CARTESIAN_POINT('Ctrl Pts',(-0.153916116413885,0.0352694274746551,
3.28775609141628));
#31914=CARTESIAN_POINT('Ctrl Pts',(-0.124284613860796,0.122201478629219,
3.28330094368282));
#31915=CARTESIAN_POINT('Ctrl Pts',(0.0197606171930289,0.18098188544746,
3.27621338444074));
#31916=CARTESIAN_POINT('Ctrl Pts',(0.162345869645737,0.0823938314495476,
3.26831614991491));
#31917=CARTESIAN_POINT('Ctrl Pts',(0.157743606844976,-0.0908948807772195,
3.26041891538907));
#31918=CARTESIAN_POINT('Ctrl Pts',(0.0101263748965706,-0.181775634735301,
3.25252168086324));
#31919=CARTESIAN_POINT('Ctrl Pts',(-0.127798960265965,-0.1167508316284,
3.24557498494725));
#31920=CARTESIAN_POINT('Ctrl Pts',(-0.153928402385683,-0.0325922506078629,
3.24126070053988));
#31921=CARTESIAN_POINT('Ctrl Pts',(-0.154128903346263,0.000101814369117853,
3.23957882764113));
#31922=CARTESIAN_POINT('Origin',(0.,0.,3.71042117235887));
#31923=CARTESIAN_POINT('',(-0.154543726005254,2.19441315424396E-5,3.33957882764113));
#31924=CARTESIAN_POINT('',(-0.154059302102979,3.16189515402649E-5,3.33542117235887));
#31925=CARTESIAN_POINT('',(-0.1543,1.43283619370552E-14,3.71042117235887));
#31926=CARTESIAN_POINT('Ctrl Pts',(-0.154059302102979,3.16189515402656E-5,
3.33542117235887));
#31927=CARTESIAN_POINT('Ctrl Pts',(-0.15410303154311,0.0236600756904899,
3.33420703559487));
#31928=CARTESIAN_POINT('Ctrl Pts',(-0.137922930779561,0.0984614290803482,
3.33036048732225));
#31929=CARTESIAN_POINT('Ctrl Pts',(-0.0219177305069036,0.180733338725286,
3.32388152754101));
#31930=CARTESIAN_POINT('Ctrl Pts',(0.139352809018331,0.117156823343995,
3.31598429301518));
#31931=CARTESIAN_POINT('Ctrl Pts',(0.174282014774141,-0.0526374957955154,
3.30808705848934));
#31932=CARTESIAN_POINT('Ctrl Pts',(0.0512020468814229,-0.174709121205821,
3.3001898239635));
#31933=CARTESIAN_POINT('Ctrl Pts',(-0.110960029365619,-0.139957157472604,
3.29263452858669));
#31934=CARTESIAN_POINT('Ctrl Pts',(-0.154105590184654,-0.0441832011483282,
3.28771164471847));
#31935=CARTESIAN_POINT('Ctrl Pts',(-0.154450609193756,0.000104390085258887,
3.28542117235887));
#31936=CARTESIAN_POINT('Ctrl Pts',(-0.154543726005254,2.19441315424298E-5,
3.33957882764113));
#31937=CARTESIAN_POINT('Ctrl Pts',(-0.154546150302478,0.00122892294348618,
3.33951630530989));
#31938=CARTESIAN_POINT('Ctrl Pts',(-0.153988815888461,0.0532516871969489,
3.33682137147005));
#31939=CARTESIAN_POINT('Ctrl Pts',(-0.0959076936642258,0.154747016604558,
3.33149402612159));
#31940=CARTESIAN_POINT('Ctrl Pts',(0.0771442407770374,0.164905096849345,
3.32359679159575));
#31941=CARTESIAN_POINT('Ctrl Pts',(0.180254949482897,0.0255553915814562,
3.31569955706992));
#31942=CARTESIAN_POINT('Ctrl Pts',(0.119941247180243,-0.13696357938087,
3.30780232254408));
#31943=CARTESIAN_POINT('Ctrl Pts',(-0.0491146989958762,-0.175307362065916,
3.29990508801825));
#31944=CARTESIAN_POINT('Ctrl Pts',(-0.144900102757682,-0.0825465196247692,
3.29383058971726));
#31945=CARTESIAN_POINT('Ctrl Pts',(-0.154315472118983,-0.0158488741865795,
3.29038850292489));
#31946=CARTESIAN_POINT('Ctrl Pts',(-0.154192638571573,-0.000125942848695916,
3.28957882764113));
#31947=CARTESIAN_POINT('Origin',(0.,0.,3.71042117235887));
#31948=CARTESIAN_POINT('',(-0.15413527741405,0.000105101588974824,3.38957882764113));
#31949=CARTESIAN_POINT('',(-0.15433909720242,-0.000134243687139869,3.38542117235887));
#31950=CARTESIAN_POINT('',(-0.1543,1.43283619370552E-14,3.71042117235887));
#31951=CARTESIAN_POINT('Ctrl Pts',(-0.15433909720242,-0.000134243687139867,
3.38542117235887));
#31952=CARTESIAN_POINT('Ctrl Pts',(-0.153972537455045,0.0402818685502336,
3.38333483797987));
#31953=CARTESIAN_POINT('Ctrl Pts',(-0.117095500692927,0.132285100657941,
3.37861609209226));
#31954=CARTESIAN_POINT('Ctrl Pts',(0.0376184653398806,0.178128542640067,
3.37126493469602));
#31955=CARTESIAN_POINT('Ctrl Pts',(0.169719281325138,0.0658808939206553,
3.36336770017019));
#31956=CARTESIAN_POINT('Ctrl Pts',(0.14794763130091,-0.10609630073556,3.35547046564435));
#31957=CARTESIAN_POINT('Ctrl Pts',(-0.00795766983708003,-0.181883485034118,
3.34757323111852));
#31958=CARTESIAN_POINT('Ctrl Pts',(-0.133788315045723,-0.106470301039161,
3.34089013335669));
#31959=CARTESIAN_POINT('Ctrl Pts',(-0.154008220246,-0.0275695907640756,
3.33683944710348));
#31960=CARTESIAN_POINT('Ctrl Pts',(-0.154059302102979,3.16189515402656E-5,
3.33542117235887));
#31961=CARTESIAN_POINT('Ctrl Pts',(-0.15413527741405,0.000105101588974825,
3.38957882764113));
#31962=CARTESIAN_POINT('Ctrl Pts',(-0.154250615308729,0.0182733082008614,
3.3886441076949));
#31963=CARTESIAN_POINT('Ctrl Pts',(-0.142908820182152,0.0874685218643051,
3.38507697624006));
#31964=CARTESIAN_POINT('Ctrl Pts',(-0.0407990805348497,0.177427055099143,
3.3788774332766));
#31965=CARTESIAN_POINT('Ctrl Pts',(0.126262173896246,0.131159400329288,
3.37098019875077));
#31966=CARTESIAN_POINT('Ctrl Pts',(0.178850447353964,-0.0340212041663437,
3.36308296422493));
#31967=CARTESIAN_POINT('Ctrl Pts',(0.0692876725278909,-0.168357189593675,
3.3551857296991));
#31968=CARTESIAN_POINT('Ctrl Pts',(-0.101728594599068,-0.150200514568663,
3.3473510175045));
#31969=CARTESIAN_POINT('Ctrl Pts',(-0.15444407880598,-0.0495891584122831,
3.3421487168185));
#31970=CARTESIAN_POINT('Ctrl Pts',(-0.154543726005254,2.19441315424298E-5,
3.33957882764113));
#31971=CARTESIAN_POINT('Origin',(0.,0.,3.71042117235887));
#31972=CARTESIAN_POINT('',(-0.154184766718537,-0.000123847547745311,3.43957882764113));
#31973=CARTESIAN_POINT('',(-0.154458280286029,0.000100830356962909,3.43542117235887));
#31974=CARTESIAN_POINT('',(-0.1543,1.43283619370552E-14,3.71042117235887));
#31975=CARTESIAN_POINT('Ctrl Pts',(-0.154458280286029,0.000100830356962935,
3.43542117235887));
#31976=CARTESIAN_POINT('Ctrl Pts',(-0.154506161619621,0.00640573612334919,
3.43509505187348));
#31977=CARTESIAN_POINT('Ctrl Pts',(-0.151303896650316,0.0635541898545394,
3.43213651987949));
#31978=CARTESIAN_POINT('Ctrl Pts',(-0.0800819726320239,0.163498636922,3.42654557637688));
#31979=CARTESIAN_POINT('Ctrl Pts',(0.0931239962001525,0.156438000435139,
3.41864834185104));
#31980=CARTESIAN_POINT('Ctrl Pts',(0.181901025498224,0.00754609564814438,
3.41075110732521));
#31981=CARTESIAN_POINT('Ctrl Pts',(0.10576126311461,-0.148187320169658,
3.40285387279937));
#31982=CARTESIAN_POINT('Ctrl Pts',(-0.0662647547190597,-0.169569775965683,
3.39495663827354));
#31983=CARTESIAN_POINT('Ctrl Pts',(-0.148638055997427,-0.0721814340714305,
3.3891457381267));
#31984=CARTESIAN_POINT('Ctrl Pts',(-0.154435040545295,-0.0107127563084332,
3.38596724948848));
#31985=CARTESIAN_POINT('Ctrl Pts',(-0.15433909720242,-0.000134243687139867,
3.38542117235887));
#31986=CARTESIAN_POINT('Ctrl Pts',(-0.154184766718538,-0.000123847547745311,
3.43957882764113));
#31987=CARTESIAN_POINT('Ctrl Pts',(-0.153916198856604,0.0349688764624186,
3.4377719100799));
#31988=CARTESIAN_POINT('Ctrl Pts',(-0.124690442079412,0.121591245361209,
3.43333258101007));
#31989=CARTESIAN_POINT('Ctrl Pts',(0.0186809873893989,0.181096509168673,
3.42626084043161));
#31990=CARTESIAN_POINT('Ctrl Pts',(0.161851630600137,0.0833605094034181,
3.41836360590578));
#31991=CARTESIAN_POINT('Ctrl Pts',(0.158282849894819,-0.0899525667211824,
3.41046637137994));
#31992=CARTESIAN_POINT('Ctrl Pts',(0.0112102066414966,-0.181712014270169,
3.40256913685411));
#31993=CARTESIAN_POINT('Ctrl Pts',(-0.127415402859048,-0.117364684067358,
3.3956066222745));
#31994=CARTESIAN_POINT('Ctrl Pts',(-0.153925794165715,-0.032893029234098,
3.39127651920351));
#31995=CARTESIAN_POINT('Ctrl Pts',(-0.15413527741405,0.000105101588974825,
3.38957882764113));
#31996=CARTESIAN_POINT('Origin',(0.,0.,3.71042117235887));
#31997=CARTESIAN_POINT('',(-0.154545466983052,1.64397697926255E-5,3.48957882764113));
#31998=CARTESIAN_POINT('',(-0.154061344734167,3.6410572125671E-5,3.48542117235887));
#31999=CARTESIAN_POINT('',(-0.1543,1.43283619370552E-14,3.71042117235887));
#32000=CARTESIAN_POINT('Ctrl Pts',(-0.154061344734167,3.64105721256669E-5,
3.48542117235887));
#32001=CARTESIAN_POINT('Ctrl Pts',(-0.154111085743468,0.0233562467547802,
3.48422285425849));
#32002=CARTESIAN_POINT('Ctrl Pts',(-0.13822562008929,0.0978397409961887,
3.48039212464949));
#32003=CARTESIAN_POINT('Ctrl Pts',(-0.0229951370022999,0.180599416102118,
3.47392898353189));
#32004=CARTESIAN_POINT('Ctrl Pts',(0.138651671100891,0.117985766817156,
3.46603174900605));
#32005=CARTESIAN_POINT('Ctrl Pts',(0.174592817347261,-0.0515972368462645,
3.45813451448022));
#32006=CARTESIAN_POINT('Ctrl Pts',(0.0522430073621133,-0.174400672749591,
3.45023727995438));
#32007=CARTESIAN_POINT('Ctrl Pts',(-0.110463377019167,-0.140545639944236,
3.44266616591394));
#32008=CARTESIAN_POINT('Ctrl Pts',(-0.15411966834722,-0.0444868242763973,
3.4377274633821));
#32009=CARTESIAN_POINT('Ctrl Pts',(-0.154458280286029,0.000100830356962935,
3.43542117235887));
#32010=CARTESIAN_POINT('Ctrl Pts',(-0.154545466983052,1.64397697926493E-5,
3.48957882764113));
#32011=CARTESIAN_POINT('Ctrl Pts',(-0.154546843102601,0.000918015954509084,
3.48953212397352));
#32012=CARTESIAN_POINT('Ctrl Pts',(-0.154132992535152,0.0526348504359433,
3.4868530087973));
#32013=CARTESIAN_POINT('Ctrl Pts',(-0.0968288031440013,0.15417230277993,
3.48154148211247));
#32014=CARTESIAN_POINT('Ctrl Pts',(0.0761594573579975,0.165362221823523,
3.47364424758663));
#32015=CARTESIAN_POINT('Ctrl Pts',(0.180099349163956,0.0266298748857393,
3.46574701306079));
#32016=CARTESIAN_POINT('Ctrl Pts',(0.120755889508211,-0.136245876208876,
3.45784977853496));
#32017=CARTESIAN_POINT('Ctrl Pts',(-0.0480683862207756,-0.175597139874519,
3.44995254400912));
#32018=CARTESIAN_POINT('Ctrl Pts',(-0.144656135320296,-0.0831690899066176,
3.44386222704451));
#32019=CARTESIAN_POINT('Ctrl Pts',(-0.154307462490191,-0.0161560295849065,
3.44040432158851));
#32020=CARTESIAN_POINT('Ctrl Pts',(-0.154184766718538,-0.000123847547745311,
3.43957882764113));
#32021=CARTESIAN_POINT('Origin',(0.,0.,3.71042117235887));
#32022=CARTESIAN_POINT('',(-0.154141660315178,0.000107924336747972,3.53957882764113));
#32023=CARTESIAN_POINT('',(-0.154329957770701,-0.000135440264844456,3.53542117235887));
#32024=CARTESIAN_POINT('',(-0.1543,1.43283619370552E-14,3.71042117235887));
#32025=CARTESIAN_POINT('Ctrl Pts',(-0.154329957770701,-0.000135440264844458,
3.53542117235887));
#32026=CARTESIAN_POINT('Ctrl Pts',(-0.153965757190248,0.0399803656323286,
3.5333506566435));
#32027=CARTESIAN_POINT('Ctrl Pts',(-0.117549955642843,0.13168538088825,
3.52864772941951));
#32028=CARTESIAN_POINT('Ctrl Pts',(0.0365555273815534,0.178349539831362,
3.52131239068689));
#32029=CARTESIAN_POINT('Ctrl Pts',(0.169323388748115,0.0668919258489962,
3.51341515616108));
#32030=CARTESIAN_POINT('Ctrl Pts',(0.148577699872602,-0.105212180693424,
3.50551792163523));
#32031=CARTESIAN_POINT('Ctrl Pts',(-0.00687287246844015,-0.181927682017732,
3.4976206871094));
#32032=CARTESIAN_POINT('Ctrl Pts',(-0.133449900938225,-0.107089534990244,
3.49092177068394));
#32033=CARTESIAN_POINT('Ctrl Pts',(-0.154001816923033,-0.0278717244546827,
3.4868552657671));
#32034=CARTESIAN_POINT('Ctrl Pts',(-0.154061344734167,3.64105721256669E-5,
3.48542117235887));
#32035=CARTESIAN_POINT('Ctrl Pts',(-0.154141660315178,0.000107924336747963,
3.53957882764113));
#32036=CARTESIAN_POINT('Ctrl Pts',(-0.154258987201045,0.017967079764623,
3.53865992635852));
#32037=CARTESIAN_POINT('Ctrl Pts',(-0.14316956514131,0.0868471600938436,
3.53510861356731));
#32038=CARTESIAN_POINT('Ctrl Pts',(-0.0418557834629445,0.177179558878914,
3.52892488926748));
#32039=CARTESIAN_POINT('Ctrl Pts',(0.125477426630257,0.13191056683484,3.52102765474164));
#32040=CARTESIAN_POINT('Ctrl Pts',(0.179050327003836,-0.0329543119327003,
3.51313042021581));
#32041=CARTESIAN_POINT('Ctrl Pts',(0.0702903405429243,-0.167940855985405,
3.50523318568997));
#32042=CARTESIAN_POINT('Ctrl Pts',(-0.101176526834898,-0.15076997316947,
3.49738265483174));
#32043=CARTESIAN_POINT('Ctrl Pts',(-0.154469279323916,-0.0498985397050101,
3.49216453548213));
#32044=CARTESIAN_POINT('Ctrl Pts',(-0.154545466983052,1.64397697926493E-5,
3.48957882764113));
#32045=CARTESIAN_POINT('Origin',(0.,0.,3.71042117235887));
#32046=CARTESIAN_POINT('',(-0.154140927489633,-0.000180264065019253,3.58957882764113));
#32047=CARTESIAN_POINT('',(-0.15446591465964,9.2330361050462E-5,3.58542117235887));
#32048=CARTESIAN_POINT('',(-0.1543,1.43283619370552E-14,3.71042117235887));
#32049=CARTESIAN_POINT('',(-0.0398513841857247,-0.149064942821851,3.6));
#32050=CARTESIAN_POINT('Ctrl Pts',(-0.0398513841857247,-0.149064942821851,
3.6));
#32051=CARTESIAN_POINT('Ctrl Pts',(-0.0891618565331957,-0.135882161272422,
3.59736758849139));
#32052=CARTESIAN_POINT('Ctrl Pts',(-0.14437796139003,-0.0838321271698221,
3.59389386437176));
#32053=CARTESIAN_POINT('Ctrl Pts',(-0.154259564981832,-0.0165262407662603,
3.59042014025214));
#32054=CARTESIAN_POINT('Ctrl Pts',(-0.154140927489633,-0.000180264065019272,
3.58957882764113));
#32055=CARTESIAN_POINT('',(0.0399440158046003,-0.149318575284508,3.6));
#32056=CARTESIAN_POINT('Origin',(0.,0.,3.6));
#32057=CARTESIAN_POINT('Ctrl Pts',(0.0399441988940755,-0.14931907659749,
3.6));
#32058=CARTESIAN_POINT('Ctrl Pts',(-0.00742263582378978,-0.161856507480607,
3.59746250047314));
#32059=CARTESIAN_POINT('Ctrl Pts',(-0.110807703402812,-0.13923343552822,
3.59260289125943));
#32060=CARTESIAN_POINT('Ctrl Pts',(-0.154134073844742,-0.0447846479172299,
3.58774328204572));
#32061=CARTESIAN_POINT('Ctrl Pts',(-0.15446591465964,9.23303610504333E-5,
3.58542117235887));
#32062=CARTESIAN_POINT('Origin',(-1.70916393953233E-17,-6.81365885416763E-18,
2.7));
#32063=CARTESIAN_POINT('Ctrl Pts',(-0.0958116152722464,0.0825211298936403,
2.7));
#32064=CARTESIAN_POINT('Ctrl Pts',(-0.100666302508711,0.0779874972024075,
2.7));
#32065=CARTESIAN_POINT('Ctrl Pts',(-0.10511524090547,0.0730607151536329,
2.7));
#32066=CARTESIAN_POINT('Ctrl Pts',(-0.109154515912936,0.0678088625732328,
2.7));
#32067=CARTESIAN_POINT('Ctrl Pts',(-0.111628556611506,0.0645921226872924,
2.7));
#32068=CARTESIAN_POINT('Ctrl Pts',(-0.113949938179476,0.0612512837881844,
2.7));
#32069=CARTESIAN_POINT('Ctrl Pts',(-0.116112529388643,0.0578058814506189,
2.7));
#32070=CARTESIAN_POINT('Ctrl Pts',(-0.120278296492253,0.0511690544554421,
2.7));
#32071=CARTESIAN_POINT('Ctrl Pts',(-0.123843133570631,0.0441670378484578,
2.7));
#32072=CARTESIAN_POINT('Ctrl Pts',(-0.126794163478656,0.0368991818833284,
2.7));
#32073=CARTESIAN_POINT('Ctrl Pts',(-0.128540684647383,0.0325978143303114,
2.7));
#32074=CARTESIAN_POINT('Ctrl Pts',(-0.130072629552482,0.0281986906446855,
2.7));
#32075=CARTESIAN_POINT('Ctrl Pts',(-0.13137784724267,0.0237479033105473,
2.7));
#32076=CARTESIAN_POINT('Ctrl Pts',(-0.134168070532741,0.0142332525574809,
2.7));
#32077=CARTESIAN_POINT('Ctrl Pts',(-0.135935427906691,0.00446386180413974,
2.7));
#32078=CARTESIAN_POINT('Ctrl Pts',(-0.136643098733652,-0.00537896296213896,
2.7));
#32079=CARTESIAN_POINT('Ctrl Pts',(-0.136956933956429,-0.00974402223206864,
2.7));
#32080=CARTESIAN_POINT('Ctrl Pts',(-0.137061776691848,-0.0141238933117977,
2.7));
#32081=CARTESIAN_POINT('Ctrl Pts',(-0.136951314304003,-0.0185038366743994,
2.7));
#32082=CARTESIAN_POINT('Ctrl Pts',(-0.136873618225507,-0.0215845633357163,
2.7));
#32083=CARTESIAN_POINT('Ctrl Pts',(-0.13668911286562,-0.0246638039330577,
2.7));
#32084=CARTESIAN_POINT('Ctrl Pts',(-0.136397287648127,-0.0277243541204411,
2.7));
#32085=CARTESIAN_POINT('Ctrl Pts',(-0.136038403631432,-0.031488191097877,
2.7));
#32086=CARTESIAN_POINT('Ctrl Pts',(-0.135517191903042,-0.0352286565107813,
2.7));
#32087=CARTESIAN_POINT('Ctrl Pts',(-0.134831588718299,-0.0389361603135121,
2.7));
#32088=CARTESIAN_POINT('Ctrl Pts',(-0.133471069242182,-0.0462933769129071,
2.7));
#32089=CARTESIAN_POINT('Ctrl Pts',(-0.131464409754198,-0.0535208830833808,
2.7));
#32090=CARTESIAN_POINT('Ctrl Pts',(-0.128873836850864,-0.0605679807942907,
2.7));
#32091=CARTESIAN_POINT('Ctrl Pts',(-0.127324936193114,-0.064781432678084,
2.7));
#32092=CARTESIAN_POINT('Ctrl Pts',(-0.125566934259419,-0.0689304108686299,
2.7));
#32093=CARTESIAN_POINT('Ctrl Pts',(-0.123610254975486,-0.0730036509543968,
2.7));
#32094=CARTESIAN_POINT('Ctrl Pts',(-0.122225010943685,-0.0758873281953399,
2.7));
#32095=CARTESIAN_POINT('Ctrl Pts',(-0.120744058613202,-0.0787247786003408,
2.7));
#32096=CARTESIAN_POINT('Ctrl Pts',(-0.11917349881759,-0.0815104554030709,
2.7));
#32097=CARTESIAN_POINT('Ctrl Pts',(-0.115042560220701,-0.0888374351557691,
2.7));
#32098=CARTESIAN_POINT('Ctrl Pts',(-0.11029123440495,-0.095810889712998,
2.7));
#32099=CARTESIAN_POINT('Ctrl Pts',(-0.104997440961948,-0.102362839712403,
2.7));
#32100=CARTESIAN_POINT('Ctrl Pts',(-0.101348653506344,-0.106878821158406,
2.7));
#32101=CARTESIAN_POINT('Ctrl Pts',(-0.0974416313653614,-0.11119454456931,
2.7));
#32102=CARTESIAN_POINT('Ctrl Pts',(-0.09329635857045,-0.115285413781573,
2.7));
#32103=CARTESIAN_POINT('Ctrl Pts',(-0.0904535089763086,-0.118090953116413,
2.7));
#32104=CARTESIAN_POINT('Ctrl Pts',(-0.0874964288334564,-0.12079189694507,
2.7));
#32105=CARTESIAN_POINT('Ctrl Pts',(-0.0844493327259437,-0.123365242468763,
2.7));
#32106=CARTESIAN_POINT('Ctrl Pts',(-0.0762097423121146,-0.130323773594913,
2.7));
#32107=CARTESIAN_POINT('Ctrl Pts',(-0.0672905965515622,-0.136377649112853,
2.7));
#32108=CARTESIAN_POINT('Ctrl Pts',(-0.0578267373609757,-0.141381851878944,
2.7));
#32109=CARTESIAN_POINT('Ctrl Pts',(-0.0536817029967175,-0.143573620798307,
2.7));
#32110=CARTESIAN_POINT('Ctrl Pts',(-0.0494316342727489,-0.145563646977507,
2.7));
#32111=CARTESIAN_POINT('Ctrl Pts',(-0.0450857388735961,-0.147337358046063,
2.7));
#32112=CARTESIAN_POINT('Ctrl Pts',(-0.043386269574786,-0.148030970576765,
2.7));
#32113=CARTESIAN_POINT('Ctrl Pts',(-0.0416721350945774,-0.148691483593437,
2.7));
#32114=CARTESIAN_POINT('Ctrl Pts',(-0.0399441884684126,-0.149319082708151,
2.7));
#32115=CARTESIAN_POINT('Ctrl Pts',(0.0398513841857358,-0.149064942821848,
2.7));
#32116=CARTESIAN_POINT('Ctrl Pts',(0.0462200530662091,-0.146737857425647,
2.7));
#32117=CARTESIAN_POINT('Ctrl Pts',(0.0524055534681357,-0.143963403134301,
2.7));
#32118=CARTESIAN_POINT('Ctrl Pts',(0.0583783483111506,-0.140779078044469,
2.7));
#32119=CARTESIAN_POINT('Ctrl Pts',(0.062793202477668,-0.138425350642158,
2.7));
#32120=CARTESIAN_POINT('Ctrl Pts',(0.067091772966825,-0.135847508755531,
2.7));
#32121=CARTESIAN_POINT('Ctrl Pts',(0.0712602009478766,-0.133058650089746,
2.7));
#32122=CARTESIAN_POINT('Ctrl Pts',(0.0751200675142575,-0.130476232360243,
2.7));
#32123=CARTESIAN_POINT('Ctrl Pts',(0.078861342939135,-0.127717307612303,
2.7));
#32124=CARTESIAN_POINT('Ctrl Pts',(0.0824683178131891,-0.124797523957272,
2.7));
#32125=CARTESIAN_POINT('Ctrl Pts',(0.0880430571667216,-0.12028486905563,
2.7));
#32126=CARTESIAN_POINT('Ctrl Pts',(0.093301870580488,-0.115385246850429,
2.7));
#32127=CARTESIAN_POINT('Ctrl Pts',(0.098201122907525,-0.11013722292202,
2.7));
#32128=CARTESIAN_POINT('Ctrl Pts',(0.100467267721939,-0.107709754113023,
2.7));
#32129=CARTESIAN_POINT('Ctrl Pts',(0.102654039344122,-0.10520989028497,
2.7));
#32130=CARTESIAN_POINT('Ctrl Pts',(0.104752062819345,-0.102648267464436,
2.7));
#32131=CARTESIAN_POINT('Ctrl Pts',(0.111288676944248,-0.0946672605266598,
2.7));
#32132=CARTESIAN_POINT('Ctrl Pts',(0.11698432795861,-0.0860702972477514,
2.7));
#32133=CARTESIAN_POINT('Ctrl Pts',(0.121705201609602,-0.0769745632194894,
2.7));
#32134=CARTESIAN_POINT('Ctrl Pts',(0.12379312017453,-0.0729517586830322,
2.7));
#32135=CARTESIAN_POINT('Ctrl Pts',(0.125689731189231,-0.0688311600363216,
2.7));
#32136=CARTESIAN_POINT('Ctrl Pts',(0.127380076370131,-0.0646223264534606,
2.7));
#32137=CARTESIAN_POINT('Ctrl Pts',(0.128615050131834,-0.0615473337827676,
2.7));
#32138=CARTESIAN_POINT('Ctrl Pts',(0.129739752069541,-0.0584245102417657,
2.7));
#32139=CARTESIAN_POINT('Ctrl Pts',(0.130743760465559,-0.0552728510655911,
2.7));
#32140=CARTESIAN_POINT('Ctrl Pts',(0.131931576408969,-0.0515442059342363,
2.7));
#32141=CARTESIAN_POINT('Ctrl Pts',(0.132952645794869,-0.0477702728539015,
2.7));
#32142=CARTESIAN_POINT('Ctrl Pts',(0.13379905511372,-0.0439575955102323,
2.7));
#32143=CARTESIAN_POINT('Ctrl Pts',(0.135238114697535,-0.0374753064460584,
2.7));
#32144=CARTESIAN_POINT('Ctrl Pts',(0.136172820012768,-0.0308808878255892,
2.7));
#32145=CARTESIAN_POINT('Ctrl Pts',(0.136617245503396,-0.0242291498972301,
2.7));
#32146=CARTESIAN_POINT('Ctrl Pts',(0.136949796542121,-0.0192518423303904,
2.7));
#32147=CARTESIAN_POINT('Ctrl Pts',(0.13700760567975,-0.0142424066500717,
2.7));
#32148=CARTESIAN_POINT('Ctrl Pts',(0.136793131026844,-0.00922497436481165,
2.7));
#32149=CARTESIAN_POINT('Ctrl Pts',(0.136645101058571,-0.00576195282855203,
2.7));
#32150=CARTESIAN_POINT('Ctrl Pts',(0.1363675285007,-0.00230375513318918,
2.7));
#32151=CARTESIAN_POINT('Ctrl Pts',(0.13596351343207,0.00113554936727295,
2.7));
#32152=CARTESIAN_POINT('Ctrl Pts',(0.13510375104742,0.00845454528710606,
2.7));
#32153=CARTESIAN_POINT('Ctrl Pts',(0.133671961121794,0.0156977511556185,
2.7));
#32154=CARTESIAN_POINT('Ctrl Pts',(0.131684102868306,0.0227886248739312,
2.7));
#32155=CARTESIAN_POINT('Ctrl Pts',(0.130343128964387,0.0275720024591066,
2.7));
#32156=CARTESIAN_POINT('Ctrl Pts',(0.128748781223598,0.0322859803615266,
2.7));
#32157=CARTESIAN_POINT('Ctrl Pts',(0.126902487239724,0.0369045444632721,
2.7));
#32158=CARTESIAN_POINT('Ctrl Pts',(0.125403567336896,0.0406541410687207,
2.7));
#32159=CARTESIAN_POINT('Ctrl Pts',(0.123736334503949,0.0443441630809861,
2.7));
#32160=CARTESIAN_POINT('Ctrl Pts',(0.121913684068145,0.047935992310073,
2.7));
#32161=CARTESIAN_POINT('Ctrl Pts',(0.117743460752234,0.0561540958496606,
2.7));
#32162=CARTESIAN_POINT('Ctrl Pts',(0.112753744605352,0.0638862445298334,
2.7));
#32163=CARTESIAN_POINT('Ctrl Pts',(0.106960788703284,0.0709645017846505,
2.7));
#32164=CARTESIAN_POINT('Ctrl Pts',(0.104535029275377,0.0739284720891533,
2.7));
#32165=CARTESIAN_POINT('Ctrl Pts',(0.101968022916162,0.0767773427076814,
2.7));
#32166=CARTESIAN_POINT('Ctrl Pts',(0.0992594073891335,0.0794964656217155,
2.7));
#32167=CARTESIAN_POINT('Ctrl Pts',(0.0981919726164135,0.0805680412369242,
2.7));
#32168=CARTESIAN_POINT('Ctrl Pts',(0.0971025353237707,0.0816194476022307,
2.7));
#32169=CARTESIAN_POINT('Ctrl Pts',(0.0959918005672169,0.0826503307119895,
2.7));
#32170=CARTESIAN_POINT('Origin',(0.,0.,3.71042117235887));
#32171=CARTESIAN_POINT('Ctrl Pts',(-0.15446591465964,9.23303610504368E-5,
3.58542117235887));
#32172=CARTESIAN_POINT('Ctrl Pts',(-0.154510258305412,0.00608920819750747,
3.58511087053711));
#32173=CARTESIAN_POINT('Ctrl Pts',(-0.151481073290489,0.0629168758661166,
3.58216815720674));
#32174=CARTESIAN_POINT('Ctrl Pts',(-0.0810549264538156,0.163034932450524,
3.57659303236775));
#32175=CARTESIAN_POINT('Ctrl Pts',(0.0921890963056651,0.156981846810788,
3.56869579784192));
#32176=CARTESIAN_POINT('Ctrl Pts',(0.181852962765875,0.00863524897295638,
3.56079856331608));
#32177=CARTESIAN_POINT('Ctrl Pts',(0.10664300202618,-0.147556335146073,
3.55290132879024));
#32178=CARTESIAN_POINT('Ctrl Pts',(-0.0652523071804818,-0.169960705131912,
3.54500409426442));
#32179=CARTESIAN_POINT('Ctrl Pts',(-0.1484307843993,-0.072802923531341,
3.53917737545395));
#32180=CARTESIAN_POINT('Ctrl Pts',(-0.154428794390259,-0.0110220529132785,
3.53598306815211));
#32181=CARTESIAN_POINT('Ctrl Pts',(-0.154329957770701,-0.000135440264844458,
3.53542117235887));
#32182=CARTESIAN_POINT('Ctrl Pts',(-0.154140927489633,-0.000180264065019272,
3.58957882764113));
#32183=CARTESIAN_POINT('Ctrl Pts',(-0.153888356116389,0.0346192390763322,
3.58778772874353));
#32184=CARTESIAN_POINT('Ctrl Pts',(-0.125147291545086,0.121067307783401,
3.58336421833732));
#32185=CARTESIAN_POINT('Ctrl Pts',(0.0176337902165689,0.181151815132919,
3.5763082964225));
#32186=CARTESIAN_POINT('Ctrl Pts',(0.161334465098627,0.0843516096779105,
3.56841106189666));
#32187=CARTESIAN_POINT('Ctrl Pts',(0.158825384561566,-0.0890212772063117,
3.56051382737082));
#32188=CARTESIAN_POINT('Ctrl Pts',(0.0122890037691484,-0.181634540286447,
3.55261659284499));
#32189=CARTESIAN_POINT('Ctrl Pts',(-0.127027468209772,-0.117980653400407,
3.54563825960175));
#32190=CARTESIAN_POINT('Ctrl Pts',(-0.153922876401689,-0.0331947231106458,
3.54129233786714));
#32191=CARTESIAN_POINT('Ctrl Pts',(-0.154141660315178,0.000107924336747963,
3.53957882764113));
#32192=CARTESIAN_POINT('Ctrl Pts',(0.0958116152722374,0.0825211298936506,
3.6));
#32193=CARTESIAN_POINT('Ctrl Pts',(0.12310948837823,0.0508267830136165,
3.59736758849139));
#32194=CARTESIAN_POINT('Ctrl Pts',(0.143341746937054,-0.0412253317476725,
3.59210276547417));
#32195=CARTESIAN_POINT('Ctrl Pts',(0.0436608358730345,-0.142764465257081,
3.58420553094833));
#32196=CARTESIAN_POINT('Ctrl Pts',(-0.0955856094744946,-0.114504131671876,
3.57630829642249));
#32197=CARTESIAN_POINT('Ctrl Pts',(-0.148178789486409,0.0173870346414916,
3.56841106189666));
#32198=CARTESIAN_POINT('Ctrl Pts',(-0.066425116332372,0.133608342244775,
3.56051382737082));
#32199=CARTESIAN_POINT('Ctrl Pts',(0.0755496515090821,0.128647793449282,
3.55261659284499));
#32200=CARTESIAN_POINT('Ctrl Pts',(0.149029858339241,0.0070766508919659,
3.54471935831915));
#32201=CARTESIAN_POINT('Ctrl Pts',(0.0873947349721999,-0.120923516391581,
3.53682212379332));
#32202=CARTESIAN_POINT('Ctrl Pts',(-0.0534747520607383,-0.13928406457505,
3.52892488926748));
#32203=CARTESIAN_POINT('Ctrl Pts',(-0.145862599457632,-0.0313691495625942,
3.52102765474165));
#32204=CARTESIAN_POINT('Ctrl Pts',(-0.106007076394109,0.104987796417131,
3.5131304202158));
#32205=CARTESIAN_POINT('Ctrl Pts',(0.029957527138026,0.146158777133349,
3.50523318568998));
#32206=CARTESIAN_POINT('Ctrl Pts',(0.138761779048601,0.0548184317796861,
3.49733595116414));
#32207=CARTESIAN_POINT('Ctrl Pts',(0.121760532397217,-0.0862221662260755,
3.4894387166383));
#32208=CARTESIAN_POINT('Ctrl Pts',(-0.0056323702114988,-0.149091091323021,
3.48154148211246));
#32209=CARTESIAN_POINT('Ctrl Pts',(-0.127918803859021,-0.0767897408219312,
3.47364424758663));
#32210=CARTESIAN_POINT('Ctrl Pts',(-0.134230305961673,0.0651314716709306,
3.46574701306079));
#32211=CARTESIAN_POINT('Ctrl Pts',(-0.0188446861564537,0.148002567505592,
3.45784977853496));
#32212=CARTESIAN_POINT('Ctrl Pts',(0.113626077839972,0.0966902152561852,
3.44995254400912));
#32213=CARTESIAN_POINT('Ctrl Pts',(0.143080115058725,-0.0422843201504222,
3.44205530948329));
#32214=CARTESIAN_POINT('Ctrl Pts',(0.0428135339010967,-0.142922651128878,
3.43415807495745));
#32215=CARTESIAN_POINT('Ctrl Pts',(-0.0962690497602299,-0.113983126411312,
3.42626084043161));
#32216=CARTESIAN_POINT('Ctrl Pts',(-0.148071296290933,0.0182968362857149,
3.41836360590578));
#32217=CARTESIAN_POINT('Ctrl Pts',(-0.0656277734239754,0.133988351515145,
3.41046637137994));
#32218=CARTESIAN_POINT('Ctrl Pts',(0.076315808940436,0.128202107291143,
3.40256913685411));
#32219=CARTESIAN_POINT('Ctrl Pts',(0.149069246106613,0.0061840816248079,
3.39467190232827));
#32220=CARTESIAN_POINT('Ctrl Pts',(0.086672143362556,-0.121440613321149,
3.38677466780244));
#32221=CARTESIAN_POINT('Ctrl Pts',(-0.0543044603643882,-0.138963695209725,
3.37887743327661));
#32222=CARTESIAN_POINT('Ctrl Pts',(-0.14604705151224,-0.0304982252781714,
3.37098019875076));
#32223=CARTESIAN_POINT('Ctrl Pts',(-0.105379112789235,0.105617827984774,
3.36308296422493));
#32224=CARTESIAN_POINT('Ctrl Pts',(0.0308286127169663,0.145977668287988,
3.35518572969909));
#32225=CARTESIAN_POINT('Ctrl Pts',(0.139086215966064,0.0539898835791761,
3.34728849517326));
#32226=CARTESIAN_POINT('Ctrl Pts',(0.121244186506805,-0.0869467091899644,
3.33939126064743));
#32227=CARTESIAN_POINT('Ctrl Pts',(-0.00652136974010873,-0.149054871565549,
3.33149402612159));
#32228=CARTESIAN_POINT('Ctrl Pts',(-0.12837446138172,-0.0760255264081264,
3.32359679159575));
#32229=CARTESIAN_POINT('Ctrl Pts',(-0.133839510420159,0.0659307853068325,
3.31569955706992));
#32230=CARTESIAN_POINT('Ctrl Pts',(-0.0179617435035512,0.148112318093405,
3.30780232254408));
#32231=CARTESIAN_POINT('Ctrl Pts',(0.114200665588904,0.0960108899018034,
3.29990508801825));
#32232=CARTESIAN_POINT('Ctrl Pts',(0.142825410033637,-0.0431368201123976,
3.29200785349241));
#32233=CARTESIAN_POINT('Ctrl Pts',(0.0419604590288785,-0.143175426937629,
3.28411061896658));
#32234=CARTESIAN_POINT('Ctrl Pts',(-0.0969470717891682,-0.113407002747589,
3.27621338444074));
#32235=CARTESIAN_POINT('Ctrl Pts',(-0.147959550895179,0.0191795281376522,
3.26831614991491));
#32236=CARTESIAN_POINT('Ctrl Pts',(-0.0648275722345507,0.134377337668448,
3.26041891538907));
#32237=CARTESIAN_POINT('Ctrl Pts',(0.0770789801059626,0.127744721325426,
3.25252168086324));
#32238=CARTESIAN_POINT('Ctrl Pts',(0.149103473944927,0.00529500313887513,
3.24462444633739));
#32239=CARTESIAN_POINT('Ctrl Pts',(0.085946395912033,-0.121955319811881,
3.23672721181157));
#32240=CARTESIAN_POINT('Ctrl Pts',(-0.0551321992305218,-0.138637381714645,
3.22882997728572));
#32241=CARTESIAN_POINT('Ctrl Pts',(-0.146226329520922,-0.0296267371731131,
3.22093274275989));
#32242=CARTESIAN_POINT('Ctrl Pts',(-0.104747391252292,0.106244374093527,
3.21303550823405));
#32243=CARTESIAN_POINT('Ctrl Pts',(0.0316985965714106,0.145791227363271,
3.20513827370822));
#32244=CARTESIAN_POINT('Ctrl Pts',(0.139405709322103,0.0531594884201076,
3.19724103918239));
#32245=CARTESIAN_POINT('Ctrl Pts',(0.12072352734024,-0.0876681980379225,
3.18934380465655));
#32246=CARTESIAN_POINT('Ctrl Pts',(-0.00741013659566878,-0.149013331203351,
3.18144657013072));
#32247=CARTESIAN_POINT('Ctrl Pts',(-0.128825553891948,-0.0752586185437851,
3.17354933560487));
#32248=CARTESIAN_POINT('Ctrl Pts',(-0.133443954917441,0.0667277595658497,
3.16565210107904));
#32249=CARTESIAN_POINT('Ctrl Pts',(-0.0170781621796165,0.148216798566333,
3.15775486655321));
#32250=CARTESIAN_POINT('Ctrl Pts',(0.114771192054407,0.0953281515350871,
3.14985763202737));
#32251=CARTESIAN_POINT('Ctrl Pts',(0.14256562565491,-0.0439877867403021,
3.14196039750153));
#32252=CARTESIAN_POINT('Ctrl Pts',(0.0411058919243144,-0.143423110584706,
3.1340631629757));
#32253=CARTESIAN_POINT('Ctrl Pts',(-0.0976216460800827,-0.112826846172802,
3.12616592844987));
#32254=CARTESIAN_POINT('Ctrl Pts',(-0.147842543583951,0.0200615380096788,
3.11826869392402));
#32255=CARTESIAN_POINT('Ctrl Pts',(-0.0640250655728793,0.134761544882338,
3.11037145939819));
#32256=CARTESIAN_POINT('Ctrl Pts',(0.0778394100992752,0.127282792380129,
3.10247422487235));
#32257=CARTESIAN_POINT('Ctrl Pts',(0.14913239918967,0.00440573633107837,
3.09457699034652));
#32258=CARTESIAN_POINT('Ctrl Pts',(0.0852175919350427,-0.122465689176514,
3.08667975582068));
#32259=CARTESIAN_POINT('Ctrl Pts',(-0.0559579774207319,-0.138306137838011,
3.07878252129485));
#32260=CARTESIAN_POINT('Ctrl Pts',(-0.14640040725691,-0.028754195445133,
3.07088528676901));
#32261=CARTESIAN_POINT('Ctrl Pts',(-0.104111944565534,0.106867141813886,
3.06298805224318));
#32262=CARTESIAN_POINT('Ctrl Pts',(0.0325674531231242,0.145599601640112,
3.05509081771734));
#32263=CARTESIAN_POINT('Ctrl Pts',(0.139720244968427,0.0523272027405333,
3.04719358319151));
#32264=CARTESIAN_POINT('Ctrl Pts',(0.120198574861694,-0.0883865691262194,
3.03929634866567));
#32265=CARTESIAN_POINT('Ctrl Pts',(-0.00829863992324496,-0.148966491453986,
3.03139911413983));
#32266=CARTESIAN_POINT('Ctrl Pts',(-0.129272064956395,-0.0744890342439453,
3.023501879614));
#32267=CARTESIAN_POINT('Ctrl Pts',(-0.133043653723939,0.0675223607738245,
3.01560464508816));
#32268=CARTESIAN_POINT('Ctrl Pts',(-0.0161939735020032,0.148316007979255,
3.00770741056233));
#32269=CARTESIAN_POINT('Ctrl Pts',(0.115337636891868,0.0946420229965858,
2.9998101760365));
#32270=CARTESIAN_POINT('Ctrl Pts',(0.142300771189819,-0.0448371890228274,
2.99191294151066));
#32271=CARTESIAN_POINT('Ctrl Pts',(0.040249862963706,-0.14366569365053,
2.98401570698482));
#32272=CARTESIAN_POINT('Ctrl Pts',(-0.0982927486352741,-0.112242677117094,
2.97611847245899));
#32273=CARTESIAN_POINT('Ctrl Pts',(-0.14772027852239,0.0209428344297273,
2.96822123793315));
#32274=CARTESIAN_POINT('Ctrl Pts',(-0.0632202819765869,0.135140959547726,
2.96032400340732));
#32275=CARTESIAN_POINT('Ctrl Pts',(0.0785970718760291,0.126816336854618,
2.95242676888148));
#32276=CARTESIAN_POINT('Ctrl Pts',(0.149156020812652,0.00351631284117927,
2.94452953435565));
#32277=CARTESIAN_POINT('Ctrl Pts',(0.0844857573500313,-0.122971703272108,
2.93663229982981));
#32278=CARTESIAN_POINT('Ctrl Pts',(-0.0567817655678681,-0.137969975356402,
2.92873506530398));
#32279=CARTESIAN_POINT('Ctrl Pts',(-0.146569278528953,-0.0278806311257436,
2.92083783077813));
#32280=CARTESIAN_POINT('Ctrl Pts',(-0.103472795328523,0.107486108997575,
2.91294059625231));
#32281=CARTESIAN_POINT('Ctrl Pts',(0.0334351514749053,0.145402797936144,
2.90504336172646));
#32282=CARTESIAN_POINT('Ctrl Pts',(0.140029811715087,0.0514930561329736,
2.89714612720063));
#32283=CARTESIAN_POINT('Ctrl Pts',(0.119669347747977,-0.0891017968949556,
2.88924889267479));
#32284=CARTESIAN_POINT('Ctrl Pts',(-0.00918684813991898,-0.148914354007184,
2.88135165814896));
#32285=CARTESIAN_POINT('Ctrl Pts',(-0.129713978666681,-0.073716800831252,
2.87345442362312));
#32286=CARTESIAN_POINT('Ctrl Pts',(-0.132638621131497,0.0683145605832212,
2.86555718909729));
#32287=CARTESIAN_POINT('Ctrl Pts',(-0.0153092088077737,0.148409942975243,
2.85765995457145));
#32288=CARTESIAN_POINT('Ctrl Pts',(0.11589997974986,0.0939525283576191,
2.84976272004561));
#32289=CARTESIAN_POINT('Ctrl Pts',(0.14203085645546,-0.0456849961183085,
2.84186548551979));
#32290=CARTESIAN_POINT('Ctrl Pts',(0.0393924018242494,-0.143903168728488,
2.83396825099394));
#32291=CARTESIAN_POINT('Ctrl Pts',(-0.0989603541143928,-0.111654514006987,
2.82607101646811));
#32292=CARTESIAN_POINT('Ctrl Pts',(-0.14759276289462,0.0218233815372009,
2.81817378194227));
#32293=CARTESIAN_POINT('Ctrl Pts',(-0.0624132446091692,0.135515576866934,
2.81027654741644));
#32294=CARTESIAN_POINT('Ctrl Pts',(0.0793519279903814,0.126345354605138,
2.8023793128906));
#32295=CARTESIAN_POINT('Ctrl Pts',(0.149174358180394,0.00262679649731067,
2.79448207836477));
#32296=CARTESIAN_POINT('Ctrl Pts',(0.0837508793007237,-0.12347340605925,
2.78658484383893));
#32297=CARTESIAN_POINT('Ctrl Pts',(-0.0576034595552612,-0.137628787005506,
2.7786876093131));
#32298=CARTESIAN_POINT('Ctrl Pts',(-0.146733081304572,-0.0270063046901533,
2.77079037478726));
#32299=CARTESIAN_POINT('Ctrl Pts',(-0.102829689230287,0.108101695072837,
2.76289314026143));
#32300=CARTESIAN_POINT('Ctrl Pts',(0.0343011276704797,0.145199973805224,
2.75499590573559));
#32301=CARTESIAN_POINT('Ctrl Pts',(0.140335424370929,0.0506587128142576,
2.74709867120975));
#32302=CARTESIAN_POINT('Ctrl Pts',(0.11913389087728,-0.0898170012241629,
2.73920143668392));
#32303=CARTESIAN_POINT('Ctrl Pts',(-0.0100709312277202,-0.14885086814231,
2.73130420215808));
#32304=CARTESIAN_POINT('Ctrl Pts',(-0.130158589013459,-0.0729535941759648,
2.72340696763225));
#32305=CARTESIAN_POINT('Ctrl Pts',(-0.132214800612389,0.0691267612890124,
2.71550973310641));
#32306=CARTESIAN_POINT('Ctrl Pts',(-0.0144510241825876,0.148455288920992,
2.70761249858058));
#32307=CARTESIAN_POINT('Ctrl Pts',(0.116510849855331,0.0933444320528056,
2.69971526405474));
#32308=CARTESIAN_POINT('Ctrl Pts',(0.141650318794474,-0.0467072968399595,
2.6918180295289));
#32309=CARTESIAN_POINT('Ctrl Pts',(0.073068805953493,-0.111356443894342,
2.68655320651168));
#32310=CARTESIAN_POINT('Ctrl Pts',(0.0326585063531192,-0.122159831625552,
2.68392079500307));
#32311=CARTESIAN_POINT('Ctrl Pts',(0.102845629995664,0.088579422941069,
3.60535973499898));
#32312=CARTESIAN_POINT('Ctrl Pts',(0.132147577876935,0.0545582339347427,
3.60272732349037));
#32313=CARTESIAN_POINT('Ctrl Pts',(0.153865188751202,-0.0442518916242316,
3.59746250047314));
#32314=CARTESIAN_POINT('Ctrl Pts',(0.046866198411756,-0.153245525906639,
3.58956526594731));
#32315=CARTESIAN_POINT('Ctrl Pts',(-0.102603031970513,-0.122910458459966,
3.58166803142147));
#32316=CARTESIAN_POINT('Ctrl Pts',(-0.159057343031147,0.0186635046949134,
3.57377079689563));
#32317=CARTESIAN_POINT('Ctrl Pts',(-0.0713017197061865,0.143417205646691,
3.5658735623698));
#32318=CARTESIAN_POINT('Ctrl Pts',(0.0810961331079431,0.138092477903117,
3.55797632784396));
#32319=CARTESIAN_POINT('Ctrl Pts',(0.159970893148119,0.00759618358562943,
3.55007909331813));
#32320=CARTESIAN_POINT('Ctrl Pts',(0.0938108239901933,-0.129801122643079,
3.54218185879229));
#32321=CARTESIAN_POINT('Ctrl Pts',(-0.0574006037673195,-0.149509611427338,
3.53428462426646));
#32322=CARTESIAN_POINT('Ctrl Pts',(-0.156571109790821,-0.0336721173108959,
3.52638738974062));
#32323=CARTESIAN_POINT('Ctrl Pts',(-0.113789591426601,0.112695480957047,
3.51849015521479));
#32324=CARTESIAN_POINT('Ctrl Pts',(0.0321568605525351,0.15688903136602,
3.51059292068895));
#32325=CARTESIAN_POINT('Ctrl Pts',(0.148948982281772,0.0588429298027895,
3.50269568616312));
#32326=CARTESIAN_POINT('Ctrl Pts',(0.130699588222345,-0.092552171048525,
3.49479845163728));
#32327=CARTESIAN_POINT('Ctrl Pts',(-0.00604587096381251,-0.160036621554591,
3.48690121711144));
#32328=CARTESIAN_POINT('Ctrl Pts',(-0.137309969504135,-0.0824272636422575,
3.47900398258561));
#32329=CARTESIAN_POINT('Ctrl Pts',(-0.144084830862247,0.0699131020545748,
3.47110674805977));
#32330=CARTESIAN_POINT('Ctrl Pts',(-0.0202281697717358,0.158868183704434,
3.46320951353394));
#32331=CARTESIAN_POINT('Ctrl Pts',(0.121967942260279,0.103788732443176,
3.4553122790081));
#32332=CARTESIAN_POINT('Ctrl Pts',(0.153584349154903,-0.045388625715703,
3.44741504448227));
#32333=CARTESIAN_POINT('Ctrl Pts',(0.0459566917214356,-0.153415325002449,
3.43951780995643));
#32334=CARTESIAN_POINT('Ctrl Pts',(-0.103336647060408,-0.122351203571073,
3.43162057543059));
#32335=CARTESIAN_POINT('Ctrl Pts',(-0.158941958217129,0.0196400994742142,
3.42372334090476));
#32336=CARTESIAN_POINT('Ctrl Pts',(-0.0704458398266582,0.14382511331743,
3.41582610637892));
#32337=CARTESIAN_POINT('Ctrl Pts',(0.0819185380270082,0.137614071672475,
3.40792887185309));
#32338=CARTESIAN_POINT('Ctrl Pts',(0.160013172570483,0.00663808629925336,
3.40003163732726));
#32339=CARTESIAN_POINT('Ctrl Pts',(0.0930351832799072,-0.130356182270652,
3.39213440280141));
#32340=CARTESIAN_POINT('Ctrl Pts',(-0.0582912251492787,-0.149165722128378,
3.38423716827558));
#32341=CARTESIAN_POINT('Ctrl Pts',(-0.15676910340262,-0.0327372540747895,
3.37633993374974));
#32342=CARTESIAN_POINT('Ctrl Pts',(-0.113115525840982,0.11337176632503,
3.36844269922391));
#32343=CARTESIAN_POINT('Ctrl Pts',(0.0330918969246043,0.156694626405347,
3.36054546469807));
#32344=CARTESIAN_POINT('Ctrl Pts',(0.149297237752422,0.0579535536930025,
3.35264823017224));
#32345=CARTESIAN_POINT('Ctrl Pts',(0.130145334771507,-0.0933299063718294,
3.3447509956464));
#32346=CARTESIAN_POINT('Ctrl Pts',(-0.00700013643909911,-0.159997742721738,
3.33685376112057));
#32347=CARTESIAN_POINT('Ctrl Pts',(-0.137799079147585,-0.0816069443874761,
3.32895652659473));
#32348=CARTESIAN_POINT('Ctrl Pts',(-0.143665345045706,0.0707710973426707,
3.3210592920689));
#32349=CARTESIAN_POINT('Ctrl Pts',(-0.019280405838002,0.158985991637365,
3.31316205754306));
#32350=CARTESIAN_POINT('Ctrl Pts',(0.122584713398713,0.103059534382534,
3.30526482301722));
#32351=CARTESIAN_POINT('Ctrl Pts',(0.153310944947138,-0.0463037120067701,
3.29736758849139));
#32352=CARTESIAN_POINT('Ctrl Pts',(0.04504098831306,-0.15368665836036,3.28947035396555));
#32353=CARTESIAN_POINT('Ctrl Pts',(-0.1040644461119,-0.121732783758583,
3.28157311943972));
#32354=CARTESIAN_POINT('Ctrl Pts',(-0.158822009027328,0.0205875941944168,
3.27367588491388));
#32355=CARTESIAN_POINT('Ctrl Pts',(-0.0695868918252512,0.14424265690943,
3.26577865038805));
#32356=CARTESIAN_POINT('Ctrl Pts',(0.0827377374433846,0.137123106692272,
3.25788141586221));
#32357=CARTESIAN_POINT('Ctrl Pts',(0.160049913247329,0.00568373606998795,
3.24998418133638));
#32358=CARTESIAN_POINT('Ctrl Pts',(0.0922561550425197,-0.130908675965198,
3.24208694681054));
#32359=CARTESIAN_POINT('Ctrl Pts',(-0.0591797325073638,-0.148815452311067,
3.2341897122847));
#32360=CARTESIAN_POINT('Ctrl Pts',(-0.156961543115644,-0.0318017856251262,
3.22629247775887));
#32361=CARTESIAN_POINT('Ctrl Pts',(-0.112437426434515,0.114044310348977,
3.21839524323303));
#32362=CARTESIAN_POINT('Ctrl Pts',(0.0340257506890165,0.156494497910436,
3.21049800870719));
#32363=CARTESIAN_POINT('Ctrl Pts',(0.149640186729828,0.0570621950300983,
3.20260077418136));
#32364=CARTESIAN_POINT('Ctrl Pts',(0.129586451385121,-0.094104363361123,
3.19470353965552));
#32365=CARTESIAN_POINT('Ctrl Pts',(-0.00795415215963184,-0.159953152671687,
3.18680630512969));
#32366=CARTESIAN_POINT('Ctrl Pts',(-0.138283288637936,-0.0807837339423469,
3.17890907060385));
#32367=CARTESIAN_POINT('Ctrl Pts',(-0.143240749815163,0.0716265815084065,
3.17101183607802));
#32368=CARTESIAN_POINT('Ctrl Pts',(-0.0183319563451689,0.159098142549652,
3.16311460155218));
#32369=CARTESIAN_POINT('Ctrl Pts',(0.123197125094384,0.10232667274308,3.15521736702635));
#32370=CARTESIAN_POINT('Ctrl Pts',(0.153032088484722,-0.047217152393966,
3.14732013250051));
#32371=CARTESIAN_POINT('Ctrl Pts',(0.0441236831200233,-0.153952525715282,
3.13942289797468));
#32372=CARTESIAN_POINT('Ctrl Pts',(-0.104788544309502,-0.121110034958652,
3.13152566344884));
#32373=CARTESIAN_POINT('Ctrl Pts',(-0.158696411618254,0.021534356867118,
3.123628428923));
#32374=CARTESIAN_POINT('Ctrl Pts',(-0.0687254690952325,0.14465507071593,
3.11573119439717));
#32375=CARTESIAN_POINT('Ctrl Pts',(0.0835539944442463,0.136627265209407,
3.10783395987133));
#32376=CARTESIAN_POINT('Ctrl Pts',(0.160080962040421,0.00472918369319909,
3.0999367253455));
#32377=CARTESIAN_POINT('Ctrl Pts',(0.091473845883615,-0.131456514123307,
3.09203949081966));
#32378=CARTESIAN_POINT('Ctrl Pts',(-0.0600661352464005,-0.148459890147985,
3.08414225629383));
#32379=CARTESIAN_POINT('Ctrl Pts',(-0.157148400777682,-0.0308651862007597,
3.07624502176799));
#32380=CARTESIAN_POINT('Ctrl Pts',(-0.111755328396166,0.114712798593949,
3.06834778724216));
#32381=CARTESIAN_POINT('Ctrl Pts',(0.0349583943897092,0.156288803974834,
3.06045055271632));
#32382=CARTESIAN_POINT('Ctrl Pts',(0.149977814027003,0.0561688070540271,
3.05255331819049));
#32383=CARTESIAN_POINT('Ctrl Pts',(0.129022959493032,-0.0948754737002677,
3.04465608366465));
#32384=CARTESIAN_POINT('Ctrl Pts',(-0.00890788500525998,-0.159902874179684,
3.03675884913881));
#32385=CARTESIAN_POINT('Ctrl Pts',(-0.138762580335427,-0.0799576505710677,
3.02886161461298));
#32386=CARTESIAN_POINT('Ctrl Pts',(-0.142811060488699,0.072479518405434,
3.02096438008714));
#32387=CARTESIAN_POINT('Ctrl Pts',(-0.0173828549097553,0.159204635426789,
3.01306714556131));
#32388=CARTESIAN_POINT('Ctrl Pts',(0.123805155509077,0.101590172042203,
3.00516991103547));
#32389=CARTESIAN_POINT('Ctrl Pts',(0.152747789715287,-0.0481289135892851,
2.99727267650964));
#32390=CARTESIAN_POINT('Ctrl Pts',(0.0432048087487045,-0.154212918029513,
2.9893754419838));
#32391=CARTESIAN_POINT('Ctrl Pts',(-0.105508915893722,-0.120482979101306,
2.98147820745797));
#32392=CARTESIAN_POINT('Ctrl Pts',(-0.158565170460834,0.0224803537097271,
2.97358097293213));
#32393=CARTESIAN_POINT('Ctrl Pts',(-0.067861602269319,0.145062340128731,
2.9656837384063));
#32394=CARTESIAN_POINT('Ctrl Pts',(0.0843672799997867,0.136126564827205,
2.95778650388046));
#32395=CARTESIAN_POINT('Ctrl Pts',(0.160106317846084,0.0037744631314833,
2.94988926935462));
#32396=CARTESIAN_POINT('Ctrl Pts',(0.0906882836244439,-0.131999677270073,
2.94199203482879));
#32397=CARTESIAN_POINT('Ctrl Pts',(-0.0609504018432475,-0.148099048280287,
2.93409480030295));
#32398=CARTESIAN_POINT('Ctrl Pts',(-0.157329669742954,-0.0299274891113821,
2.92619756577712));
#32399=CARTESIAN_POINT('Ctrl Pts',(-0.111069255984644,0.115377207285653,
2.91830033125128));
#32400=CARTESIAN_POINT('Ctrl Pts',(0.0358897948611611,0.156077551916693,
2.91040309672545));
#32401=CARTESIAN_POINT('Ctrl Pts',(0.150310107632486,0.0552734215298454,
2.90250586219961));
#32402=CARTESIAN_POINT('Ctrl Pts',(0.128454879143209,-0.0956432099528824,
2.89460862767377));
#32403=CARTESIAN_POINT('Ctrl Pts',(-0.00986130107440376,-0.159846909059511,
2.88671139314794));
#32404=CARTESIAN_POINT('Ctrl Pts',(-0.139236937163761,-0.079128723602177,
2.8788141586221));
#32405=CARTESIAN_POINT('Ctrl Pts',(-0.142376292407395,0.0733298776050816,
2.87091692409627));
#32406=CARTESIAN_POINT('Ctrl Pts',(-0.0164331351694357,0.159305466665398,
2.86301968957043));
#32407=CARTESIAN_POINT('Ctrl Pts',(0.124408782797267,0.10085005811842,2.85512245504459));
#32408=CARTESIAN_POINT('Ctrl Pts',(0.152458059176653,-0.0490389624868201,
2.84722522051876));
#32409=CARTESIAN_POINT('Ctrl Pts',(0.0422843970550532,-0.154467827352683,
2.83932798599292));
#32410=CARTESIAN_POINT('Ctrl Pts',(-0.106225533663848,-0.11985163596585,
2.83143075146709));
#32411=CARTESIAN_POINT('Ctrl Pts',(-0.158428293266612,0.0234255462289395,
2.82353351694125));
#32412=CARTESIAN_POINT('Ctrl Pts',(-0.0669953162115558,0.145464459997932,
2.81563628241542));
#32413=CARTESIAN_POINT('Ctrl Pts',(0.085177553915074,0.13562100539136,2.80773904788958));
#32414=CARTESIAN_POINT('Ctrl Pts',(0.160126001452633,0.00281964289891892,
2.79984181336375));
#32415=CARTESIAN_POINT('Ctrl Pts',(0.0898994544648863,-0.132538212593453,
2.79194457883791));
#32416=CARTESIAN_POINT('Ctrl Pts',(-0.0618324205375044,-0.147732811568847,
2.78404734431207));
#32417=CARTESIAN_POINT('Ctrl Pts',(-0.157505498107873,-0.028988973955003,
2.77615010978624));
#32418=CARTESIAN_POINT('Ctrl Pts',(-0.110378936218723,0.11603798664468,
2.7682528752604));
#32419=CARTESIAN_POINT('Ctrl Pts',(0.0368193467442185,0.155859837441643,
2.76035564073457));
#32420=CARTESIAN_POINT('Ctrl Pts',(0.150638156857367,0.0543778248529476,
2.75245840620873));
#32421=CARTESIAN_POINT('Ctrl Pts',(0.127880111678472,-0.0964109210451539,
2.7445611716829));
#32422=CARTESIAN_POINT('Ctrl Pts',(-0.0108102891681236,-0.159778762376561,
2.73666393715706));
#32423=CARTESIAN_POINT('Ctrl Pts',(-0.139714188602295,-0.0783094860905571,
2.72876670263123));
#32424=CARTESIAN_POINT('Ctrl Pts',(-0.141921357082812,0.0742017060679738,
2.72086946810539));
#32425=CARTESIAN_POINT('Ctrl Pts',(-0.0155119468753121,0.159354141686116,
2.71297223357956));
#32426=CARTESIAN_POINT('Ctrl Pts',(0.125064499963334,0.100197318391729,
2.70507499905372));
#32427=CARTESIAN_POINT('Ctrl Pts',(0.152049584323474,-0.050136315469175,
2.69717776452788));
#32428=CARTESIAN_POINT('Ctrl Pts',(0.0784331561467309,-0.119531683020366,
2.69191294151066));
#32429=CARTESIAN_POINT('Ctrl Pts',(0.0350561322973247,-0.131128202024318,
2.68928053000205));
#32430=CARTESIAN_POINT('Ctrl Pts',(0.10987964471909,0.0946377159884874,
3.61071946999795));
#32431=CARTESIAN_POINT('Ctrl Pts',(0.14118566737564,0.0582896848558689,
3.60808705848934));
#32432=CARTESIAN_POINT('Ctrl Pts',(0.16438863056535,-0.0472784515007908,
3.60282223547212));
#32433=CARTESIAN_POINT('Ctrl Pts',(0.0500715609504776,-0.163726586556196,
3.59492500094628));
#32434=CARTESIAN_POINT('Ctrl Pts',(-0.109620454466532,-0.131316785248055,
3.58702776642045));
#32435=CARTESIAN_POINT('Ctrl Pts',(-0.169935896575886,0.0199399747483351,
3.57913053189461));
#32436=CARTESIAN_POINT('Ctrl Pts',(-0.0761783230800011,0.153226069048607,
3.57123329736878));
#32437=CARTESIAN_POINT('Ctrl Pts',(0.0866426147068042,0.147537162356952,
3.56333606284294));
#32438=CARTESIAN_POINT('Ctrl Pts',(0.170911927956997,0.00811571627929297,
3.55543882831711));
#32439=CARTESIAN_POINT('Ctrl Pts',(0.100226913008187,-0.138678728894576,
3.54754159379127));
#32440=CARTESIAN_POINT('Ctrl Pts',(-0.0613264554739007,-0.159735158279625,
3.53964435926544));
#32441=CARTESIAN_POINT('Ctrl Pts',(-0.167279620124009,-0.0359750850591977,
3.53174712473959));
#32442=CARTESIAN_POINT('Ctrl Pts',(-0.121572106459094,0.120403165496963,
3.52384989021377));
#32443=CARTESIAN_POINT('Ctrl Pts',(0.0343561939670442,0.167619285598691,
3.51595265568792));
#32444=CARTESIAN_POINT('Ctrl Pts',(0.159136185514944,0.0628674278258929,
3.5080554211621));
#32445=CARTESIAN_POINT('Ctrl Pts',(0.139638644047474,-0.0988821758709744,
3.50015818663625));
#32446=CARTESIAN_POINT('Ctrl Pts',(-0.00645937171612636,-0.170982151786161,
3.49226095211042));
#32447=CARTESIAN_POINT('Ctrl Pts',(-0.146701135149248,-0.0880647864625838,
3.48436371758458));
#32448=CARTESIAN_POINT('Ctrl Pts',(-0.15393935576282,0.074694732438219,
3.47646648305875));
#32449=CARTESIAN_POINT('Ctrl Pts',(-0.0216116533870178,0.169733799903276,
3.46856924853291));
#32450=CARTESIAN_POINT('Ctrl Pts',(0.130309806680585,0.110887249630166,
3.46067201400708));
#32451=CARTESIAN_POINT('Ctrl Pts',(0.164088583251082,-0.0484929312809838,
3.45277477948124));
#32452=CARTESIAN_POINT('Ctrl Pts',(0.0490998495417746,-0.16390799887602,
3.4448775449554));
#32453=CARTESIAN_POINT('Ctrl Pts',(-0.110404244360585,-0.130719280730833,
3.43698031042957));
#32454=CARTESIAN_POINT('Ctrl Pts',(-0.169812620143325,0.0209833626627134,
3.42908307590373));
#32455=CARTESIAN_POINT('Ctrl Pts',(-0.075263906229341,0.153661875119715,
3.4211858413779));
#32456=CARTESIAN_POINT('Ctrl Pts',(0.0875212671135803,0.147026036053807,
3.41328860685206));
#32457=CARTESIAN_POINT('Ctrl Pts',(0.170957099034354,0.00709209097369881,
3.40539137232623));
#32458=CARTESIAN_POINT('Ctrl Pts',(0.0993982231972585,-0.139271751220155,
3.39749413780039));
#32459=CARTESIAN_POINT('Ctrl Pts',(-0.0622779899341693,-0.15936774904703,
3.38959690327456));
#32460=CARTESIAN_POINT('Ctrl Pts',(-0.167491155293001,-0.0349762828714076,
3.38169966874872));
#32461=CARTESIAN_POINT('Ctrl Pts',(-0.120851938892729,0.121125704665286,
3.37380243422289));
#32462=CARTESIAN_POINT('Ctrl Pts',(0.0353551811322426,0.167411584522707,
3.36590519969705));
#32463=CARTESIAN_POINT('Ctrl Pts',(0.15950825953878,0.0619172238068289,
3.35800796517121));
#32464=CARTESIAN_POINT('Ctrl Pts',(0.139046483036208,-0.0997131035536944,
3.35011073064538));
#32465=CARTESIAN_POINT('Ctrl Pts',(-0.00747890313808957,-0.170940613877928,
3.34221349611955));
#32466=CARTESIAN_POINT('Ctrl Pts',(-0.14722369691345,-0.0871883623668259,
3.33431626159371));
#32467=CARTESIAN_POINT('Ctrl Pts',(-0.153491179671254,0.0756114093785092,
3.32641902706787));
#32468=CARTESIAN_POINT('Ctrl Pts',(-0.0205990681724529,0.169859665181325,
3.31852179254204));
#32469=CARTESIAN_POINT('Ctrl Pts',(0.130968761208522,0.110108178863265,
3.3106245580162));
#32470=CARTESIAN_POINT('Ctrl Pts',(0.16379647986064,-0.0494706039011429,
3.30272732349037));
#32471=CARTESIAN_POINT('Ctrl Pts',(0.0481215175972415,-0.16419788978309,
3.29483008896453));
#32472=CARTESIAN_POINT('Ctrl Pts',(-0.111181820434632,-0.130058564769576,
3.2869328544387));
#32473=CARTESIAN_POINT('Ctrl Pts',(-0.169684467159477,0.0219956602511813,
3.27903561991286));
#32474=CARTESIAN_POINT('Ctrl Pts',(-0.0743462114159517,0.154107976150411,
3.27113838538702));
#32475=CARTESIAN_POINT('Ctrl Pts',(0.0883964947808067,0.146501492059118,
3.26324115086119));
#32476=CARTESIAN_POINT('Ctrl Pts',(0.170996352549731,0.00607246900110077,
3.25534391633535));
#32477=CARTESIAN_POINT('Ctrl Pts',(0.0985659141730064,-0.139862032118515,
3.24744668180952));
#32478=CARTESIAN_POINT('Ctrl Pts',(-0.0632272657842059,-0.15899352290749,
3.23954944728368));
#32479=CARTESIAN_POINT('Ctrl Pts',(-0.167696756710366,-0.0339768340771394,
3.23165221275785));
#32480=CARTESIAN_POINT('Ctrl Pts',(-0.120127461616738,0.121844246604426,
3.22375497823201));
#32481=CARTESIAN_POINT('Ctrl Pts',(0.0363529048066224,0.167197768457601,
3.21585774370617));
#32482=CARTESIAN_POINT('Ctrl Pts',(0.159874664137553,0.0609649016400891,
3.20796050918034));
#32483=CARTESIAN_POINT('Ctrl Pts',(0.138449375430002,-0.100540528684324,
3.2000632746545));
#32484=CARTESIAN_POINT('Ctrl Pts',(-0.00849816772359493,-0.170892974140023,
3.19216604012867));
#32485=CARTESIAN_POINT('Ctrl Pts',(-0.147741023383925,-0.0863088493409087,
3.18426880560283));
#32486=CARTESIAN_POINT('Ctrl Pts',(-0.153037544712885,0.0765254034509632,
3.176371571077));
#32487=CARTESIAN_POINT('Ctrl Pts',(-0.0195857505107214,0.169979486532972,
3.16847433655116));
#32488=CARTESIAN_POINT('Ctrl Pts',(0.131623058134361,0.109325193951073,
3.16057710202532));
#32489=CARTESIAN_POINT('Ctrl Pts',(0.163498551314534,-0.0504465180476298,
3.15267986749949));
#32490=CARTESIAN_POINT('Ctrl Pts',(0.0471414743157323,-0.164481940845858,
3.14478263297365));
#32491=CARTESIAN_POINT('Ctrl Pts',(-0.111955442538922,-0.129393223744503,
3.13688539844782));
#32492=CARTESIAN_POINT('Ctrl Pts',(-0.169550279652557,0.0230071757245571,
3.12898816392198));
#32493=CARTESIAN_POINT('Ctrl Pts',(-0.0734258726175858,0.154548596549523,
3.12109092939615));
#32494=CARTESIAN_POINT('Ctrl Pts',(0.0892685787892176,0.145971738038684,
3.11319369487031));
#32495=CARTESIAN_POINT('Ctrl Pts',(0.171029524891172,0.00505263105532012,
3.10529646034447));
#32496=CARTESIAN_POINT('Ctrl Pts',(0.0977300998321875,-0.140447339070101,
3.09739922581864));
#32497=CARTESIAN_POINT('Ctrl Pts',(-0.0641742930720691,-0.158613642457959,
3.0895019912928));
#32498=CARTESIAN_POINT('Ctrl Pts',(-0.167896394298454,-0.0329761769563863,
3.08160475676697));
#32499=CARTESIAN_POINT('Ctrl Pts',(-0.119398712226798,0.122558455374011,
3.07370752224113));
#32500=CARTESIAN_POINT('Ctrl Pts',(0.0373493356562941,0.166978006309557,
3.0658102877153));
#32501=CARTESIAN_POINT('Ctrl Pts',(0.160235383085578,0.0600104113675208,
3.05791305318946));
#32502=CARTESIAN_POINT('Ctrl Pts',(0.13784734412437,-0.101364378274316,
3.05001581866363));
#32503=CARTESIAN_POINT('Ctrl Pts',(-0.00951713008727486,-0.170839256905381,
3.04211858413779));
#32504=CARTESIAN_POINT('Ctrl Pts',(-0.148253095714458,-0.0854262668981903,
3.03422134961195));
#32505=CARTESIAN_POINT('Ctrl Pts',(-0.152578467253459,0.0774366760370435,
3.02632411508612));
#32506=CARTESIAN_POINT('Ctrl Pts',(-0.0185717363175075,0.170093262874324,
3.01842688056029));
#32507=CARTESIAN_POINT('Ctrl Pts',(0.132272674126287,0.10853832108782,3.01052964603445));
#32508=CARTESIAN_POINT('Ctrl Pts',(0.163194808240755,-0.051420638155743,
3.00263241150862));
#32509=CARTESIAN_POINT('Ctrl Pts',(0.0461597545337032,-0.164760142408496,
2.99473517698277));
#32510=CARTESIAN_POINT('Ctrl Pts',(-0.112725083152171,-0.128723281085519,
2.98683794245694));
#32511=CARTESIAN_POINT('Ctrl Pts',(-0.169410062399277,0.024017872989727,
2.9789407079311));
#32512=CARTESIAN_POINT('Ctrl Pts',(-0.0725029225620513,0.154983720709736,
2.97104347340527));
#32513=CARTESIAN_POINT('Ctrl Pts',(0.0901374881235442,0.145436792799793,
2.96314623887944));
#32514=CARTESIAN_POINT('Ctrl Pts',(0.171056614879515,0.00403261342178739,
2.95524900435359));
#32515=CARTESIAN_POINT('Ctrl Pts',(0.0968908098988563,-0.141027651268038,
2.94735176982777));
#32516=CARTESIAN_POINT('Ctrl Pts',(-0.0651190381186268,-0.158228121204172,
2.93945453530192));
#32517=CARTESIAN_POINT('Ctrl Pts',(-0.168090060956955,-0.0319743470970206,
2.93155730077609));
#32518=CARTESIAN_POINT('Ctrl Pts',(-0.118665716640764,0.123268305573731,
2.92366006625025));
#32519=CARTESIAN_POINT('Ctrl Pts',(0.0383444382474168,0.166752305897243,
2.91576283172442));
#32520=CARTESIAN_POINT('Ctrl Pts',(0.160590403549885,0.0590537869267172,
2.90786559719859));
#32521=CARTESIAN_POINT('Ctrl Pts',(0.137240410538441,-0.102184623010809,
2.89996836267275));
#32522=CARTESIAN_POINT('Ctrl Pts',(-0.0105357540088883,-0.170779464111837,
2.89207112814692));
#32523=CARTESIAN_POINT('Ctrl Pts',(-0.14875989566084,-0.0845406463731019,
2.88417389362107));
#32524=CARTESIAN_POINT('Ctrl Pts',(-0.152113963683294,0.0783451946269418,
2.87627665909525));
#32525=CARTESIAN_POINT('Ctrl Pts',(-0.0175570615310977,0.170200990355554,
2.86837942456941));
#32526=CARTESIAN_POINT('Ctrl Pts',(0.132917585844673,0.10774758787922,2.86048219004357));
#32527=CARTESIAN_POINT('Ctrl Pts',(0.162885261897846,-0.0523929288553319,
2.85258495551774));
#32528=CARTESIAN_POINT('Ctrl Pts',(0.0451763922858567,-0.165032485976878,
2.8446877209919));
#32529=CARTESIAN_POINT('Ctrl Pts',(-0.113490713213303,-0.128048757924713,
2.83679048646607));
#32530=CARTESIAN_POINT('Ctrl Pts',(-0.169263823638604,0.0250277109206782,
2.82889325194023));
#32531=CARTESIAN_POINT('Ctrl Pts',(-0.0715773878139425,0.15541334312893,
2.82099601741439));
#32532=CARTESIAN_POINT('Ctrl Pts',(0.0910031798397666,0.144896656177581,
2.81309878288856));
#32533=CARTESIAN_POINT('Ctrl Pts',(0.171077644724872,0.00301248930052715,
2.80520154836272));
#32534=CARTESIAN_POINT('Ctrl Pts',(0.0960480296290492,-0.141603019127657,
2.79730431383689));
#32535=CARTESIAN_POINT('Ctrl Pts',(-0.0660613815197478,-0.157836836132188,
2.78940707931105));
#32536=CARTESIAN_POINT('Ctrl Pts',(-0.168277914911174,-0.0309716432198527,
2.78150984478522));
#32537=CARTESIAN_POINT('Ctrl Pts',(-0.11792818320716,0.123974278216523,
2.77361261025938));
#32538=CARTESIAN_POINT('Ctrl Pts',(0.0393375658179575,0.166519701078062,
2.76571537573355));
#32539=CARTESIAN_POINT('Ctrl Pts',(0.160940889343806,0.0580969368916377,
2.75781814120771));
#32540=CARTESIAN_POINT('Ctrl Pts',(0.136626332479664,-0.103004840866145,
2.74992090668187));
#32541=CARTESIAN_POINT('Ctrl Pts',(-0.011549647108527,-0.170706656610813,
2.74202367215604));
#32542=CARTESIAN_POINT('Ctrl Pts',(-0.149269788191131,-0.0836653780051494,
2.7341264376302));
#32543=CARTESIAN_POINT('Ctrl Pts',(-0.151627913553235,0.0792766508469352,
2.72622920310437));
#32544=CARTESIAN_POINT('Ctrl Pts',(-0.0165728695680367,0.170252994451239,
2.71833196857853));
#32545=CARTESIAN_POINT('Ctrl Pts',(0.133618150071337,0.107050204730652,
2.7104347340527));
#32546=CARTESIAN_POINT('Ctrl Pts',(0.162448849852474,-0.0535653340983903,
2.70253749952686));
#32547=CARTESIAN_POINT('Ctrl Pts',(0.0837975063399687,-0.127706922146391,
2.69727267650963));
#32548=CARTESIAN_POINT('Ctrl Pts',(0.0374537582415302,-0.140096572423083,
2.69464026500102));
#32549=CARTESIAN_POINT('Ctrl Pts',(0.116913659442517,0.100696009035906,
3.61607920499693));
#32550=CARTESIAN_POINT('Ctrl Pts',(0.150223756874345,0.0620211357769951,
3.61344679348832));
#32551=CARTESIAN_POINT('Ctrl Pts',(0.174912072379498,-0.0503050113773498,
3.60818197047109));
#32552=CARTESIAN_POINT('Ctrl Pts',(0.0532769234891989,-0.174207647205754,
3.60028473594526));
#32553=CARTESIAN_POINT('Ctrl Pts',(-0.11663787696255,-0.139723112036145,
3.59238750141943));
#32554=CARTESIAN_POINT('Ctrl Pts',(-0.180814450120624,0.0212164448017569,
3.58449026689359));
#32555=CARTESIAN_POINT('Ctrl Pts',(-0.0810549264538156,0.163034932450524,
3.57659303236775));
#32556=CARTESIAN_POINT('Ctrl Pts',(0.0921890963056651,0.156981846810788,
3.56869579784192));
#32557=CARTESIAN_POINT('Ctrl Pts',(0.181852962765875,0.00863524897295638,
3.56079856331608));
#32558=CARTESIAN_POINT('Ctrl Pts',(0.10664300202618,-0.147556335146073,
3.55290132879024));
#32559=CARTESIAN_POINT('Ctrl Pts',(-0.0652523071804818,-0.169960705131912,
3.54500409426442));
#32560=CARTESIAN_POINT('Ctrl Pts',(-0.177988130457198,-0.0382780528074994,
3.53710685973857));
#32561=CARTESIAN_POINT('Ctrl Pts',(-0.129354621491586,0.128110850036879,
3.52920962521275));
#32562=CARTESIAN_POINT('Ctrl Pts',(0.0365555273815534,0.178349539831362,
3.52131239068689));
#32563=CARTESIAN_POINT('Ctrl Pts',(0.169323388748115,0.0668919258489962,
3.51341515616108));
#32564=CARTESIAN_POINT('Ctrl Pts',(0.148577699872602,-0.105212180693424,
3.50551792163523));
#32565=CARTESIAN_POINT('Ctrl Pts',(-0.00687287246844015,-0.181927682017732,
3.4976206871094));
#32566=CARTESIAN_POINT('Ctrl Pts',(-0.156092300794361,-0.0937023092829102,
3.48972345258356));
#32567=CARTESIAN_POINT('Ctrl Pts',(-0.163793880663394,0.0794763628218631,
3.48182621805772));
#32568=CARTESIAN_POINT('Ctrl Pts',(-0.0229951370022999,0.180599416102118,
3.47392898353189));
#32569=CARTESIAN_POINT('Ctrl Pts',(0.138651671100891,0.117985766817156,
3.46603174900605));
#32570=CARTESIAN_POINT('Ctrl Pts',(0.174592817347261,-0.0515972368462645,
3.45813451448022));
#32571=CARTESIAN_POINT('Ctrl Pts',(0.0522430073621133,-0.174400672749591,
3.45023727995438));
#32572=CARTESIAN_POINT('Ctrl Pts',(-0.117471841660763,-0.139087357890593,
3.44234004542855));
#32573=CARTESIAN_POINT('Ctrl Pts',(-0.180683282069521,0.0223266258512126,
3.43444281090271));
#32574=CARTESIAN_POINT('Ctrl Pts',(-0.0800819726320239,0.163498636922,3.42654557637688));
#32575=CARTESIAN_POINT('Ctrl Pts',(0.0931239962001525,0.156438000435139,
3.41864834185104));
#32576=CARTESIAN_POINT('Ctrl Pts',(0.181901025498224,0.00754609564814438,
3.41075110732521));
#32577=CARTESIAN_POINT('Ctrl Pts',(0.10576126311461,-0.148187320169658,
3.40285387279937));
#32578=CARTESIAN_POINT('Ctrl Pts',(-0.0662647547190597,-0.169569775965683,
3.39495663827354));
#32579=CARTESIAN_POINT('Ctrl Pts',(-0.178213207183381,-0.0372153116680257,
3.3870594037477));
#32580=CARTESIAN_POINT('Ctrl Pts',(-0.128588351944475,0.128879643005541,
3.37916216922186));
#32581=CARTESIAN_POINT('Ctrl Pts',(0.0376184653398806,0.178128542640067,
3.37126493469602));
#32582=CARTESIAN_POINT('Ctrl Pts',(0.169719281325138,0.0658808939206553,
3.36336770017019));
#32583=CARTESIAN_POINT('Ctrl Pts',(0.14794763130091,-0.10609630073556,3.35547046564435));
#32584=CARTESIAN_POINT('Ctrl Pts',(-0.00795766983708003,-0.181883485034118,
3.34757323111852));
#32585=CARTESIAN_POINT('Ctrl Pts',(-0.156648314679315,-0.0927697803461756,
3.33967599659268));
#32586=CARTESIAN_POINT('Ctrl Pts',(-0.163317014296801,0.0804517214143475,
3.33177876206685));
#32587=CARTESIAN_POINT('Ctrl Pts',(-0.0219177305069036,0.180733338725286,
3.32388152754101));
#32588=CARTESIAN_POINT('Ctrl Pts',(0.139352809018331,0.117156823343995,
3.31598429301518));
#32589=CARTESIAN_POINT('Ctrl Pts',(0.174282014774141,-0.0526374957955154,
3.30808705848934));
#32590=CARTESIAN_POINT('Ctrl Pts',(0.0512020468814229,-0.174709121205821,
3.3001898239635));
#32591=CARTESIAN_POINT('Ctrl Pts',(-0.118299194757364,-0.13838434578057,
3.29229258943767));
#32592=CARTESIAN_POINT('Ctrl Pts',(-0.180546925291626,0.0234037263079457,
3.28439535491183));
#32593=CARTESIAN_POINT('Ctrl Pts',(-0.0791055310066521,0.163973295391393,
3.27649812038601));
#32594=CARTESIAN_POINT('Ctrl Pts',(0.0940552521182287,0.155879877425964,
3.26860088586016));
#32595=CARTESIAN_POINT('Ctrl Pts',(0.181942791852133,0.00646120193221371,
3.26070365133433));
#32596=CARTESIAN_POINT('Ctrl Pts',(0.104875673303493,-0.148815388271832,
3.25280641680849));
#32597=CARTESIAN_POINT('Ctrl Pts',(-0.067274799061048,-0.169171593503912,
3.24490918228266));
#32598=CARTESIAN_POINT('Ctrl Pts',(-0.178431970305088,-0.0361518825291525,
3.23701194775682));
#32599=CARTESIAN_POINT('Ctrl Pts',(-0.127817496798961,0.129644182859876,
3.22911471323099));
#32600=CARTESIAN_POINT('Ctrl Pts',(0.0386800589242284,0.177901039004767,
3.22121747870515));
#32601=CARTESIAN_POINT('Ctrl Pts',(0.170109141545278,0.0648676082500797,
3.21332024417931));
#32602=CARTESIAN_POINT('Ctrl Pts',(0.147312299474883,-0.106976694007524,
3.20542300965349));
#32603=CARTESIAN_POINT('Ctrl Pts',(-0.00904218328755787,-0.18183279560836,
3.19752577512764));
#32604=CARTESIAN_POINT('Ctrl Pts',(-0.157198758129913,-0.0918339647394704,
3.18962854060181));
#32605=CARTESIAN_POINT('Ctrl Pts',(-0.162834339610607,0.0814242253935201,
3.18173130607597));
#32606=CARTESIAN_POINT('Ctrl Pts',(-0.0208395446762738,0.180860830516292,
3.17383407155014));
#32607=CARTESIAN_POINT('Ctrl Pts',(0.140048991174337,0.116323715159066,
3.1659368370243));
#32608=CARTESIAN_POINT('Ctrl Pts',(0.173965014144346,-0.0536758837012937,
3.15803960249847));
#32609=CARTESIAN_POINT('Ctrl Pts',(0.050159265511441,-0.175011355976434,
3.15014236797263));
#32610=CARTESIAN_POINT('Ctrl Pts',(-0.119122340768341,-0.137676412530354,
3.14224513344679));
#32611=CARTESIAN_POINT('Ctrl Pts',(-0.180404147686861,0.0244799945819963,
3.13434789892096));
#32612=CARTESIAN_POINT('Ctrl Pts',(-0.0781262761399388,0.164442122383114,
3.12645066439512));
#32613=CARTESIAN_POINT('Ctrl Pts',(0.0949831631341886,0.155316210867962,
3.11855342986929));
#32614=CARTESIAN_POINT('Ctrl Pts',(0.181978087741923,0.00537607841744088,
3.11065619534345));
#32615=CARTESIAN_POINT('Ctrl Pts',(0.10398635378076,-0.149438164016893,
3.10275896081762));
#32616=CARTESIAN_POINT('Ctrl Pts',(-0.0682824508977375,-0.168767394767933,
3.09486172629178));
#32617=CARTESIAN_POINT('Ctrl Pts',(-0.178644387819226,-0.0350871677120128,
3.08696449176594));
#32618=CARTESIAN_POINT('Ctrl Pts',(-0.127042096057429,0.130404112154074,
3.07906725724011));
#32619=CARTESIAN_POINT('Ctrl Pts',(0.039740276922879,0.17766720864428,3.07117002271427));
#32620=CARTESIAN_POINT('Ctrl Pts',(0.170492952144154,0.0638520156810144,
3.06327278818844));
#32621=CARTESIAN_POINT('Ctrl Pts',(0.146671728755708,-0.107853282848364,
3.0553755536626));
#32622=CARTESIAN_POINT('Ctrl Pts',(-0.0101263751692898,-0.181775639631079,
3.04747831913677));
#32623=CARTESIAN_POINT('Ctrl Pts',(-0.15774361109349,-0.0908948832253125,
3.03958108461093));
#32624=CARTESIAN_POINT('Ctrl Pts',(-0.162345874018219,0.0823938336686527,
3.0316838500851));
#32625=CARTESIAN_POINT('Ctrl Pts',(-0.0197606177252597,0.180981890321858,
3.02378661555926));
#32626=CARTESIAN_POINT('Ctrl Pts',(0.140740192743497,0.115486470133437,
3.01588938103343));
#32627=CARTESIAN_POINT('Ctrl Pts',(0.173641826766224,-0.0547123627222005,
3.00799214650759));
#32628=CARTESIAN_POINT('Ctrl Pts',(0.0491147003187017,-0.175307366787479,
3.00009491198175));
#32629=CARTESIAN_POINT('Ctrl Pts',(-0.119941250410619,-0.136963583069732,
2.99219767745592));
#32630=CARTESIAN_POINT('Ctrl Pts',(-0.180254954337721,0.0255553922697266,
2.98430044293008));
#32631=CARTESIAN_POINT('Ctrl Pts',(-0.0771442428547834,0.164905101290741,
2.97640320840425));
#32632=CARTESIAN_POINT('Ctrl Pts',(0.0959076962473017,0.15474702077238,
2.96850597387841));
#32633=CARTESIAN_POINT('Ctrl Pts',(0.182006911912947,0.00429076371209153,
2.96060873935257));
#32634=CARTESIAN_POINT('Ctrl Pts',(0.103093336173269,-0.150055625266004,
2.95271150482674));
#32635=CARTESIAN_POINT('Ctrl Pts',(-0.069287674394006,-0.168357194128057,
2.9448142703009));
#32636=CARTESIAN_POINT('Ctrl Pts',(-0.178850452170956,-0.0340212050826592,
2.93691703577507));
#32637=CARTESIAN_POINT('Ctrl Pts',(-0.126262177296885,0.131159403861809,
2.92901980124923));
#32638=CARTESIAN_POINT('Ctrl Pts',(0.0407990816336726,0.177427059877793,
2.9211225667234));
#32639=CARTESIAN_POINT('Ctrl Pts',(0.170870699467283,0.0628341523235889,
2.91322533219756));
#32640=CARTESIAN_POINT('Ctrl Pts',(0.146025941933673,-0.108726036068736,
2.90532809767173));
#32641=CARTESIAN_POINT('Ctrl Pts',(-0.0112102069433731,-0.181712019164164,
2.89743086314589));
#32642=CARTESIAN_POINT('Ctrl Pts',(-0.158282854157919,-0.0899525691440268,
2.88953362862006));
#32643=CARTESIAN_POINT('Ctrl Pts',(-0.161851634959193,0.0833605116488022,
2.88163639409422));
#32644=CARTESIAN_POINT('Ctrl Pts',(-0.0186809878927599,0.181096514045709,
2.87373915956839));
#32645=CARTESIAN_POINT('Ctrl Pts',(0.14142638889208,0.114645117640021,2.86584192504255));
#32646=CARTESIAN_POINT('Ctrl Pts',(0.173312464619039,-0.0557468952238434,
2.85794469051671));
#32647=CARTESIAN_POINT('Ctrl Pts',(0.0480683875166603,-0.175597144601074,
2.85004745599088));
#32648=CARTESIAN_POINT('Ctrl Pts',(-0.120755892762759,-0.136245879883575,
2.84215022146504));
#32649=CARTESIAN_POINT('Ctrl Pts',(-0.180099354010596,0.0266298756124168,
2.83425298693921));
#32650=CARTESIAN_POINT('Ctrl Pts',(-0.0761594594163292,0.165362226259928,
2.82635575241337));
#32651=CARTESIAN_POINT('Ctrl Pts',(0.0968288057644592,0.154172306963803,
2.81845851788754));
#32652=CARTESIAN_POINT('Ctrl Pts',(0.182029287997112,0.0032053357021354,
2.8105612833617));
#32653=CARTESIAN_POINT('Ctrl Pts',(0.102196604793212,-0.150667825661861,
2.80266404883587));
#32654=CARTESIAN_POINT('Ctrl Pts',(-0.0702903425019912,-0.167940860695529,
2.79476681431002));
#32655=CARTESIAN_POINT('Ctrl Pts',(-0.179050331714475,-0.0329543124847025,
2.7868695797842));
#32656=CARTESIAN_POINT('Ctrl Pts',(-0.125477430195597,0.131910569788365,
2.77897234525835));
#32657=CARTESIAN_POINT('Ctrl Pts',(0.0418557848916964,0.17717956471448,
2.77107511073252));
#32658=CARTESIAN_POINT('Ctrl Pts',(0.171243621830244,0.0618160489303277,
2.76317787620668));
#32659=CARTESIAN_POINT('Ctrl Pts',(0.145372553280857,-0.109598760687136,
2.75528064168085));
#32660=CARTESIAN_POINT('Ctrl Pts',(-0.0122890050489303,-0.181634550845065,
2.74738340715501));
#32661=CARTESIAN_POINT('Ctrl Pts',(-0.158825387779967,-0.0890212699197419,
2.73948617262918));
#32662=CARTESIAN_POINT('Ctrl Pts',(-0.161334470023658,0.0843515956258966,
2.73158893810334));
#32663=CARTESIAN_POINT('Ctrl Pts',(-0.0176337922607613,0.181151847216363,
2.72369170357751));
#32664=CARTESIAN_POINT('Ctrl Pts',(0.14217180017934,0.113903091069576,2.71579446905167));
#32665=CARTESIAN_POINT('Ctrl Pts',(0.172848115381474,-0.0569943527276058,
2.70789723452584));
#32666=CARTESIAN_POINT('Ctrl Pts',(0.0891618565332066,-0.135882161272415,
2.70263241150861));
#32667=CARTESIAN_POINT('Ctrl Pts',(0.0398513841857358,-0.149064942821848,
2.7));
#32668=CARTESIAN_POINT('Ctrl Pts',(0.0958116152722374,0.0825211298936506,
3.6));
#32669=CARTESIAN_POINT('Ctrl Pts',(0.102493614798766,0.0762810303731869,
3.6));
#32670=CARTESIAN_POINT('Ctrl Pts',(0.108396094096263,0.0693090539021388,
3.6));
#32671=CARTESIAN_POINT('Ctrl Pts',(0.113512571306729,0.0617846659987563,
3.6));
#32672=CARTESIAN_POINT('Ctrl Pts',(0.117461600031764,0.0559771498608983,
3.6));
#32673=CARTESIAN_POINT('Ctrl Pts',(0.120942091267611,0.0498392138898472,
3.6));
#32674=CARTESIAN_POINT('Ctrl Pts',(0.123938893544148,0.0434377969520944,
3.6));
#32675=CARTESIAN_POINT('Ctrl Pts',(0.125176287448039,0.0407946214723323,
3.6));
#32676=CARTESIAN_POINT('Ctrl Pts',(0.126329312445263,0.0381097373250835,
3.6));
#32677=CARTESIAN_POINT('Ctrl Pts',(0.12739426777321,0.0353959223183902,
3.6));
#32678=CARTESIAN_POINT('Ctrl Pts',(0.130992400282108,0.0262268372474364,
3.6));
#32679=CARTESIAN_POINT('Ctrl Pts',(0.13360037697833,0.0167048680256365,
3.6));
#32680=CARTESIAN_POINT('Ctrl Pts',(0.135185783736742,0.0070125550480467,
3.6));
#32681=CARTESIAN_POINT('Ctrl Pts',(0.135855615028331,0.00291757154566029,
3.6));
#32682=CARTESIAN_POINT('Ctrl Pts',(0.13634239472836,-0.00120821237992505,
3.6));
#32683=CARTESIAN_POINT('Ctrl Pts',(0.136641151680689,-0.0053522141362822,
3.6));
#32684=CARTESIAN_POINT('Ctrl Pts',(0.136866179264237,-0.00847352962091436,
3.6));
#32685=CARTESIAN_POINT('Ctrl Pts',(0.136984148876184,-0.0116047424016575,
3.6));
#32686=CARTESIAN_POINT('Ctrl Pts',(0.136993305813875,-0.0147266162095009,
3.6));
#32687=CARTESIAN_POINT('Ctrl Pts',(0.1370171880242,-0.0228687756739225,
3.6));
#32688=CARTESIAN_POINT('Ctrl Pts',(0.1363045911537,-0.0309705737407376,
3.6));
#32689=CARTESIAN_POINT('Ctrl Pts',(0.134831565375878,-0.0389361856515032,
3.6));
#32690=CARTESIAN_POINT('Ctrl Pts',(0.133932184221546,-0.043799726631656,
3.6));
#32691=CARTESIAN_POINT('Ctrl Pts',(0.132748938308619,-0.0486126850413777,
3.6));
#32692=CARTESIAN_POINT('Ctrl Pts',(0.131298540463925,-0.0533602760289537,
3.6));
#32693=CARTESIAN_POINT('Ctrl Pts',(0.130441077796828,-0.0561670107778959,
3.6));
#32694=CARTESIAN_POINT('Ctrl Pts',(0.129489770756279,-0.058951963571448,
3.6));
#32695=CARTESIAN_POINT('Ctrl Pts',(0.128448797183808,-0.061708664264176,
3.6));
#32696=CARTESIAN_POINT('Ctrl Pts',(0.124844109667278,-0.0712545786242284,
3.6));
#32697=CARTESIAN_POINT('Ctrl Pts',(0.120197621014249,-0.0803872939153616,
3.6));
#32698=CARTESIAN_POINT('Ctrl Pts',(0.114666430721154,-0.0889848980033025,
3.6));
#32699=CARTESIAN_POINT('Ctrl Pts',(0.111763941762871,-0.0934964858552134,
3.6));
#32700=CARTESIAN_POINT('Ctrl Pts',(0.108616890563154,-0.0978607268708147,
3.6));
#32701=CARTESIAN_POINT('Ctrl Pts',(0.105242483611131,-0.102058774522217,
3.6));
#32702=CARTESIAN_POINT('Ctrl Pts',(0.103051571759935,-0.104784454169668,
3.6));
#32703=CARTESIAN_POINT('Ctrl Pts',(0.100763130867069,-0.107441777418394,
3.6));
#32704=CARTESIAN_POINT('Ctrl Pts',(0.098386472215756,-0.110019467506635,
3.6));
#32705=CARTESIAN_POINT('Ctrl Pts',(0.0926299038901994,-0.116262959438837,
3.6));
#32706=CARTESIAN_POINT('Ctrl Pts',(0.0863771877690887,-0.12201951201926,
3.6));
#32707=CARTESIAN_POINT('Ctrl Pts',(0.0796980248685607,-0.127218319244159,
3.6));
#32708=CARTESIAN_POINT('Ctrl Pts',(0.0749983795646852,-0.130876345006388,
3.6));
#32709=CARTESIAN_POINT('Ctrl Pts',(0.0700820293375014,-0.134260491890013,
3.6));
#32710=CARTESIAN_POINT('Ctrl Pts',(0.064997448628775,-0.137327043702736,
3.6));
#32711=CARTESIAN_POINT('Ctrl Pts',(0.0586168958330981,-0.141175206779031,
3.6));
#32712=CARTESIAN_POINT('Ctrl Pts',(0.0519659322704503,-0.144529310638398,
3.6));
#32713=CARTESIAN_POINT('Ctrl Pts',(0.0450857487477646,-0.147337352418514,
3.6));
#32714=CARTESIAN_POINT('Ctrl Pts',(0.0433856322299594,-0.148031228998597,
3.6));
#32715=CARTESIAN_POINT('Ctrl Pts',(0.0416714833555574,-0.148691718060548,
3.6));
#32716=CARTESIAN_POINT('Ctrl Pts',(0.0399441988940855,-0.149319076597487,
3.6));
#32717=CARTESIAN_POINT('Ctrl Pts',(-0.126474550616365,-0.00011099430647141,
3.51934196736194));
#32718=CARTESIAN_POINT('Ctrl Pts',(-0.126555547962724,-0.00903265450993761,
3.51990386315518));
#32719=CARTESIAN_POINT('Ctrl Pts',(-0.125690900286005,-0.0179387227435883,
3.52046575894841));
#32720=CARTESIAN_POINT('Ctrl Pts',(-0.123822037714229,-0.0266288110680491,
3.52102765474165));
#32721=CARTESIAN_POINT('Ctrl Pts',(-0.115066650325334,-0.0673407879000796,
3.52366006625026));
#32722=CARTESIAN_POINT('Ctrl Pts',(-0.0842707011930362,-0.103312426237565,
3.52629247775887));
#32723=CARTESIAN_POINT('Ctrl Pts',(-0.0453944787880641,-0.118238154042396,
3.52892488926748));
#32724=CARTESIAN_POINT('Ctrl Pts',(-0.00651825638309213,-0.133163881847227,
3.53155730077609));
#32725=CARTESIAN_POINT('Ctrl Pts',(0.0404382392945539,-0.127043699119404,
3.5341897122847));
#32726=CARTESIAN_POINT('Ctrl Pts',(0.0741890076945504,-0.102650246541568,
3.53682212379332));
#32727=CARTESIAN_POINT('Ctrl Pts',(0.107939776094547,-0.0782567939637322,
3.53945453530193));
#32728=CARTESIAN_POINT('Ctrl Pts',(0.128484817216894,-0.0355900715358833,
3.54208694681054));
#32729=CARTESIAN_POINT('Ctrl Pts',(0.126510636639707,0.00600514677092718,
3.54471935831915));
#32730=CARTESIAN_POINT('Ctrl Pts',(0.124536456062521,0.0476003650777378,
3.54735176982776));
#32731=CARTESIAN_POINT('Ctrl Pts',(0.100043053785802,0.0881240792635097,
3.54998418133637));
#32732=CARTESIAN_POINT('Ctrl Pts',(0.0641338913405327,0.109212694488978,
3.55261659284499));
#32733=CARTESIAN_POINT('Ctrl Pts',(0.028224728895264,0.130301309714446,
3.5552490043536));
#32734=CARTESIAN_POINT('Ctrl Pts',(-0.019100193718554,0.13195482597961,
3.55788141586221));
#32735=CARTESIAN_POINT('Ctrl Pts',(-0.0563882672178024,0.113411366178312,
3.56051382737082));
#32736=CARTESIAN_POINT('Ctrl Pts',(-0.0936763407170509,0.0948679063770136,
3.56314623887943));
#32737=CARTESIAN_POINT('Ctrl Pts',(-0.12092756510173,0.0561274705092526,
3.56577865038805));
#32738=CARTESIAN_POINT('Ctrl Pts',(-0.125787647292084,0.0147753915231441,
3.56841106189666));
#32739=CARTESIAN_POINT('Ctrl Pts',(-0.126360541139662,0.00990091600857084,
3.56872136371842));
#32740=CARTESIAN_POINT('Ctrl Pts',(-0.126622308248343,0.0049901515008091,
3.56903166554018));
#32741=CARTESIAN_POINT('Ctrl Pts',(-0.126585968300139,7.56654190205153E-5,
3.56934196736194));
#32742=CARTESIAN_POINT('Ctrl Pts',(-0.0398513841857247,-0.149064942821851,
3.6));
#32743=CARTESIAN_POINT('Ctrl Pts',(-0.0891618565331957,-0.135882161272422,
3.59736758849139));
#32744=CARTESIAN_POINT('Ctrl Pts',(-0.17284812802765,-0.0569944292149041,
3.59210276547417));
#32745=CARTESIAN_POINT('Ctrl Pts',(-0.142171789002704,0.113903133580536,
3.58420553094833));
#32746=CARTESIAN_POINT('Ctrl Pts',(0.0176337902165689,0.181151815132919,
3.5763082964225));
#32747=CARTESIAN_POINT('Ctrl Pts',(0.161334465098627,0.0843516096779105,
3.56841106189666));
#32748=CARTESIAN_POINT('Ctrl Pts',(0.158825384561566,-0.0890212772063117,
3.56051382737082));
#32749=CARTESIAN_POINT('Ctrl Pts',(0.0122890037691484,-0.181634540286447,
3.55261659284499));
#32750=CARTESIAN_POINT('Ctrl Pts',(-0.145372548664834,-0.109598761010981,
3.54471935831915));
#32751=CARTESIAN_POINT('Ctrl Pts',(-0.171243617690229,0.0618160491398297,
3.53682212379332));
#32752=CARTESIAN_POINT('Ctrl Pts',(-0.0418557834629445,0.177179558878914,
3.52892488926748));
#32753=CARTESIAN_POINT('Ctrl Pts',(0.125477426630257,0.13191056683484,3.52102765474164));
#32754=CARTESIAN_POINT('Ctrl Pts',(0.179050327003836,-0.0329543119327003,
3.51313042021581));
#32755=CARTESIAN_POINT('Ctrl Pts',(0.0702903405429243,-0.167940855985405,
3.50523318568997));
#32756=CARTESIAN_POINT('Ctrl Pts',(-0.102196602002365,-0.150667821707605,
3.49733595116413));
#32757=CARTESIAN_POINT('Ctrl Pts',(-0.182029283116568,0.00320533567306586,
3.4894387166383));
#32758=CARTESIAN_POINT('Ctrl Pts',(-0.0968288031440013,0.15417230277993,
3.48154148211247));
#32759=CARTESIAN_POINT('Ctrl Pts',(0.0761594573579975,0.165362221823523,
3.47364424758663));
#32760=CARTESIAN_POINT('Ctrl Pts',(0.180099349163956,0.0266298748857393,
3.46574701306079));
#32761=CARTESIAN_POINT('Ctrl Pts',(0.120755889508211,-0.136245876208876,
3.45784977853496));
#32762=CARTESIAN_POINT('Ctrl Pts',(-0.0480683862207756,-0.175597139874519,
3.44995254400912));
#32763=CARTESIAN_POINT('Ctrl Pts',(-0.173312459951882,-0.0557468937208932,
3.44205530948329));
#32764=CARTESIAN_POINT('Ctrl Pts',(-0.141426385082663,0.114645114551432,
3.43415807495745));
#32765=CARTESIAN_POINT('Ctrl Pts',(0.0186809873893989,0.181096509168673,
3.42626084043161));
#32766=CARTESIAN_POINT('Ctrl Pts',(0.161851630600137,0.0833605094034181,
3.41836360590578));
#32767=CARTESIAN_POINT('Ctrl Pts',(0.158282849894819,-0.0899525667211824,
3.41046637137994));
#32768=CARTESIAN_POINT('Ctrl Pts',(0.0112102066414966,-0.181712014270169,
3.40256913685411));
#32769=CARTESIAN_POINT('Ctrl Pts',(-0.146025938000753,-0.108726033140384,
3.39467190232827));
#32770=CARTESIAN_POINT('Ctrl Pts',(-0.170870694865204,0.0628341506312357,
3.38677466780244));
#32771=CARTESIAN_POINT('Ctrl Pts',(-0.0407990805348497,0.177427055099143,
3.3788774332766));
#32772=CARTESIAN_POINT('Ctrl Pts',(0.126262173896246,0.131159400329288,
3.37098019875077));
#32773=CARTESIAN_POINT('Ctrl Pts',(0.178850447353964,-0.0340212041663437,
3.36308296422493));
#32774=CARTESIAN_POINT('Ctrl Pts',(0.0692876725278909,-0.168357189593675,
3.3551857296991));
#32775=CARTESIAN_POINT('Ctrl Pts',(-0.103093333396635,-0.150055621224551,
3.34728849517326));
#32776=CARTESIAN_POINT('Ctrl Pts',(-0.18200690701094,0.00429076359651101,
3.33939126064742));
#32777=CARTESIAN_POINT('Ctrl Pts',(-0.0959076936642258,0.154747016604558,
3.33149402612159));
#32778=CARTESIAN_POINT('Ctrl Pts',(0.0771442407770374,0.164905096849345,
3.32359679159575));
#32779=CARTESIAN_POINT('Ctrl Pts',(0.180254949482897,0.0255553915814562,
3.31569955706992));
#32780=CARTESIAN_POINT('Ctrl Pts',(0.119941247180243,-0.13696357938087,
3.30780232254408));
#32781=CARTESIAN_POINT('Ctrl Pts',(-0.0491146989958762,-0.175307362065916,
3.29990508801825));
#32782=CARTESIAN_POINT('Ctrl Pts',(-0.173641822089509,-0.0547123612486432,
3.29200785349241));
#32783=CARTESIAN_POINT('Ctrl Pts',(-0.14074018895294,0.115486467023018,
3.28411061896658));
#32784=CARTESIAN_POINT('Ctrl Pts',(0.0197606171930289,0.18098188544746,
3.27621338444074));
#32785=CARTESIAN_POINT('Ctrl Pts',(0.162345869645737,0.0823938314495476,
3.26831614991491));
#32786=CARTESIAN_POINT('Ctrl Pts',(0.157743606844976,-0.0908948807772195,
3.26041891538907));
#32787=CARTESIAN_POINT('Ctrl Pts',(0.0101263748965706,-0.181775634735301,
3.25252168086324));
#32788=CARTESIAN_POINT('Ctrl Pts',(-0.146671724805377,-0.107853279943556,
3.2446244463374));
#32789=CARTESIAN_POINT('Ctrl Pts',(-0.170492947552259,0.0638520139612676,
3.23672721181156));
#32790=CARTESIAN_POINT('Ctrl Pts',(-0.0397402758525677,0.177667203859151,
3.22882997728572));
#32791=CARTESIAN_POINT('Ctrl Pts',(0.127042092635782,0.130404108641901,
3.22093274275989));
#32792=CARTESIAN_POINT('Ctrl Pts',(0.178644383007786,-0.0350871667669908,
3.21303550823405));
#32793=CARTESIAN_POINT('Ctrl Pts',(0.0682824490586963,-0.1687673902225,
3.20513827370822));
#32794=CARTESIAN_POINT('Ctrl Pts',(-0.103986350980073,-0.149438159992073,
3.19724103918238));
#32795=CARTESIAN_POINT('Ctrl Pts',(-0.181978082840693,0.00537607827262928,
3.18934380465655));
#32796=CARTESIAN_POINT('Ctrl Pts',(-0.0949831605760139,0.155316206684809,
3.18144657013072));
#32797=CARTESIAN_POINT('Ctrl Pts',(0.0781262740357409,0.164442117954189,
3.17354933560488));
#32798=CARTESIAN_POINT('Ctrl Pts',(0.180404142828019,0.0244799939226929,
3.16565210107904));
#32799=CARTESIAN_POINT('Ctrl Pts',(0.119122337560023,-0.137676408822293,
3.15775486655321));
#32800=CARTESIAN_POINT('Ctrl Pts',(-0.0501592641604809,-0.175011351262844,
3.14985763202737));
#32801=CARTESIAN_POINT('Ctrl Pts',(-0.173965009458927,-0.0536758822556528,
3.14196039750153));
#32802=CARTESIAN_POINT('Ctrl Pts',(-0.140048987402398,0.116323712026096,
3.1340631629757));
#32803=CARTESIAN_POINT('Ctrl Pts',(0.0208395441149821,0.180860825645154,
3.12616592844986));
#32804=CARTESIAN_POINT('Ctrl Pts',(0.162834335224968,0.0814242232005321,
3.11826869392403));
#32805=CARTESIAN_POINT('Ctrl Pts',(0.157198753896076,-0.0918339622660831,
3.1103714593982));
#32806=CARTESIAN_POINT('Ctrl Pts',(0.00904218304404205,-0.181832790711041,
3.10247422487235));
#32807=CARTESIAN_POINT('Ctrl Pts',(-0.147312295507299,-0.106976691126326,
3.09457699034652));
#32808=CARTESIAN_POINT('Ctrl Pts',(-0.170109136963721,0.0648676065029794,
3.08667975582068));
#32809=CARTESIAN_POINT('Ctrl Pts',(-0.0386800578824722,0.177901034213339,
3.07878252129485));
#32810=CARTESIAN_POINT('Ctrl Pts',(0.127817493356429,0.129644179368171,
3.07088528676902));
#32811=CARTESIAN_POINT('Ctrl Pts',(0.178431965499368,-0.0361518815554529,
3.06298805224317));
#32812=CARTESIAN_POINT('Ctrl Pts',(0.0672747972491473,-0.169171588947593,
3.05509081771735));
#32813=CARTESIAN_POINT('Ctrl Pts',(-0.104875670478854,-0.148815384263785,
3.0471935831915));
#32814=CARTESIAN_POINT('Ctrl Pts',(-0.181942786951853,0.00646120175817659,
3.03929634866568));
#32815=CARTESIAN_POINT('Ctrl Pts',(-0.0940552495850459,0.15587987322763,
3.03139911413983));
#32816=CARTESIAN_POINT('Ctrl Pts',(0.0791055288760802,0.163973290975094,
3.02350187961401));
#32817=CARTESIAN_POINT('Ctrl Pts',(0.180546920428939,0.0234037256776295,
3.01560464508816));
#32818=CARTESIAN_POINT('Ctrl Pts',(0.118299191571216,-0.138384342053441,
3.00770741056233));
#32819=CARTESIAN_POINT('Ctrl Pts',(-0.0512020455023775,-0.174709116500372,
2.99981017603649));
#32820=CARTESIAN_POINT('Ctrl Pts',(-0.174282010080185,-0.0526374943778417,
2.99191294151066));
#32821=CARTESIAN_POINT('Ctrl Pts',(-0.139352805265142,0.117156820188587,
2.98401570698483));
#32822=CARTESIAN_POINT('Ctrl Pts',(0.0219177299165732,0.180733333857582,
2.97611847245899));
#32823=CARTESIAN_POINT('Ctrl Pts',(0.163317009898163,0.0804517192475515,
2.96822123793315));
#32824=CARTESIAN_POINT('Ctrl Pts',(0.156648310460303,-0.0927697778475837,
2.96032400340732));
#32825=CARTESIAN_POINT('Ctrl Pts',(0.00795766962277319,-0.181883480135435,
2.95242676888148));
#32826=CARTESIAN_POINT('Ctrl Pts',(-0.147947627316214,-0.106096297878073,
2.94452953435564));
#32827=CARTESIAN_POINT('Ctrl Pts',(-0.169719276754081,0.0658808921462626,
2.93663229982981));
#32828=CARTESIAN_POINT('Ctrl Pts',(-0.0376184643267171,0.178128537842515,
2.92873506530397));
#32829=CARTESIAN_POINT('Ctrl Pts',(0.128588348481182,0.128879639534425,
2.92083783077814));
#32830=CARTESIAN_POINT('Ctrl Pts',(0.178213202383553,-0.0372153106656781,
2.9129405962523));
#32831=CARTESIAN_POINT('Ctrl Pts',(0.0662647529343645,-0.169569771398652,
2.90504336172647));
#32832=CARTESIAN_POINT('Ctrl Pts',(-0.105761260266122,-0.148187316178505,
2.89714612720063));
#32833=CARTESIAN_POINT('Ctrl Pts',(-0.181901020599063,0.00754609544484455,
2.8892488926748));
#32834=CARTESIAN_POINT('Ctrl Pts',(-0.0931239936920636,0.15643799622185,
2.88135165814895));
#32835=CARTESIAN_POINT('Ctrl Pts',(0.080081970475175,0.163498632518342,
2.87345442362313));
#32836=CARTESIAN_POINT('Ctrl Pts',(0.180683277203119,0.0223266252501708,
2.86555718909729));
#32837=CARTESIAN_POINT('Ctrl Pts',(0.11747183849698,-0.139087354145018,
2.85765995457145));
#32838=CARTESIAN_POINT('Ctrl Pts',(-0.0522430059551858,-0.174400668051551,
2.84976272004562));
#32839=CARTESIAN_POINT('Ctrl Pts',(-0.174592812644639,-0.0515972354582594,
2.84186548551978));
#32840=CARTESIAN_POINT('Ctrl Pts',(-0.138651667367148,0.117985763642445,
2.83396825099395));
#32841=CARTESIAN_POINT('Ctrl Pts',(0.0229951363840201,0.180599411232496,
2.82607101646811));
#32842=CARTESIAN_POINT('Ctrl Pts',(0.163793876249876,0.0794763606914083,
2.81817378194228));
#32843=CARTESIAN_POINT('Ctrl Pts',(0.1560922965942,-0.0937023067775016,
2.81027654741644));
#32844=CARTESIAN_POINT('Ctrl Pts',(0.00687287227597422,-0.181927677084725,
2.8023793128906));
#32845=CARTESIAN_POINT('Ctrl Pts',(-0.148577695856893,-0.105212177919503,
2.79448207836477));
#32846=CARTESIAN_POINT('Ctrl Pts',(-0.169323384214447,0.0668919241546485,
2.78658484383893));
#32847=CARTESIAN_POINT('Ctrl Pts',(-0.0365555263461618,0.178349534836247,
2.7786876093131));
#32848=CARTESIAN_POINT('Ctrl Pts',(0.129354617910885,0.128110846926664,
2.77079037478726));
#32849=CARTESIAN_POINT('Ctrl Pts',(0.177988125847537,-0.0382780523762908,
2.76289314026143));
#32850=CARTESIAN_POINT('Ctrl Pts',(0.0652523050728403,-0.169960699505811,
2.75499590573559));
#32851=CARTESIAN_POINT('Ctrl Pts',(-0.106642998487829,-0.147556332986489,
2.74709867120975));
#32852=CARTESIAN_POINT('Ctrl Pts',(-0.181852959134814,0.00863525184135577,
2.73920143668392));
#32853=CARTESIAN_POINT('Ctrl Pts',(-0.0921890914137533,0.156981837366664,
2.73130420215808));
#32854=CARTESIAN_POINT('Ctrl Pts',(0.081054919689294,0.163034936656946,
2.72340696763225));
#32855=CARTESIAN_POINT('Ctrl Pts',(0.180814453969382,0.0212164304176998,
2.71550973310641));
#32856=CARTESIAN_POINT('Ctrl Pts',(0.116637857196403,-0.139723086682139,
2.70761249858058));
#32857=CARTESIAN_POINT('Ctrl Pts',(-0.0532768903028442,-0.174207676028794,
2.69971526405474));
#32858=CARTESIAN_POINT('Ctrl Pts',(-0.17491212592378,-0.0503049553127666,
2.69181802952891));
#32859=CARTESIAN_POINT('Ctrl Pts',(-0.150223756874352,0.0620211357769783,
2.68655320651168));
#32860=CARTESIAN_POINT('Ctrl Pts',(-0.116913659442528,0.100696009035893,
2.68392079500307));
#32861=CARTESIAN_POINT('Ctrl Pts',(-0.0374537582415199,-0.140096572423086,
3.60535973499898));
#32862=CARTESIAN_POINT('Ctrl Pts',(-0.0837975063399586,-0.127706922146397,
3.60272732349037));
#32863=CARTESIAN_POINT('Ctrl Pts',(-0.162448861737804,-0.0535654059838928,
3.59746250047314));
#32864=CARTESIAN_POINT('Ctrl Pts',(-0.133618139567134,0.107050244683975,
3.5895652659473));
#32865=CARTESIAN_POINT('Ctrl Pts',(0.0165728676468313,0.170252964298069,
3.58166803142147));
#32866=CARTESIAN_POINT('Ctrl Pts',(0.151627908924514,0.0792766640535213,
3.57377079689563));
#32867=CARTESIAN_POINT('Ctrl Pts',(0.149269785166362,-0.0836653848533289,
3.5658735623698));
#32868=CARTESIAN_POINT('Ctrl Pts',(0.0115496459057422,-0.170706646687446,
3.55797632784397));
#32869=CARTESIAN_POINT('Ctrl Pts',(-0.136626328141362,-0.103004841170506,
3.55007909331813));
#32870=CARTESIAN_POINT('Ctrl Pts',(-0.160940885452871,0.0580969370885353,
3.54218185879229));
#32871=CARTESIAN_POINT('Ctrl Pts',(-0.0393375644751653,0.166519695593587,
3.53428462426645));
#32872=CARTESIAN_POINT('Ctrl Pts',(0.117928179856326,0.123974275440694,
3.52638738974062));
#32873=CARTESIAN_POINT('Ctrl Pts',(0.168277910483947,-0.0309716427010613,
3.51849015521478));
#32874=CARTESIAN_POINT('Ctrl Pts',(0.0660613796785464,-0.157836831705444,
3.51059292068895));
#32875=CARTESIAN_POINT('Ctrl Pts',(-0.0960480270061105,-0.141603015411306,
3.50269568616311));
#32876=CARTESIAN_POINT('Ctrl Pts',(-0.171077640137963,0.00301248927320663,
3.49479845163728));
#32877=CARTESIAN_POINT('Ctrl Pts',(-0.0910031773769663,0.144896652245428,
3.48690121711144));
#32878=CARTESIAN_POINT('Ctrl Pts',(0.0715773858794485,0.155413338959437,
3.47900398258561));
#32879=CARTESIAN_POINT('Ctrl Pts',(0.169263819083558,0.0250277102377205,
3.47110674805977));
#32880=CARTESIAN_POINT('Ctrl Pts',(0.113490710154562,-0.128048754471099,
3.46320951353393));
#32881=CARTESIAN_POINT('Ctrl Pts',(-0.0451763910679377,-0.165032481534694,
3.4553122790081));
#32882=CARTESIAN_POINT('Ctrl Pts',(-0.162885257511484,-0.0523929274428053,
3.44741504448226));
#32883=CARTESIAN_POINT('Ctrl Pts',(-0.132917582264447,0.107747584976454,
3.43951780995643));
#32884=CARTESIAN_POINT('Ctrl Pts',(0.0175570610580211,0.17020098577194,
3.43162057543059));
#32885=CARTESIAN_POINT('Ctrl Pts',(0.152113959586497,0.0783451925166497,
3.42372334090476));
#32886=CARTESIAN_POINT('Ctrl Pts',(0.148759891654226,-0.0845406440960262,
3.41582610637892));
#32887=CARTESIAN_POINT('Ctrl Pts',(0.0105357537251741,-0.170779459512285,
3.40792887185309));
#32888=CARTESIAN_POINT('Ctrl Pts',(-0.137240406842142,-0.102184620258639,
3.40003163732725));
#32889=CARTESIAN_POINT('Ctrl Pts',(-0.160590399224686,0.059053785336183,
3.39213440280142));
#32890=CARTESIAN_POINT('Ctrl Pts',(-0.0383444372147038,0.166752301406097,
3.38423716827558));
#32891=CARTESIAN_POINT('Ctrl Pts',(0.118665713444722,0.123268302253741,
3.37633993374974));
#32892=CARTESIAN_POINT('Ctrl Pts',(0.168090056429774,-0.0319743462358346,
3.36844269922391));
#32893=CARTESIAN_POINT('Ctrl Pts',(0.065119036364785,-0.158228116942597,
3.36054546469807));
#32894=CARTESIAN_POINT('Ctrl Pts',(-0.0968908072892766,-0.141027647469737,
3.35264823017224));
#32895=CARTESIAN_POINT('Ctrl Pts',(-0.171056610272434,0.00403261331316083,
3.3447509956464));
#32896=CARTESIAN_POINT('Ctrl Pts',(-0.090137485695877,0.145436788882724,
3.33685376112057));
#32897=CARTESIAN_POINT('Ctrl Pts',(0.0725029206093111,0.154983716535553,
3.32895652659473));
#32898=CARTESIAN_POINT('Ctrl Pts',(0.16941005783654,0.0240178723428656,
3.3210592920689));
#32899=CARTESIAN_POINT('Ctrl Pts',(0.112725080116148,-0.128723277618595,
3.31316205754306));
#32900=CARTESIAN_POINT('Ctrl Pts',(-0.0461597532904643,-0.164760137971002,
3.30526482301723));
#32901=CARTESIAN_POINT('Ctrl Pts',(-0.163194803845412,-0.0514206367708408,
3.29736758849139));
#32902=CARTESIAN_POINT('Ctrl Pts',(-0.132272670563786,0.108538318164536,
3.28947035396555));
#32903=CARTESIAN_POINT('Ctrl Pts',(0.0185717358172978,0.17009325829319,
3.28157311943971));
#32904=CARTESIAN_POINT('Ctrl Pts',(0.152578463144044,0.0774366739514488,
3.27367588491388));
#32905=CARTESIAN_POINT('Ctrl Pts',(0.148253091721553,-0.0854262645973846,
3.26577865038804));
#32906=CARTESIAN_POINT('Ctrl Pts',(0.00951712983096357,-0.170839252304153,
3.25788141586221));
#32907=CARTESIAN_POINT('Ctrl Pts',(-0.137847340411707,-0.101364375544273,
3.24998418133637));
#32908=CARTESIAN_POINT('Ctrl Pts',(-0.160235378769951,0.060010409751241,
3.24208694681054));
#32909=CARTESIAN_POINT('Ctrl Pts',(-0.0373493346503772,0.166978001812321,
3.2341897122847));
#32910=CARTESIAN_POINT('Ctrl Pts',(0.119398709011011,0.122558452073145,
3.22629247775887));
#32911=CARTESIAN_POINT('Ctrl Pts',(0.16789638977649,-0.0329761760682205,
3.21839524323303));
#32912=CARTESIAN_POINT('Ctrl Pts',(0.0641742913436723,-0.158613638185999,
3.2104980087072));
#32913=CARTESIAN_POINT('Ctrl Pts',(-0.0977300972000018,-0.14044733528743,
3.20260077418136));
#32914=CARTESIAN_POINT('Ctrl Pts',(-0.17102952028482,0.00505263091922082,
3.19470353965552));
#32915=CARTESIAN_POINT('Ctrl Pts',(-0.0892685763849535,0.145971734107207,
3.18680630512969));
#32916=CARTESIAN_POINT('Ctrl Pts',(0.0734258706399851,0.15454859238706,
3.17890907060385));
#32917=CARTESIAN_POINT('Ctrl Pts',(0.169550275086044,0.0230071751049201,
3.17101183607802));
#32918=CARTESIAN_POINT('Ctrl Pts',(0.11195543952363,-0.129393220259535,
3.16311460155218));
#32919=CARTESIAN_POINT('Ctrl Pts',(-0.0471414730460515,-0.164481936415857,
3.15521736702635));
#32920=CARTESIAN_POINT('Ctrl Pts',(-0.163498546911009,-0.0504465166889647,
3.14732013250051));
#32921=CARTESIAN_POINT('Ctrl Pts',(-0.131623054589357,0.109325191006596,
3.13942289797468));
#32922=CARTESIAN_POINT('Ctrl Pts',(0.0195857499831994,0.169979481954902,
3.13152566344884));
#32923=CARTESIAN_POINT('Ctrl Pts',(0.153037540591104,0.0765254013899147,
3.123628428923));
#32924=CARTESIAN_POINT('Ctrl Pts',(0.147741019404812,-0.0863088470163307,
3.11573119439717));
#32925=CARTESIAN_POINT('Ctrl Pts',(0.00849816749472986,-0.170892969537348,
3.10783395987133));
#32926=CARTESIAN_POINT('Ctrl Pts',(-0.138449371701125,-0.100540525976471,
3.09993672534551));
#32927=CARTESIAN_POINT('Ctrl Pts',(-0.159874659831641,0.0609648999981013,
3.09203949081965));
#32928=CARTESIAN_POINT('Ctrl Pts',(-0.0363529038275426,0.167197763954447,
3.08414225629384));
#32929=CARTESIAN_POINT('Ctrl Pts',(0.120127458381323,0.121844243322797,
3.07624502176798));
#32930=CARTESIAN_POINT('Ctrl Pts',(0.167696752193779,-0.0339768331620215,
3.06834778724216));
#32931=CARTESIAN_POINT('Ctrl Pts',(0.0632272640813166,-0.158993518625298,
3.06045055271632));
#32932=CARTESIAN_POINT('Ctrl Pts',(-0.0985659115183093,-0.139862028351609,
3.05255331819049));
#32933=CARTESIAN_POINT('Ctrl Pts',(-0.170996347944273,0.0060724688375345,
3.04465608366465));
#32934=CARTESIAN_POINT('Ctrl Pts',(-0.0883964924000305,0.146501488113373,
3.03675884913881));
#32935=CARTESIAN_POINT('Ctrl Pts',(0.0743462094135637,0.154107971999816,
3.02886161461298));
#32936=CARTESIAN_POINT('Ctrl Pts',(0.16968446258935,0.0219956596587875,
3.02096438008714));
#32937=CARTESIAN_POINT('Ctrl Pts',(0.111181817440176,-0.130058561266688,
3.01306714556131));
#32938=CARTESIAN_POINT('Ctrl Pts',(-0.048121516301165,-0.16419788536074,
3.00516991103547));
#32939=CARTESIAN_POINT('Ctrl Pts',(-0.163796475449092,-0.0494706025687624,
2.99727267650963));
#32940=CARTESIAN_POINT('Ctrl Pts',(-0.13096875768114,0.110108175897699,
2.9893754419838));
#32941=CARTESIAN_POINT('Ctrl Pts',(0.020599067617639,0.169859660606483,
2.98147820745796));
#32942=CARTESIAN_POINT('Ctrl Pts',(0.153491175537256,0.0756114073420768,
2.97358097293213));
#32943=CARTESIAN_POINT('Ctrl Pts',(0.147223692948271,-0.0871883600185597,
2.96568373840629));
#32944=CARTESIAN_POINT('Ctrl Pts',(0.00747890293667656,-0.17094060927397,
2.95778650388045));
#32945=CARTESIAN_POINT('Ctrl Pts',(-0.139046479291249,-0.0997131008681262,
2.94988926935462));
#32946=CARTESIAN_POINT('Ctrl Pts',(-0.159508255242737,0.0619172221391909,
2.94199203482878));
#32947=CARTESIAN_POINT('Ctrl Pts',(-0.0353551801800353,0.167411580013796,
2.93409480030295));
#32948=CARTESIAN_POINT('Ctrl Pts',(0.120851935637802,0.121125701403006,
2.92619756577711));
#32949=CARTESIAN_POINT('Ctrl Pts',(0.167491150781951,-0.0349762819293654,
2.91830033125128));
#32950=CARTESIAN_POINT('Ctrl Pts',(0.0622779882568489,-0.159367744754771,
2.91040309672545));
#32951=CARTESIAN_POINT('Ctrl Pts',(-0.0993982205201476,-0.139271747469127,
2.9025058621996));
#32952=CARTESIAN_POINT('Ctrl Pts',(-0.170957094429947,0.0070920907826306,
2.89460862767378));
#32953=CARTESIAN_POINT('Ctrl Pts',(-0.0875212647563887,0.147026032094007,
2.88671139314793));
#32954=CARTESIAN_POINT('Ctrl Pts',(0.0752639042022573,0.153661870981,2.8788141586221));
#32955=CARTESIAN_POINT('Ctrl Pts',(0.169812615569706,0.0209833620978328,
2.87091692409627));
#32956=CARTESIAN_POINT('Ctrl Pts',(0.110404241387148,-0.130719277210608,
2.86301968957043));
#32957=CARTESIAN_POINT('Ctrl Pts',(-0.0490998482194935,-0.163907994460633,
2.8551224550446));
#32958=CARTESIAN_POINT('Ctrl Pts',(-0.164088578831389,-0.0484929299764868,
2.84722522051876));
#32959=CARTESIAN_POINT('Ctrl Pts',(-0.130309803171479,0.110887246646458,
2.83932798599293));
#32960=CARTESIAN_POINT('Ctrl Pts',(0.0216116528059362,0.16973379532663,
2.83143075146709));
#32961=CARTESIAN_POINT('Ctrl Pts',(0.153939351614839,0.0746947304359413,
2.82353351694125));
#32962=CARTESIAN_POINT('Ctrl Pts',(0.146701131201786,-0.0880647841079112,
2.81563628241542));
#32963=CARTESIAN_POINT('Ctrl Pts',(0.00645937153523989,-0.170982147149946,
2.80773904788958));
#32964=CARTESIAN_POINT('Ctrl Pts',(-0.139638640273367,-0.0988821732639446,
2.79984181336375));
#32965=CARTESIAN_POINT('Ctrl Pts',(-0.15913618125404,0.0628674262334842,
2.79194457883791));
#32966=CARTESIAN_POINT('Ctrl Pts',(-0.0343561929939461,0.167619280904103,
2.78404734431207));
#32967=CARTESIAN_POINT('Ctrl Pts',(0.121572103093823,0.120403162573872,
2.77615010978624));
#32968=CARTESIAN_POINT('Ctrl Pts',(0.167279615791685,-0.0359750846539325,
2.7682528752604));
#32969=CARTESIAN_POINT('Ctrl Pts',(0.0613264534930637,-0.159735152992013,
2.76035564073457));
#32970=CARTESIAN_POINT('Ctrl Pts',(-0.100226909682718,-0.138678726864922,
2.75245840620873));
#32971=CARTESIAN_POINT('Ctrl Pts',(-0.170911924544395,0.00811571897511738,
2.74456117168289));
#32972=CARTESIAN_POINT('Ctrl Pts',(-0.0866426101092102,0.147537153481027,
2.73666393715706));
#32973=CARTESIAN_POINT('Ctrl Pts',(0.0761783167224614,0.153226073001953,
2.72876670263122));
#32974=CARTESIAN_POINT('Ctrl Pts',(0.169935900193086,0.0199399612296831,
2.72086946810539));
#32975=CARTESIAN_POINT('Ctrl Pts',(0.109620435889599,-0.131316761419452,
2.71297223357956));
#32976=CARTESIAN_POINT('Ctrl Pts',(-0.0500715297607526,-0.163726613645121,
2.70507499905371));
#32977=CARTESIAN_POINT('Ctrl Pts',(-0.164388680888184,-0.0472783988092873,
2.69717776452789));
#32978=CARTESIAN_POINT('Ctrl Pts',(-0.141185667375647,0.0582896848558531,
2.69191294151066));
#32979=CARTESIAN_POINT('Ctrl Pts',(-0.1098796447191,0.0946377159884756,
2.68928053000205));
#32980=CARTESIAN_POINT('Ctrl Pts',(-0.035056132297315,-0.13112820202432,
3.61071946999795));
#32981=CARTESIAN_POINT('Ctrl Pts',(-0.0784331561467214,-0.119531683020372,
3.60808705848934));
#32982=CARTESIAN_POINT('Ctrl Pts',(-0.152049595447957,-0.0501363827528818,
3.60282223547212));
#32983=CARTESIAN_POINT('Ctrl Pts',(-0.125064490131564,0.100197355787414,
3.59492500094628));
#32984=CARTESIAN_POINT('Ctrl Pts',(0.015511945077094,0.15935411346322,3.58702776642045));
#32985=CARTESIAN_POINT('Ctrl Pts',(0.141921352750402,0.074201718429132,
3.57913053189461));
#32986=CARTESIAN_POINT('Ctrl Pts',(0.139714185771159,-0.078309492500346,
3.57123329736877));
#32987=CARTESIAN_POINT('Ctrl Pts',(0.0108102880423358,-0.159778753088445,
3.56333606284294));
#32988=CARTESIAN_POINT('Ctrl Pts',(-0.127880107617888,-0.0964109213300309,
3.5554388283171));
#32989=CARTESIAN_POINT('Ctrl Pts',(-0.150638153215513,0.0543778250372407,
3.54754159379127));
#32990=CARTESIAN_POINT('Ctrl Pts',(-0.0368193454873861,0.155859832308261,
3.53964435926543));
#32991=CARTESIAN_POINT('Ctrl Pts',(0.110378933082395,0.116037984046548,
3.5317471247396));
#32992=CARTESIAN_POINT('Ctrl Pts',(0.157505493964057,-0.0289889734694223,
3.52384989021376));
#32993=CARTESIAN_POINT('Ctrl Pts',(0.0618324188141689,-0.147732807425485,
3.51595265568793));
#32994=CARTESIAN_POINT('Ctrl Pts',(-0.089899452009857,-0.132538209115007,
3.50805542116209));
#32995=CARTESIAN_POINT('Ctrl Pts',(-0.160125997159357,0.00281964287334723,
3.50015818663625));
#32996=CARTESIAN_POINT('Ctrl Pts',(-0.0851775516099315,0.135621001710926,
3.49226095211042));
#32997=CARTESIAN_POINT('Ctrl Pts',(0.0669953144008998,0.145464456095352,
3.48436371758458));
#32998=CARTESIAN_POINT('Ctrl Pts',(0.15842828900316,0.0234255455897019,
3.47646648305875));
#32999=CARTESIAN_POINT('Ctrl Pts',(0.106225530800914,-0.119851632733321,
3.46856924853291));
#33000=CARTESIAN_POINT('Ctrl Pts',(-0.0422843959151,-0.154467823194868,
3.46067201400708));
#33001=CARTESIAN_POINT('Ctrl Pts',(-0.152458055071087,-0.0490389611647173,
3.45277477948124));
#33002=CARTESIAN_POINT('Ctrl Pts',(-0.124408779446231,0.100850055401476,
3.44487754495541));
#33003=CARTESIAN_POINT('Ctrl Pts',(0.0164331347266433,0.159305462375208,
3.43698031042957));
#33004=CARTESIAN_POINT('Ctrl Pts',(0.142376288572858,0.0733298756298809,
3.42908307590374));
#33005=CARTESIAN_POINT('Ctrl Pts',(0.139236933413632,-0.0791287214708696,
3.4211858413779));
#33006=CARTESIAN_POINT('Ctrl Pts',(0.00986130080885162,-0.159846904754402,
3.41328860685207));
#33007=CARTESIAN_POINT('Ctrl Pts',(-0.128454875683531,-0.0956432073768941,
3.40539137232623));
#33008=CARTESIAN_POINT('Ctrl Pts',(-0.150310103584168,0.0552734200411303,
3.3974941378004));
#33009=CARTESIAN_POINT('Ctrl Pts',(-0.0358897938945578,0.15607754771305,
3.38959690327456));
#33010=CARTESIAN_POINT('Ctrl Pts',(0.111069252993198,0.115377204178194,
3.38169966874872));
#33011=CARTESIAN_POINT('Ctrl Pts',(0.157329665505583,-0.0299274883053255,
3.37380243422289));
#33012=CARTESIAN_POINT('Ctrl Pts',(0.060950400201679,-0.14809904429152,
3.36590519969705));
#33013=CARTESIAN_POINT('Ctrl Pts',(-0.090688281181918,-0.131999673714922,
3.35800796517121));
#33014=CARTESIAN_POINT('Ctrl Pts',(-0.160106313533927,0.00377446302981049,
3.35011073064538));
#33015=CARTESIAN_POINT('Ctrl Pts',(-0.0843672777275282,0.13612656116089,
3.34221349611954));
#33016=CARTESIAN_POINT('Ctrl Pts',(0.0678616004415848,0.145062336221761,
3.33431626159371));
#33017=CARTESIAN_POINT('Ctrl Pts',(0.158565166190183,0.0224803531042752,
3.32641902706787));
#33018=CARTESIAN_POINT('Ctrl Pts',(0.105508913052052,-0.12048297585632,
3.31852179254204));
#33019=CARTESIAN_POINT('Ctrl Pts',(-0.0432048075850524,-0.154212913876088,
3.3106245580162));
#33020=CARTESIAN_POINT('Ctrl Pts',(-0.152747785601314,-0.0481289122930385,
3.30272732349037));
#33021=CARTESIAN_POINT('Ctrl Pts',(-0.123805152174632,0.101590169306055,
3.29483008896453));
#33022=CARTESIAN_POINT('Ctrl Pts',(0.0173828544415669,0.159204631138919,
3.28693285443869));
#33023=CARTESIAN_POINT('Ctrl Pts',(0.142811056642351,0.0724795164533502,
3.27903561991286));
#33024=CARTESIAN_POINT('Ctrl Pts',(0.13876257659813,-0.0799576484175498,
3.27113838538702));
#33025=CARTESIAN_POINT('Ctrl Pts',(0.00890788476535658,-0.159902869873006,
3.26324115086119));
#33026=CARTESIAN_POINT('Ctrl Pts',(-0.129022956018037,-0.0948754711449903,
3.25534391633535));
#33027=CARTESIAN_POINT('Ctrl Pts',(-0.149977809987643,0.0561688055412144,
3.24744668180951));
#33028=CARTESIAN_POINT('Ctrl Pts',(-0.0349583934481866,0.156288799765492,
3.23954944728368));
#33029=CARTESIAN_POINT('Ctrl Pts',(0.111755325386239,0.11471279550439,3.23165221275784));
#33030=CARTESIAN_POINT('Ctrl Pts',(0.157148396545194,-0.0308651853694504,
3.22375497823201));
#33031=CARTESIAN_POINT('Ctrl Pts',(0.0600661336286481,-0.148459886149497,
3.21585774370617));
#33032=CARTESIAN_POINT('Ctrl Pts',(-0.0914738434199304,-0.131456510582787,
3.20796050918034));
#33033=CARTESIAN_POINT('Ctrl Pts',(-0.160080957728948,0.00472918356581254,
3.2000632746545));
#33034=CARTESIAN_POINT('Ctrl Pts',(-0.0835539921938928,0.136627261529605,
3.19216604012867));
#33035=CARTESIAN_POINT('Ctrl Pts',(0.0687254672442293,0.144655066819931,
3.18426880560283));
#33036=CARTESIAN_POINT('Ctrl Pts',(0.158696407344068,0.0215343562871474,
3.176371571077));
#33037=CARTESIAN_POINT('Ctrl Pts',(0.104788541487236,-0.121110031696776,
3.16847433655116));
#33038=CARTESIAN_POINT('Ctrl Pts',(-0.0441236819316221,-0.15395252156887,
3.16057710202533));
#33039=CARTESIAN_POINT('Ctrl Pts',(-0.153032084363091,-0.0472171511222767,
3.15267986749949));
#33040=CARTESIAN_POINT('Ctrl Pts',(-0.123197121776316,0.102326669987095,
3.14478263297366));
#33041=CARTESIAN_POINT('Ctrl Pts',(0.0183319558514166,0.159098138264651,
3.13688539844782));
#33042=CARTESIAN_POINT('Ctrl Pts',(0.143240745957241,0.0716265795792973,
3.12898816392198));
#33043=CARTESIAN_POINT('Ctrl Pts',(0.138283284913549,-0.0807837317665782,
3.12109092939615));
#33044=CARTESIAN_POINT('Ctrl Pts',(0.00795415194541781,-0.159953148363655,
3.11319369487031));
#33045=CARTESIAN_POINT('Ctrl Pts',(-0.12958644789495,-0.0941043608266151,
3.10529646034448));
#33046=CARTESIAN_POINT('Ctrl Pts',(-0.149640182699562,0.0570621934932236,
3.09739922581864));
#33047=CARTESIAN_POINT('Ctrl Pts',(-0.0340257497726133,0.156494493695554,
3.08950199129281));
#33048=CARTESIAN_POINT('Ctrl Pts',(0.112437423406217,0.114044307277423,
3.08160475676696));
#33049=CARTESIAN_POINT('Ctrl Pts',(0.156961538888189,-0.0318017847685902,
3.07370752224114));
#33050=CARTESIAN_POINT('Ctrl Pts',(0.0591797309134862,-0.148815448303003,
3.06581028771529));
#33051=CARTESIAN_POINT('Ctrl Pts',(-0.0922561525577649,-0.130908672439433,
3.05791305318946));
#33052=CARTESIAN_POINT('Ctrl Pts',(-0.160049908936692,0.00568373591689232,
3.05001581866362));
#33053=CARTESIAN_POINT('Ctrl Pts',(-0.0827377352150154,0.137123102999116,
3.04211858413779));
#33054=CARTESIAN_POINT('Ctrl Pts',(0.0695868899510474,0.144242653024537,
3.03422134961195));
#33055=CARTESIAN_POINT('Ctrl Pts',(0.15882200474976,0.0205875936399453,
3.02632411508612));
#33056=CARTESIAN_POINT('Ctrl Pts',(0.104064443309136,-0.121732780479934,
3.01842688056028));
#33057=CARTESIAN_POINT('Ctrl Pts',(-0.0450409870999527,-0.153686654221109,
3.01052964603445));
#33058=CARTESIAN_POINT('Ctrl Pts',(-0.153310940817998,-0.0463037107596828,
3.00263241150861));
#33059=CARTESIAN_POINT('Ctrl Pts',(-0.122584710097139,0.103059531606811,
2.99473517698278));
#33060=CARTESIAN_POINT('Ctrl Pts',(0.019280405318705,0.158985987355384,
2.98683794245694));
#33061=CARTESIAN_POINT('Ctrl Pts',(0.143665341176349,0.0707710954366019,
2.97894070793111));
#33062=CARTESIAN_POINT('Ctrl Pts',(0.13779907543624,-0.0816069421895357,
2.97104347340527));
#33063=CARTESIAN_POINT('Ctrl Pts',(0.00700013625057968,-0.159997738412506,
2.96314623887943));
#33064=CARTESIAN_POINT('Ctrl Pts',(-0.130145331266283,-0.0933299038581796,
2.9552490043536));
#33065=CARTESIAN_POINT('Ctrl Pts',(-0.149297233731393,0.0579535521321195,
2.94735176982776));
#33066=CARTESIAN_POINT('Ctrl Pts',(-0.0330918960333533,0.156694622185077,
2.93945453530193));
#33067=CARTESIAN_POINT('Ctrl Pts',(0.113115522794421,0.113371763271587,
2.93155730077609));
#33068=CARTESIAN_POINT('Ctrl Pts',(0.156769099180348,-0.0327372531930529,
2.92366006625026));
#33069=CARTESIAN_POINT('Ctrl Pts',(0.0582912235793329,-0.14916571811089,
2.91576283172442));
#33070=CARTESIAN_POINT('Ctrl Pts',(-0.0930351807741731,-0.130356178759748,
2.90786559719858));
#33071=CARTESIAN_POINT('Ctrl Pts',(-0.160013168260831,0.00663808612041647,
2.89996836267275));
#33072=CARTESIAN_POINT('Ctrl Pts',(-0.0819185358207136,0.137614067966164,
2.89207112814691));
#33073=CARTESIAN_POINT('Ctrl Pts',(0.0704458379293395,0.143825109443657,
2.88417389362108));
#33074=CARTESIAN_POINT('Ctrl Pts',(0.158941953936293,0.0196400989454948,
2.87627665909524));
#33075=CARTESIAN_POINT('Ctrl Pts',(0.103336644277317,-0.122351200276197,
2.86837942456941));
#33076=CARTESIAN_POINT('Ctrl Pts',(-0.0459566904838012,-0.153415320869716,
2.86048219004357));
#33077=CARTESIAN_POINT('Ctrl Pts',(-0.15358434501814,-0.0453886244947142,
2.85258495551773));
#33078=CARTESIAN_POINT('Ctrl Pts',(-0.12196793897581,0.103788729650472,
2.8446877209919));
#33079=CARTESIAN_POINT('Ctrl Pts',(0.0202281692278525,0.158868179420765,
2.83679048646607));
#33080=CARTESIAN_POINT('Ctrl Pts',(0.144084826979801,0.0699131001804741,
2.82889325194023));
#33081=CARTESIAN_POINT('Ctrl Pts',(0.137309965809371,-0.0824272614383206,
2.8209960174144));
#33082=CARTESIAN_POINT('Ctrl Pts',(0.00604587079450571,-0.160036617215166,
2.81309878288855));
#33083=CARTESIAN_POINT('Ctrl Pts',(-0.13069958468984,-0.0925521686083858,
2.80520154836272));
#33084=CARTESIAN_POINT('Ctrl Pts',(-0.148948978293633,0.0588429283123199,
2.79730431383689));
#33085=CARTESIAN_POINT('Ctrl Pts',(-0.0321568596417307,0.156889026971959,
2.78940707931105));
#33086=CARTESIAN_POINT('Ctrl Pts',(0.113789588276761,0.11269547822108,2.78150984478522));
#33087=CARTESIAN_POINT('Ctrl Pts',(0.156571105735832,-0.0336721169315741,
2.77361261025938));
#33088=CARTESIAN_POINT('Ctrl Pts',(0.0574006019132872,-0.149509606478216,
2.76571537573355));
#33089=CARTESIAN_POINT('Ctrl Pts',(-0.0938108208776064,-0.129801120743354,
2.75781814120771));
#33090=CARTESIAN_POINT('Ctrl Pts',(-0.159970889953977,0.00759618610887905,
2.74992090668187));
#33091=CARTESIAN_POINT('Ctrl Pts',(-0.0810961288046671,0.138092469595389,
2.74202367215604));
#33092=CARTESIAN_POINT('Ctrl Pts',(0.0713017137556289,0.143417209346961,
2.7341264376302));
#33093=CARTESIAN_POINT('Ctrl Pts',(0.15905734641679,0.0186634920416663,
2.72622920310437));
#33094=CARTESIAN_POINT('Ctrl Pts',(0.102603014582794,-0.122910436156766,
2.71833196857853));
#33095=CARTESIAN_POINT('Ctrl Pts',(-0.046866169218661,-0.153245551261449,
2.7104347340527));
#33096=CARTESIAN_POINT('Ctrl Pts',(-0.153865235852588,-0.044251842305808,
2.70253749952686));
#33097=CARTESIAN_POINT('Ctrl Pts',(-0.132147577876941,0.0545582339347279,
2.69727267650964));
#33098=CARTESIAN_POINT('Ctrl Pts',(-0.102845629995673,0.0885794229410579,
2.69464026500102));
#33099=CARTESIAN_POINT('Ctrl Pts',(-0.0326585063531101,-0.122159831625555,
3.61607920499693));
#33100=CARTESIAN_POINT('Ctrl Pts',(-0.0730688059534842,-0.111356443894347,
3.61344679348832));
#33101=CARTESIAN_POINT('Ctrl Pts',(-0.14165032915811,-0.0467073595218706,
3.60818197047109));
#33102=CARTESIAN_POINT('Ctrl Pts',(-0.116510840695994,0.0933444668908538,
3.60028473594526));
#33103=CARTESIAN_POINT('Ctrl Pts',(0.0144510225073566,0.148455262628371,
3.59238750141942));
#33104=CARTESIAN_POINT('Ctrl Pts',(0.132214796576289,0.0691267728047427,
3.58449026689359));
#33105=CARTESIAN_POINT('Ctrl Pts',(0.130158586375956,-0.0729536001473631,
3.57659303236775));
#33106=CARTESIAN_POINT('Ctrl Pts',(0.0100709301789295,-0.148850859489444,
3.56869579784192));
#33107=CARTESIAN_POINT('Ctrl Pts',(-0.119133887094416,-0.0898170014895561,
3.56079856331608));
#33108=CARTESIAN_POINT('Ctrl Pts',(-0.140335420978156,0.0506587129859461,
3.55290132879025));
#33109=CARTESIAN_POINT('Ctrl Pts',(-0.0343011264996069,0.145199969022934,
3.54500409426441));
#33110=CARTESIAN_POINT('Ctrl Pts',(0.102829686308464,0.108101692652402,
3.53710685973857));
#33111=CARTESIAN_POINT('Ctrl Pts',(0.146733077444168,-0.0270063042377832,
3.52920962521274));
#33112=CARTESIAN_POINT('Ctrl Pts',(0.0576034579497911,-0.137628783145524,
3.5213123906869));
#33113=CARTESIAN_POINT('Ctrl Pts',(-0.0837508770136032,-0.123473402818708,
3.51341515616107));
#33114=CARTESIAN_POINT('Ctrl Pts',(-0.149174354180752,0.00262679647348802,
3.50551792163523));
#33115=CARTESIAN_POINT('Ctrl Pts',(-0.0793519258428967,0.126345351176423,
3.4976206871094));
#33116=CARTESIAN_POINT('Ctrl Pts',(0.062413242922351,0.135515573231267,
3.48972345258356));
#33117=CARTESIAN_POINT('Ctrl Pts',(0.147592758922763,0.0218233809416831,
3.48182621805773));
#33118=CARTESIAN_POINT('Ctrl Pts',(0.0989603514472664,-0.111654510995544,
3.47392898353189));
#33119=CARTESIAN_POINT('Ctrl Pts',(-0.0393924007622622,-0.143903164855042,
3.46603174900606));
#33120=CARTESIAN_POINT('Ctrl Pts',(-0.14203085263069,-0.0456849948866295,
3.45813451448022));
#33121=CARTESIAN_POINT('Ctrl Pts',(-0.115899976628015,0.0939525258264977,
3.45023727995438));
#33122=CARTESIAN_POINT('Ctrl Pts',(0.0153092083952656,0.148409938978475,
3.44234004542855));
#33123=CARTESIAN_POINT('Ctrl Pts',(0.132638617559218,0.0683145587431124,
3.43444281090271));
#33124=CARTESIAN_POINT('Ctrl Pts',(0.129713975173039,-0.0737167988457132,
3.42654557637688));
#33125=CARTESIAN_POINT('Ctrl Pts',(0.00918684789252914,-0.148914349996519,
3.41864834185104));
#33126=CARTESIAN_POINT('Ctrl Pts',(-0.11966934452492,-0.0891017944951492,
3.4107511073252));
#33127=CARTESIAN_POINT('Ctrl Pts',(-0.140029807943649,0.0514930547460776,
3.40285387279937));
#33128=CARTESIAN_POINT('Ctrl Pts',(-0.0334351505744119,0.145402794020004,
3.39495663827353));
#33129=CARTESIAN_POINT('Ctrl Pts',(0.103472792541674,0.107486106102647,
3.3870594037477));
#33130=CARTESIAN_POINT('Ctrl Pts',(0.146569274581392,-0.0278806303748164,
3.37916216922186));
#33131=CARTESIAN_POINT('Ctrl Pts',(0.0567817640385731,-0.137969971640442,
3.37126493469603));
#33132=CARTESIAN_POINT('Ctrl Pts',(-0.0844857550745595,-0.122971699960107,
3.36336770017019));
#33133=CARTESIAN_POINT('Ctrl Pts',(-0.14915601679542,0.00351631274646034,
3.35547046564435));
#33134=CARTESIAN_POINT('Ctrl Pts',(-0.0785970697591793,0.126816333439056,
3.34757323111852));
#33135=CARTESIAN_POINT('Ctrl Pts',(0.0632202802738586,0.13514095590797,
3.33967599659268));
#33136=CARTESIAN_POINT('Ctrl Pts',(0.147720274543826,0.0209428338656845,
3.33177876206685));
#33137=CARTESIAN_POINT('Ctrl Pts',(0.0982927459879567,-0.112242674094044,
3.32388152754101));
#33138=CARTESIAN_POINT('Ctrl Pts',(-0.0402498618796406,-0.143665689781173,
3.31598429301518));
#33139=CARTESIAN_POINT('Ctrl Pts',(-0.142300767357216,-0.0448371878152361,
3.30808705848934));
#33140=CARTESIAN_POINT('Ctrl Pts',(-0.115337633785478,0.0946420204475735,
3.30018982396351));
#33141=CARTESIAN_POINT('Ctrl Pts',(0.0161939730658361,0.148316003984649,
3.29229258943767));
#33142=CARTESIAN_POINT('Ctrl Pts',(0.133043650140658,0.0675223589552513,
3.28439535491184));
#33143=CARTESIAN_POINT('Ctrl Pts',(0.129272061474707,-0.0744890322377149,
3.276498120386));
#33144=CARTESIAN_POINT('Ctrl Pts',(0.00829863969974947,-0.148966487441859,
3.26860088586017));
#33145=CARTESIAN_POINT('Ctrl Pts',(-0.120198571624367,-0.0883865667457073,
3.26070365133432));
#33146=CARTESIAN_POINT('Ctrl Pts',(-0.139720241205335,0.0523272013311878,
3.2528064168085));
#33147=CARTESIAN_POINT('Ctrl Pts',(-0.032567452245996,0.145599597718663,
3.24490918228265));
#33148=CARTESIAN_POINT('Ctrl Pts',(0.104111941761468,0.106867138935634,
3.23701194775683));
#33149=CARTESIAN_POINT('Ctrl Pts',(0.146400403313899,-0.0287541946706802,
3.22911471323098));
#33150=CARTESIAN_POINT('Ctrl Pts',(0.0559579759136239,-0.138306134112995,
3.22121747870515));
#33151=CARTESIAN_POINT('Ctrl Pts',(-0.085217589639859,-0.122465685878144,
3.21332024417931));
#33152=CARTESIAN_POINT('Ctrl Pts',(-0.149132395173076,0.00440573621240416,
3.20542300965348));
#33153=CARTESIAN_POINT('Ctrl Pts',(-0.077839408002832,0.127282788952003,
3.19752577512764));
#33154=CARTESIAN_POINT('Ctrl Pts',(0.0640250638484733,0.134761541252801,
3.18962854060181));
#33155=CARTESIAN_POINT('Ctrl Pts',(0.147842539602093,0.0200615374693747,
3.18173130607597));
#33156=CARTESIAN_POINT('Ctrl Pts',(0.0976216434508421,-0.112826843134018,
3.17383407155013));
#33157=CARTESIAN_POINT('Ctrl Pts',(-0.0411058908171925,-0.143423106721883,
3.1659368370243));
#33158=CARTESIAN_POINT('Ctrl Pts',(-0.142565621815174,-0.0439877855555886,
3.15803960249846));
#33159=CARTESIAN_POINT('Ctrl Pts',(-0.114771188963274,0.0953281489675947,
3.15014236797263));
#33160=CARTESIAN_POINT('Ctrl Pts',(0.0170781617196339,0.148216794574399,
3.14224513344679));
#33161=CARTESIAN_POINT('Ctrl Pts',(0.133443951323378,0.0667277577686799,
3.13434789892096));
#33162=CARTESIAN_POINT('Ctrl Pts',(0.128825550422286,-0.0752586165168258,
3.12645066439512));
#33163=CARTESIAN_POINT('Ctrl Pts',(0.00741013639610572,-0.149013327189962,
3.11855342986929));
#33164=CARTESIAN_POINT('Ctrl Pts',(-0.120723524088775,-0.0876681956767594,
3.11065619534345));
#33165=CARTESIAN_POINT('Ctrl Pts',(-0.139405705567482,0.0531594869883457,
3.10275896081762));
#33166=CARTESIAN_POINT('Ctrl Pts',(-0.0316985957176838,0.145791223436661,
3.09486172629178));
#33167=CARTESIAN_POINT('Ctrl Pts',(0.104747388431111,0.106244371232049,
3.08696449176594));
#33168=CARTESIAN_POINT('Ctrl Pts',(0.1462263255826,-0.0296267363751589,
3.07906725724011));
#33169=CARTESIAN_POINT('Ctrl Pts',(0.0551321977456556,-0.138637377980708,
3.07117002271428));
#33170=CARTESIAN_POINT('Ctrl Pts',(-0.0859463935972202,-0.121955316527256,
3.06327278818844));
#33171=CARTESIAN_POINT('Ctrl Pts',(-0.149103469929111,0.00529500299625034,
3.0553755536626));
#33172=CARTESIAN_POINT('Ctrl Pts',(-0.0770789780300003,0.127744717884859,
3.04747831913677));
#33173=CARTESIAN_POINT('Ctrl Pts',(0.064827570488531,0.134377334049259,
3.03958108461093));
#33174=CARTESIAN_POINT('Ctrl Pts',(0.147959546910171,0.0191795276211033,
3.0316838500851));
#33175=CARTESIAN_POINT('Ctrl Pts',(0.096947069178096,-0.11340699969318,
3.02378661555926));
#33176=CARTESIAN_POINT('Ctrl Pts',(-0.0419604578987403,-0.143175423081478,
3.01588938103343));
#33177=CARTESIAN_POINT('Ctrl Pts',(-0.142825406186904,-0.0431368189506033,
3.00799214650759));
#33178=CARTESIAN_POINT('Ctrl Pts',(-0.114200662513138,0.0960108873159227,
3.00009491198175));
#33179=CARTESIAN_POINT('Ctrl Pts',(0.0179617430197712,0.148112314104285,
2.99219767745592));
#33180=CARTESIAN_POINT('Ctrl Pts',(0.133839506815442,0.065930783531127,
2.98430044293008));
#33181=CARTESIAN_POINT('Ctrl Pts',(0.128374457924208,-0.0760255243605117,
2.97640320840425));
#33182=CARTESIAN_POINT('Ctrl Pts',(0.00652136956448273,-0.149054867551042,
2.96850597387841));
#33183=CARTESIAN_POINT('Ctrl Pts',(-0.121244183241318,-0.0869467068482327,
2.96060873935258));
#33184=CARTESIAN_POINT('Ctrl Pts',(-0.139086212220049,0.0539898821250478,
2.95271150482674));
#33185=CARTESIAN_POINT('Ctrl Pts',(-0.0308286118866713,0.145977664356358,
2.9448142703009));
#33186=CARTESIAN_POINT('Ctrl Pts',(0.10537910995104,0.105617825140169,2.93691703577507));
#33187=CARTESIAN_POINT('Ctrl Pts',(0.146047047578745,-0.0304982244567401,
2.92901980124923));
#33188=CARTESIAN_POINT('Ctrl Pts',(0.0543044589018171,-0.138963691467009,
2.9211225667234));
#33189=CARTESIAN_POINT('Ctrl Pts',(-0.0866721410281989,-0.121440610050369,
2.91322533219756));
#33190=CARTESIAN_POINT('Ctrl Pts',(-0.149069242091714,0.0061840814582022,
2.90532809767173));
#33191=CARTESIAN_POINT('Ctrl Pts',(-0.0763158068850386,0.128202103838321,
2.89743086314589));
#33192=CARTESIAN_POINT('Ctrl Pts',(0.0656277716564218,0.133988347906315,
2.88953362862006));
#33193=CARTESIAN_POINT('Ctrl Pts',(0.14807129230288,0.0182968357931569,
2.88163639409422));
#33194=CARTESIAN_POINT('Ctrl Pts',(0.0962690471674858,-0.113983123341786,
2.87373915956838));
#33195=CARTESIAN_POINT('Ctrl Pts',(-0.0428135327481091,-0.142922647278798,
2.86584192504255));
#33196=CARTESIAN_POINT('Ctrl Pts',(-0.14308011120489,-0.0422843190129418,
2.85794469051671));
#33197=CARTESIAN_POINT('Ctrl Pts',(-0.113626074780142,0.0966902126544859,
2.85004745599088));
#33198=CARTESIAN_POINT('Ctrl Pts',(0.0188446856497688,0.1480025635149,2.84215022146504));
#33199=CARTESIAN_POINT('Ctrl Pts',(0.134230302344763,0.0651314699250072,
2.8342529869392));
#33200=CARTESIAN_POINT('Ctrl Pts',(0.127918800416957,-0.0767897387687304,
2.82635575241337));
#33201=CARTESIAN_POINT('Ctrl Pts',(0.00563237005377145,-0.149091087280386,
2.81845851788753));
#33202=CARTESIAN_POINT('Ctrl Pts',(-0.121760529106313,-0.0862221639528271,
2.8105612833617));
#33203=CARTESIAN_POINT('Ctrl Pts',(-0.138761775333226,0.0548184303911556,
2.80266404883586));
#33204=CARTESIAN_POINT('Ctrl Pts',(-0.0299575262895149,0.146158773039815,
2.79476681431003));
#33205=CARTESIAN_POINT('Ctrl Pts',(0.106007073459698,0.104987793868287,
2.7868695797842));
#33206=CARTESIAN_POINT('Ctrl Pts',(0.145862595679981,-0.0313691492092156,
2.77897234525835));
#33207=CARTESIAN_POINT('Ctrl Pts',(0.0534747503335104,-0.139284059964419,
2.77107511073252));
#33208=CARTESIAN_POINT('Ctrl Pts',(-0.0873947320724949,-0.120923514621786,
2.76317787620668));
#33209=CARTESIAN_POINT('Ctrl Pts',(-0.149029855363559,0.00707665324264049,
2.75528064168085));
#33210=CARTESIAN_POINT('Ctrl Pts',(-0.0755496475001239,0.128647785709752,
2.74738340715502));
#33211=CARTESIAN_POINT('Ctrl Pts',(0.0664251107887961,0.133608345691969,
2.73948617262918));
#33212=CARTESIAN_POINT('Ctrl Pts',(0.148178792640495,0.0173870228536497,
2.73158893810334));
#33213=CARTESIAN_POINT('Ctrl Pts',(0.0955855932759896,-0.114504110894079,
2.72369170357751));
#33214=CARTESIAN_POINT('Ctrl Pts',(-0.0436608086765693,-0.142764488877777,
2.71579446905167));
#33215=CARTESIAN_POINT('Ctrl Pts',(-0.143341790816993,-0.0412252858023288,
2.70789723452584));
#33216=CARTESIAN_POINT('Ctrl Pts',(-0.123109488378236,0.0508267830136028,
2.70263241150861));
#33217=CARTESIAN_POINT('Ctrl Pts',(-0.0958116152722464,0.0825211298936403,
2.7));
#33218=CARTESIAN_POINT('Ctrl Pts',(-0.126320239448181,8.84447983197572E-5,
3.55565803263806));
#33219=CARTESIAN_POINT('Ctrl Pts',(-0.126416389705588,0.0147241557759941,
3.55473913135546));
#33220=CARTESIAN_POINT('Ctrl Pts',(-0.124064907197002,0.029329993953288,
3.55382023007285));
#33221=CARTESIAN_POINT('Ctrl Pts',(-0.119129449584441,0.0430029699128602,
3.55290132879025));
#33222=CARTESIAN_POINT('Ctrl Pts',(-0.104990656151973,0.0821724649982754,
3.55026891728164));
#33223=CARTESIAN_POINT('Ctrl Pts',(-0.0696458913257897,0.113686217010605,
3.54763650577302));
#33224=CARTESIAN_POINT('Ctrl Pts',(-0.0291183734446862,0.123260046955014,
3.54500409426441));
#33225=CARTESIAN_POINT('Ctrl Pts',(0.011409144436417,0.132833876899423,
3.5423716827558));
#33226=CARTESIAN_POINT('Ctrl Pts',(0.0571194153724406,0.120467784775912,
3.53973927124719));
#33227=CARTESIAN_POINT('Ctrl Pts',(0.0872917826964029,0.0917667392324598,
3.53710685973857));
#33228=CARTESIAN_POINT('Ctrl Pts',(0.117464150020365,0.0630656936890069,
3.53447444822996));
#33229=CARTESIAN_POINT('Ctrl Pts',(0.132098613732267,0.0180296947256118,
3.53184203672135));
#33230=CARTESIAN_POINT('Ctrl Pts',(0.124560909005821,-0.0229253845740426,
3.52920962521274));
#33231=CARTESIAN_POINT('Ctrl Pts',(0.117023204279375,-0.0638804638736969,
3.52657721370413));
#33232=CARTESIAN_POINT('Ctrl Pts',(0.0873133311145834,-0.100754623509611,
3.52394480219552));
#33233=CARTESIAN_POINT('Ctrl Pts',(0.048899338704955,-0.116832473273098,
3.5213123906869));
#33234=CARTESIAN_POINT('Ctrl Pts',(0.0104853462953266,-0.132910323036586,
3.51867997917829));
#33235=CARTESIAN_POINT('Ctrl Pts',(-0.0366327653591382,-0.128191862927647,
3.51604756766968));
#33236=CARTESIAN_POINT('Ctrl Pts',(-0.0710957340475621,-0.104815932991145,
3.51341515616107));
#33237=CARTESIAN_POINT('Ctrl Pts',(-0.104947268304411,-0.0818547336764444,
3.51082944832006));
#33238=CARTESIAN_POINT('Ctrl Pts',(-0.126588725667586,-0.0408922251827605,
3.50824374047906));
#33239=CARTESIAN_POINT('Ctrl Pts',(-0.12665116202208,1.34725138570783E-5,
3.50565803263806));
#33240=CARTESIAN_POINT('Ctrl Pts',(-0.0398513841857247,-0.149064942821851,
3.6));
#33241=CARTESIAN_POINT('Ctrl Pts',(-0.0498814435786606,-0.145400000402268,
3.6));
#33242=CARTESIAN_POINT('Ctrl Pts',(-0.059436150936811,-0.14063603073288,
3.6));
#33243=CARTESIAN_POINT('Ctrl Pts',(-0.0684043669488933,-0.134923276476459,
3.6));
#33244=CARTESIAN_POINT('Ctrl Pts',(-0.0756266237179617,-0.130322698385691,
3.6));
#33245=CARTESIAN_POINT('Ctrl Pts',(-0.0824683814027756,-0.125105404214097,
3.6));
#33246=CARTESIAN_POINT('Ctrl Pts',(-0.0888542192956036,-0.119334036703677,
3.6));
#33247=CARTESIAN_POINT('Ctrl Pts',(-0.091539386939335,-0.116907246428204,
3.6));
#33248=CARTESIAN_POINT('Ctrl Pts',(-0.0941378270474737,-0.114387469535812,
3.6));
#33249=CARTESIAN_POINT('Ctrl Pts',(-0.0966394276056281,-0.111785621852247,
3.6));
#33250=CARTESIAN_POINT('Ctrl Pts',(-0.103848676908048,-0.104287474901247,
3.6));
#33251=CARTESIAN_POINT('Ctrl Pts',(-0.110272002565724,-0.0960958678941195,
3.6));
#33252=CARTESIAN_POINT('Ctrl Pts',(-0.115776223647425,-0.0873309061633839,
3.6));
#33253=CARTESIAN_POINT('Ctrl Pts',(-0.118162872674894,-0.0835303888731155,
3.6));
#33254=CARTESIAN_POINT('Ctrl Pts',(-0.120376124201495,-0.0796218141710604,
3.6));
#33255=CARTESIAN_POINT('Ctrl Pts',(-0.122402049312502,-0.0756142631648066,
3.6));
#33256=CARTESIAN_POINT('Ctrl Pts',(-0.123825086107396,-0.0727993059344893,
3.6));
#33257=CARTESIAN_POINT('Ctrl Pts',(-0.125154691418473,-0.0699368314187636,
3.6));
#33258=CARTESIAN_POINT('Ctrl Pts',(-0.126381872197889,-0.0670411886576404,
3.6));
#33259=CARTESIAN_POINT('Ctrl Pts',(-0.129549149387792,-0.0595677149679855,
3.6));
#33260=CARTESIAN_POINT('Ctrl Pts',(-0.132046086846552,-0.0518539539453467,
3.6));
#33261=CARTESIAN_POINT('Ctrl Pts',(-0.133799060139059,-0.0439576297154888,
3.6));
#33262=CARTESIAN_POINT('Ctrl Pts',(-0.135388531616607,-0.0367978046374413,
3.6));
#33263=CARTESIAN_POINT('Ctrl Pts',(-0.136365840160023,-0.0294873792206846,
3.6));
#33264=CARTESIAN_POINT('Ctrl Pts',(-0.13674259160829,-0.0221011370783161,
3.6));
#33265=CARTESIAN_POINT('Ctrl Pts',(-0.136915659814306,-0.0187081211187088,
3.6));
#33266=CARTESIAN_POINT('Ctrl Pts',(-0.136961265679344,-0.0153067045798101,
3.6));
#33267=CARTESIAN_POINT('Ctrl Pts',(-0.136881936917631,-0.0119112232715221,
3.6));
#33268=CARTESIAN_POINT('Ctrl Pts',(-0.136684990383263,-0.0034813894794369,
3.6));
#33269=CARTESIAN_POINT('Ctrl Pts',(-0.135720534319688,0.00492632812693493,
3.6));
#33270=CARTESIAN_POINT('Ctrl Pts',(-0.134014244604164,0.0131981027910972,
3.6));
#33271=CARTESIAN_POINT('Ctrl Pts',(-0.133007067351581,0.0180807104774909,
3.6));
#33272=CARTESIAN_POINT('Ctrl Pts',(-0.131740913976379,0.0229158302155836,
3.6));
#33273=CARTESIAN_POINT('Ctrl Pts',(-0.130217237780107,0.0276776331326924,
3.6));
#33274=CARTESIAN_POINT('Ctrl Pts',(-0.129150755329031,0.0310106111361586,
3.6));
#33275=CARTESIAN_POINT('Ctrl Pts',(-0.127957851528495,0.0343071390648417,
3.6));
#33276=CARTESIAN_POINT('Ctrl Pts',(-0.126644351454204,0.0375455932808108,
3.6));
#33277=CARTESIAN_POINT('Ctrl Pts',(-0.12454778430103,0.0427147111736446,
3.6));
#33278=CARTESIAN_POINT('Ctrl Pts',(-0.122141614879321,0.0477447959908898,
3.6));
#33279=CARTESIAN_POINT('Ctrl Pts',(-0.11942949850221,0.0525991124010946,
3.6));
#33280=CARTESIAN_POINT('Ctrl Pts',(-0.116867678035268,0.0571844197417489,
3.6));
#33281=CARTESIAN_POINT('Ctrl Pts',(-0.11402973916396,0.0616160698651957,
3.6));
#33282=CARTESIAN_POINT('Ctrl Pts',(-0.110933547566151,0.0658375038383711,
3.6));
#33283=CARTESIAN_POINT('Ctrl Pts',(-0.107383747559623,0.0706774001665366,
3.6));
#33284=CARTESIAN_POINT('Ctrl Pts',(-0.103491800365401,0.0752476578095535,
3.6));
#33285=CARTESIAN_POINT('Ctrl Pts',(-0.0992594032733973,0.0794964740507377,
3.6));
#33286=CARTESIAN_POINT('Ctrl Pts',(-0.0981916513129811,0.080568368245057,
3.6));
#33287=CARTESIAN_POINT('Ctrl Pts',(-0.0971022039419119,0.081619760070457,
3.6));
#33288=CARTESIAN_POINT('Ctrl Pts',(-0.0959917963302726,0.0826503396631628,
3.6));
#33289=CARTESIAN_POINT('Origin',(0.,0.,3.1));
#33290=CARTESIAN_POINT('Origin',(0.,0.,2.6));
#33291=CARTESIAN_POINT('Origin',(4.61329551933804E-18,0.,1.7));
#33292=CARTESIAN_POINT('Ctrl Pts',(0.163512932725146,-0.0319230454628286,
1.7));
#33293=CARTESIAN_POINT('Ctrl Pts',(0.162868713265022,-0.0402193660776135,
1.7));
#33294=CARTESIAN_POINT('Ctrl Pts',(0.161556142957416,-0.0484298106643142,
1.7));
#33295=CARTESIAN_POINT('Ctrl Pts',(0.159633648446255,-0.0565030284772356,
1.7));
#33296=CARTESIAN_POINT('Ctrl Pts',(0.15857220935963,-0.0609603774536462,
1.7));
#33297=CARTESIAN_POINT('Ctrl Pts',(0.15732455882578,-0.0653759608776499,
1.7));
#33298=CARTESIAN_POINT('Ctrl Pts',(0.155898537051345,-0.0697413060244838,
1.7));
#33299=CARTESIAN_POINT('Ctrl Pts',(0.154359565759251,-0.0744524128122629,
1.7));
#33300=CARTESIAN_POINT('Ctrl Pts',(0.152615240924071,-0.0790971028454583,
1.7));
#33301=CARTESIAN_POINT('Ctrl Pts',(0.150679159438777,-0.0836586618069671,
1.7));
#33302=CARTESIAN_POINT('Ctrl Pts',(0.147458757270998,-0.0912461804520635,
1.7));
#33303=CARTESIAN_POINT('Ctrl Pts',(0.143706663154478,-0.098609365081655,
1.7));
#33304=CARTESIAN_POINT('Ctrl Pts',(0.139465780840256,-0.105699927668597,
1.7));
#33305=CARTESIAN_POINT('Ctrl Pts',(0.137613322919106,-0.108797153164702,
1.7));
#33306=CARTESIAN_POINT('Ctrl Pts',(0.135667748856481,-0.111841429389798,
1.7));
#33307=CARTESIAN_POINT('Ctrl Pts',(0.133638504154441,-0.114820282936825,
1.7));
#33308=CARTESIAN_POINT('Ctrl Pts',(0.126764362615545,-0.124911259587064,
1.7));
#33309=CARTESIAN_POINT('Ctrl Pts',(0.118918297697151,-0.134279562536914,
1.7));
#33310=CARTESIAN_POINT('Ctrl Pts',(0.110233695412878,-0.142776634038112,
1.7));
#33311=CARTESIAN_POINT('Ctrl Pts',(0.1060042704444,-0.146914731004415,1.7));
#33312=CARTESIAN_POINT('Ctrl Pts',(0.101575189643516,-0.150846009251356,
1.7));
#33313=CARTESIAN_POINT('Ctrl Pts',(0.0969579219100265,-0.154551255269456,
1.7));
#33314=CARTESIAN_POINT('Ctrl Pts',(0.0930558717128837,-0.157682556460965,
1.7));
#33315=CARTESIAN_POINT('Ctrl Pts',(0.089014879864356,-0.160654885938173,
1.7));
#33316=CARTESIAN_POINT('Ctrl Pts',(0.084867234382875,-0.163439189909414,
1.7));
#33317=CARTESIAN_POINT('Ctrl Pts',(0.0797924645177416,-0.166845870145637,
1.7));
#33318=CARTESIAN_POINT('Ctrl Pts',(0.0745525511585738,-0.169976381556328,
1.7));
#33319=CARTESIAN_POINT('Ctrl Pts',(0.069162704388918,-0.172812601917057,
1.7));
#33320=CARTESIAN_POINT('Ctrl Pts',(0.0615917910053332,-0.176796533113158,
1.7));
#33321=CARTESIAN_POINT('Ctrl Pts',(0.0537253644412386,-0.180200415745643,
1.7));
#33322=CARTESIAN_POINT('Ctrl Pts',(0.0456302879589726,-0.183039981733068,
1.7));
#33323=CARTESIAN_POINT('Ctrl Pts',(0.039725979220554,-0.185111076961087,
1.7));
#33324=CARTESIAN_POINT('Ctrl Pts',(0.0336998028892366,-0.186881755092485,
1.7));
#33325=CARTESIAN_POINT('Ctrl Pts',(0.027575472779275,-0.188354488495274,
1.7));
#33326=CARTESIAN_POINT('Ctrl Pts',(0.0240503901388611,-0.189202174178265,
1.7));
#33327=CARTESIAN_POINT('Ctrl Pts',(0.0204971902089821,-0.189949869388286,
1.7));
#33328=CARTESIAN_POINT('Ctrl Pts',(0.0169287682122467,-0.190597281499825,
1.7));
#33329=CARTESIAN_POINT('Ctrl Pts',(0.00540716645046445,-0.192687624102725,
1.7));
#33330=CARTESIAN_POINT('Ctrl Pts',(-0.00629626416002409,-0.193741044106324,
1.7));
#33331=CARTESIAN_POINT('Ctrl Pts',(-0.0180243092057446,-0.193790924616578,
1.7));
#33332=CARTESIAN_POINT('Ctrl Pts',(-0.0246815057039127,-0.193819238317361,
1.7));
#33333=CARTESIAN_POINT('Ctrl Pts',(-0.0313470218059255,-0.19352361589825,
1.7));
#33334=CARTESIAN_POINT('Ctrl Pts',(-0.0379937712674718,-0.192905366089908,
1.7));
#33335=CARTESIAN_POINT('Ctrl Pts',(-0.0421040672802865,-0.192523045417697,
1.7));
#33336=CARTESIAN_POINT('Ctrl Pts',(-0.0462092418665425,-0.192016959216387,
1.7));
#33337=CARTESIAN_POINT('Ctrl Pts',(-0.0502964475671879,-0.191387744025229,
1.7));
#33338=CARTESIAN_POINT('Ctrl Pts',(-0.0635557644152557,-0.189346505047739,
1.7));
#33339=CARTESIAN_POINT('Ctrl Pts',(-0.076538642829352,-0.186027878905466,
1.7));
#33340=CARTESIAN_POINT('Ctrl Pts',(-0.0890304894083597,-0.181464562959599,
1.7));
#33341=CARTESIAN_POINT('Ctrl Pts',(-0.0993708472336289,-0.177687193500922,
1.7));
#33342=CARTESIAN_POINT('Ctrl Pts',(-0.109375752092602,-0.173056097632409,
1.7));
#33343=CARTESIAN_POINT('Ctrl Pts',(-0.118921685270779,-0.167562801749516,
1.7));
#33344=CARTESIAN_POINT('Ctrl Pts',(-0.120076087508369,-0.166898490263086,
1.7));
#33345=CARTESIAN_POINT('Ctrl Pts',(-0.121223766120909,-0.16622153952215,
1.7));
#33346=CARTESIAN_POINT('Ctrl Pts',(-0.122364641233049,-0.165532117868825,
1.7));
#33347=CARTESIAN_POINT('Ctrl Pts',(-0.188262750966375,-0.0823232180103074,
1.7));
#33348=CARTESIAN_POINT('Ctrl Pts',(-0.190918693248964,-0.0742705707004131,
1.7));
#33349=CARTESIAN_POINT('Ctrl Pts',(-0.193028471001937,-0.0660604959755095,
1.7));
#33350=CARTESIAN_POINT('Ctrl Pts',(-0.194604369739905,-0.0577442961437627,
1.7));
#33351=CARTESIAN_POINT('Ctrl Pts',(-0.195791431603972,-0.0514800334494749,
1.7));
#33352=CARTESIAN_POINT('Ctrl Pts',(-0.196675380086104,-0.0451554970342283,
1.7));
#33353=CARTESIAN_POINT('Ctrl Pts',(-0.197258353741452,-0.0387928833243269,
1.7));
#33354=CARTESIAN_POINT('Ctrl Pts',(-0.197694864529353,-0.0340287752070089,
1.7));
#33355=CARTESIAN_POINT('Ctrl Pts',(-0.197962173616876,-0.0292446940334784,
1.7));
#33356=CARTESIAN_POINT('Ctrl Pts',(-0.198061149421263,-0.0244622127102265,
1.7));
#33357=CARTESIAN_POINT('Ctrl Pts',(-0.198268317226716,-0.0144519261913088,
1.7));
#33358=CARTESIAN_POINT('Ctrl Pts',(-0.197740578304783,-0.00443368324017007,
1.7));
#33359=CARTESIAN_POINT('Ctrl Pts',(-0.196485470149517,0.00550410801291526,
1.7));
#33360=CARTESIAN_POINT('Ctrl Pts',(-0.19583094903621,0.0106865252950324,
1.7));
#33361=CARTESIAN_POINT('Ctrl Pts',(-0.194977340636945,0.0158499464463904,
1.7));
#33362=CARTESIAN_POINT('Ctrl Pts',(-0.193930228257619,0.0209568152791792,
1.7));
#33363=CARTESIAN_POINT('Ctrl Pts',(-0.191365358848382,0.0334659326431063,
1.7));
#33364=CARTESIAN_POINT('Ctrl Pts',(-0.187640262305008,0.0456682931313192,
1.7));
#33365=CARTESIAN_POINT('Ctrl Pts',(-0.18276823303275,0.0573755743540122,
1.7));
#33366=CARTESIAN_POINT('Ctrl Pts',(-0.180530605205125,0.0627524998168591,
1.7));
#33367=CARTESIAN_POINT('Ctrl Pts',(-0.178050427357818,0.0680246443278264,
1.7));
#33368=CARTESIAN_POINT('Ctrl Pts',(-0.175326059031915,0.0731713030262629,
1.7));
#33369=CARTESIAN_POINT('Ctrl Pts',(-0.173546095954943,0.0765338668785476,
1.7));
#33370=CARTESIAN_POINT('Ctrl Pts',(-0.171660782837765,0.0798445731517242,
1.7));
#33371=CARTESIAN_POINT('Ctrl Pts',(-0.169672721187811,0.0830915804684565,
1.7));
#33372=CARTESIAN_POINT('Ctrl Pts',(-0.165401890376176,0.0900669269795776,
1.7));
#33373=CARTESIAN_POINT('Ctrl Pts',(-0.160674569826176,0.0967219627994757,
1.7));
#33374=CARTESIAN_POINT('Ctrl Pts',(-0.15549277623518,0.103004446710986,
1.7));
#33375=CARTESIAN_POINT('Ctrl Pts',(-0.149788864011586,0.109919955047648,
1.7));
#33376=CARTESIAN_POINT('Ctrl Pts',(-0.143534087392955,0.116384355174537,
1.7));
#33377=CARTESIAN_POINT('Ctrl Pts',(-0.1368007840805,0.122364607652698,1.7));
#33378=CARTESIAN_POINT('Ctrl Pts',(-0.132573081040691,0.126119485519849,
1.7));
#33379=CARTESIAN_POINT('Ctrl Pts',(-0.128156557788873,0.129683253321797,
1.7));
#33380=CARTESIAN_POINT('Ctrl Pts',(-0.123568264594465,0.133044997940945,
1.7));
#33381=CARTESIAN_POINT('Ctrl Pts',(-0.120777285576228,0.135089888774893,
1.7));
#33382=CARTESIAN_POINT('Ctrl Pts',(-0.117925900172203,0.137057490795076,
1.7));
#33383=CARTESIAN_POINT('Ctrl Pts',(-0.115025210475747,0.138941543144738,
1.7));
#33384=CARTESIAN_POINT('Ctrl Pts',(-0.106405133477763,0.144540444792911,
1.7));
#33385=CARTESIAN_POINT('Ctrl Pts',(-0.0973325886051703,0.149416450333531,
1.7));
#33386=CARTESIAN_POINT('Ctrl Pts',(-0.0879171639429846,0.15351829690281,
1.7));
#33387=CARTESIAN_POINT('Ctrl Pts',(-0.0791136675584941,0.157353555825057,
1.7));
#33388=CARTESIAN_POINT('Ctrl Pts',(-0.0700097444331976,0.160511945106675,
1.7));
#33389=CARTESIAN_POINT('Ctrl Pts',(-0.0606944403481407,0.162929898574301,
1.7));
#33390=CARTESIAN_POINT('Ctrl Pts',(-0.0571572012739495,0.163848052121106,
1.7));
#33391=CARTESIAN_POINT('Ctrl Pts',(-0.0535976091548405,0.16465702786045,
1.7));
#33392=CARTESIAN_POINT('Ctrl Pts',(-0.0500249348171965,0.165353504526832,
1.7));
#33393=CARTESIAN_POINT('Ctrl Pts',(-0.0389427731093366,0.16751392171383,
1.7));
#33394=CARTESIAN_POINT('Ctrl Pts',(-0.0277208597802445,0.168598940439913,
1.7));
#33395=CARTESIAN_POINT('Ctrl Pts',(-0.016510036378599,0.168511954471149,
1.7));
#33396=CARTESIAN_POINT('Ctrl Pts',(-0.0103145529256217,0.168463883057408,
1.7));
#33397=CARTESIAN_POINT('Ctrl Pts',(-0.00412256070196868,0.168057036314866,
1.7));
#33398=CARTESIAN_POINT('Ctrl Pts',(0.00203815650313415,0.16726854038896,
1.7));
#33399=CARTESIAN_POINT('Ctrl Pts',(0.00311390584534565,0.167130857722252,
1.7));
#33400=CARTESIAN_POINT('Ctrl Pts',(0.00418869523159273,0.166981526327298,
1.7));
#33401=CARTESIAN_POINT('Ctrl Pts',(0.00526237188779194,0.16682061735739,
1.7));
#33402=CARTESIAN_POINT('Origin',(0.,0.,0.645407471946233));
#33403=CARTESIAN_POINT('Ctrl Pts',(0.205654271051376,0.000148184871923513,
0.820407471946232));
#33404=CARTESIAN_POINT('Ctrl Pts',(0.20573642152142,0.00997667026911825,
0.820941869468311));
#33405=CARTESIAN_POINT('Ctrl Pts',(0.200629007389055,0.0878566204334846,
0.825180863342659));
#33406=CARTESIAN_POINT('Ctrl Pts',(0.101090873180113,0.220844643128561,
0.833124453569275));
#33407=CARTESIAN_POINT('Ctrl Pts',(-0.130696704329673,0.204681987270635,
0.844238242626078));
#33408=CARTESIAN_POINT('Ctrl Pts',(-0.242858579725743,0.00121498249237738,
0.855352031682883));
#33409=CARTESIAN_POINT('Ctrl Pts',(-0.132727951496213,-0.203386773400678,
0.866465820739686));
#33410=CARTESIAN_POINT('Ctrl Pts',(0.0988894015246068,-0.221814471640749,
0.877579609796491));
#33411=CARTESIAN_POINT('Ctrl Pts',(0.200212227802606,-0.0892608439806378,
0.885560160198673));
#33412=CARTESIAN_POINT('Ctrl Pts',(0.205725385245381,-0.0106740336596208,
0.889836114248587));
#33413=CARTESIAN_POINT('Ctrl Pts',(0.205635165348036,-0.000160487501855345,
0.890407471946233));
#33414=CARTESIAN_POINT('Ctrl Pts',(0.205269394176581,-0.000252214316689755,
0.814592528053767));
#33415=CARTESIAN_POINT('Ctrl Pts',(0.204912576919524,0.0467765744646069,
0.817137544740381));
#33416=CARTESIAN_POINT('Ctrl Pts',(0.165648098003252,0.162976258711784,
0.823387157779263));
#33417=CARTESIAN_POINT('Ctrl Pts',(-0.0272119409517698,0.241262826763902,
0.833341367170412));
#33418=CARTESIAN_POINT('Ctrl Pts',(-0.217470922739143,0.108102090643486,
0.844455156227217));
#33419=CARTESIAN_POINT('Ctrl Pts',(-0.208759451561279,-0.124141896006793,
0.85556894528402));
#33420=CARTESIAN_POINT('Ctrl Pts',(-0.00892472216375234,-0.242686445659381,
0.866682734340826));
#33421=CARTESIAN_POINT('Ctrl Pts',(0.172122246966409,-0.152544606240875,
0.87635726193074));
#33422=CARTESIAN_POINT('Ctrl Pts',(0.20498850808804,-0.0417917950361515,
0.882327193168388));
#33423=CARTESIAN_POINT('Ctrl Pts',(0.205205445749305,0.000116004416325009,
0.884592528053768));
#33424=CARTESIAN_POINT('Ctrl Pts',(-0.126907087985236,0.107935865304854,
0.8));
#33425=CARTESIAN_POINT('Ctrl Pts',(-0.162798331100657,0.0657362393039544,
0.803704596352268));
#33426=CARTESIAN_POINT('Ctrl Pts',(-0.188554427056889,-0.0565517713871986,
0.811113789056805));
#33427=CARTESIAN_POINT('Ctrl Pts',(-0.0544936724634594,-0.189356862721456,
0.822227578113607));
#33428=CARTESIAN_POINT('Ctrl Pts',(0.12941144825895,-0.14834225030535,0.833341367170414));
#33429=CARTESIAN_POINT('Ctrl Pts',(0.194879695227305,0.0282018585329969,
0.844455156227216));
#33430=CARTESIAN_POINT('Ctrl Pts',(0.0819649080024663,0.179061771725117,
0.855568945284021));
#33431=CARTESIAN_POINT('Ctrl Pts',(-0.105969441252334,0.165957021921342,
0.866682734340825));
#33432=CARTESIAN_POINT('Ctrl Pts',(-0.196910764727139,0.000985112949166876,
0.877796523397629));
#33433=CARTESIAN_POINT('Ctrl Pts',(-0.107616385055452,-0.164906857031527,
0.888910312454434));
#33434=CARTESIAN_POINT('Ctrl Pts',(0.0801799454629491,-0.179848112789142,
0.900024101511237));
#33435=CARTESIAN_POINT('Ctrl Pts',(0.194586948216313,-0.0301773643334041,
0.911137890568042));
#33436=CARTESIAN_POINT('Ctrl Pts',(0.13088616131906,0.147117686303235,0.922251679624846));
#33437=CARTESIAN_POINT('Ctrl Pts',(-0.0526161354638876,0.18975288262963,
0.93336546868165));
#33438=CARTESIAN_POINT('Ctrl Pts',(-0.187958327447607,0.0587058278606146,
0.944479257738454));
#33439=CARTESIAN_POINT('Ctrl Pts',(-0.151260109468812,-0.126075710016806,
0.955593046795258));
#33440=CARTESIAN_POINT('Ctrl Pts',(0.0238881910101356,-0.195458525846084,
0.966706835852062));
#33441=CARTESIAN_POINT('Ctrl Pts',(0.177171365146215,-0.0859360381031547,
0.977820624908868));
#33442=CARTESIAN_POINT('Ctrl Pts',(0.168287576475019,0.102244733060238,
0.98893441396567));
#33443=CARTESIAN_POINT('Ctrl Pts',(0.00536826212740452,0.196839712751384,
1.00004820302248));
#33444=CARTESIAN_POINT('Ctrl Pts',(-0.162464684252001,0.111265085550637,
1.01116199207928));
#33445=CARTESIAN_POINT('Ctrl Pts',(-0.181591862229106,-0.076151743861926,
1.02227578113608));
#33446=CARTESIAN_POINT('Ctrl Pts',(-0.0345059495415616,-0.193866014541413,
1.03338957019289));
#33447=CARTESIAN_POINT('Ctrl Pts',(0.144163650203206,-0.134132525587662,
1.04450335924969));
#33448=CARTESIAN_POINT('Ctrl Pts',(0.190878625928487,0.0483739862822188,
1.0556171483065));
#33449=CARTESIAN_POINT('Ctrl Pts',(0.062880230662697,0.186603239345861,
1.0667309373633));
#33450=CARTESIAN_POINT('Ctrl Pts',(-0.122673152855754,0.154032431506053,
1.07784472642011));
#33451=CARTESIAN_POINT('Ctrl Pts',(-0.195942408348395,-0.019526007891641,
1.08895851547691));
#33452=CARTESIAN_POINT('Ctrl Pts',(-0.0898633553462809,-0.175212070745787,
1.10007230453371));
#33453=CARTESIAN_POINT('Ctrl Pts',(0.0984686459264395,-0.170524538248248,
1.11118609359052));
#33454=CARTESIAN_POINT('Ctrl Pts',(0.196671178871044,-0.00975396199037572,
1.12229988264732));
#33455=CARTESIAN_POINT('Ctrl Pts',(0.114858351392768,0.159944526283292,
1.13341367170412));
#33456=CARTESIAN_POINT('Ctrl Pts',(-0.0720856276979479,0.183243975761544,
1.14452746076093));
#33457=CARTESIAN_POINT('Ctrl Pts',(-0.193048814249935,0.0388181360941049,
1.15564124981773));
#33458=CARTESIAN_POINT('Ctrl Pts',(-0.13731223179659,-0.141138383766243,
1.16675503887454));
#33459=CARTESIAN_POINT('Ctrl Pts',(0.0441077936468435,-0.191909340348063,
1.17786882793134));
#33460=CARTESIAN_POINT('Ctrl Pts',(0.185155455348894,-0.0670235013089116,
1.18898261698815));
#33461=CARTESIAN_POINT('Ctrl Pts',(0.156728228964436,0.119209708576257,
1.20009640604495));
#33462=CARTESIAN_POINT('Ctrl Pts',(-0.0151541228101832,0.196328920271653,
1.21121019510176));
#33463=CARTESIAN_POINT('Ctrl Pts',(-0.173165734117196,0.0937460447209521,
1.22232398415856));
#33464=CARTESIAN_POINT('Ctrl Pts',(-0.172676785153749,-0.0946436487152594,
1.23343777321536));
#33465=CARTESIAN_POINT('Ctrl Pts',(-0.0141348164511399,-0.196404937150434,
1.24455156227217));
#33466=CARTESIAN_POINT('Ctrl Pts',(0.157344910048918,-0.118394559228326,
1.25566535132897));
#33467=CARTESIAN_POINT('Ctrl Pts',(0.184805055968556,0.0679837014410847,
1.26677914038578));
#33468=CARTESIAN_POINT('Ctrl Pts',(0.0431110383282961,0.192135709193865,
1.27789292944258));
#33469=CARTESIAN_POINT('Ctrl Pts',(-0.138043001606285,0.140423723354349,
1.28900671849938));
#33470=CARTESIAN_POINT('Ctrl Pts',(-0.192844716656512,-0.0398196889847226,
1.30012050755619));
#33471=CARTESIAN_POINT('Ctrl Pts',(-0.0711334755432105,-0.183615688410121,
1.31123429661299));
#33472=CARTESIAN_POINT('Ctrl Pts',(0.115687042443292,-0.159346165890141,
1.32234808566979));
#33473=CARTESIAN_POINT('Ctrl Pts',(0.196617898501115,0.0107747093774004,
1.3334618747266));
#33474=CARTESIAN_POINT('Ctrl Pts',(0.0975821622623196,0.171033370958511,
1.3445756637834));
#33475=CARTESIAN_POINT('Ctrl Pts',(-0.0907716337523168,0.174743248450528,
1.35568945284021));
#33476=CARTESIAN_POINT('Ctrl Pts',(-0.196041123972824,0.0185086489133565,
1.36680324189701));
#33477=CARTESIAN_POINT('Ctrl Pts',(-0.121871950164007,-0.1546671268781,
1.37791703095382));
#33478=CARTESIAN_POINT('Ctrl Pts',(0.0638480017529153,-0.186274327390575,
1.38903082001062));
#33479=CARTESIAN_POINT('Ctrl Pts',(0.191127153577756,-0.0473825235535316,
1.40014460906743));
#33480=CARTESIAN_POINT('Ctrl Pts',(0.143465454207459,0.134879041457197,
1.41125839812423));
#33481=CARTESIAN_POINT('Ctrl Pts',(-0.0355118024153517,0.193684290169161,
1.42237218718103));
#33482=CARTESIAN_POINT('Ctrl Pts',(-0.181984703541769,0.0752081115995363,
1.43348597623784));
#33483=CARTESIAN_POINT('Ctrl Pts',(-0.16188494169705,-0.112106904510744,
1.44459976529464));
#33484=CARTESIAN_POINT('Ctrl Pts',(0.00638994323583646,-0.196809199398823,
1.45571355435144));
#33485=CARTESIAN_POINT('Ctrl Pts',(0.168816040557079,-0.101369802386164,
1.46682734340825));
#33486=CARTESIAN_POINT('Ctrl Pts',(0.17672290164568,0.0868545248928826,
1.47794113246505));
#33487=CARTESIAN_POINT('Ctrl Pts',(0.0228732863137639,0.195579919524334,
1.48905492152186));
#33488=CARTESIAN_POINT('Ctrl Pts',(-0.15191250667306,0.125288797732896,
1.50016871057866));
#33489=CARTESIAN_POINT('Ctrl Pts',(-0.187651060854054,-0.0596805852186566,
1.51128249963547));
#33490=CARTESIAN_POINT('Ctrl Pts',(-0.0516304683294577,-0.190023644566662,
1.52239628869227));
#33491=CARTESIAN_POINT('Ctrl Pts',(0.131648072412201,-0.146435920677088,
1.53351007774908));
#33492=CARTESIAN_POINT('Ctrl Pts',(0.194427649007747,0.0311862882363455,
1.54462386680588));
#33493=CARTESIAN_POINT('Ctrl Pts',(0.0792453752737409,0.180263283819487,
1.55573765586268));
#33494=CARTESIAN_POINT('Ctrl Pts',(-0.108471054243311,0.164343347185408,
1.56685144491949));
#33495=CARTESIAN_POINT('Ctrl Pts',(-0.196902764500876,-0.00200210229874768,
1.57796523397629));
#33496=CARTESIAN_POINT('Ctrl Pts',(-0.105107013422145,-0.16651465373019,
1.5890790230331));
#33497=CARTESIAN_POINT('Ctrl Pts',(0.0828941340502818,-0.178615126425815,
1.6001928120899));
#33498=CARTESIAN_POINT('Ctrl Pts',(0.195021809584276,-0.0272258612485208,
1.61130660114671));
#33499=CARTESIAN_POINT('Ctrl Pts',(0.128642913099457,0.149081079408297,
1.62242039020351));
#33500=CARTESIAN_POINT('Ctrl Pts',(-0.0554825813599488,0.188937135031884,
1.63353417926031));
#33501=CARTESIAN_POINT('Ctrl Pts',(-0.188827531603801,0.0558478560140352,
1.64464796831712));
#33502=CARTESIAN_POINT('Ctrl Pts',(-0.149330198326453,-0.128342305854753,
1.65576175737392));
#33503=CARTESIAN_POINT('Ctrl Pts',(0.0268386909069323,-0.195092411199392,
1.66687554643073));
#33504=CARTESIAN_POINT('Ctrl Pts',(0.178464943022445,-0.0832088009083063,
1.67798933548753));
#33505=CARTESIAN_POINT('Ctrl Pts',(0.166695798680381,0.104715122443915,
1.68910312454433));
#33506=CARTESIAN_POINT('Ctrl Pts',(0.00243441762381693,0.197027042329472,
1.70021691360114));
#33507=CARTESIAN_POINT('Ctrl Pts',(-0.164232046005026,0.108529764925501,
1.71133070265794));
#33508=CARTESIAN_POINT('Ctrl Pts',(-0.174839538171076,-0.0159901738299179,
1.71873989536248));
#33509=CARTESIAN_POINT('Ctrl Pts',(-0.152644235605294,-0.0667480137268189,
1.72244449171475));
#33510=CARTESIAN_POINT('Ctrl Pts',(-0.136778062465881,0.116331236980977,
0.792518502761751));
#33511=CARTESIAN_POINT('Ctrl Pts',(-0.175460966397852,0.0708492771249652,
0.796223099114019));
#33512=CARTESIAN_POINT('Ctrl Pts',(-0.203220400149799,-0.0609504310764289,
0.803632291818556));
#33513=CARTESIAN_POINT('Ctrl Pts',(-0.0587322509288797,-0.204085250153022,
0.814746080875359));
#33514=CARTESIAN_POINT('Ctrl Pts',(0.139477214667647,-0.159880475556692,
0.825859869932165));
#33515=CARTESIAN_POINT('Ctrl Pts',(0.210037654715023,0.0303954304627091,
0.836973658988967));
#33516=CARTESIAN_POINT('Ctrl Pts',(0.0883402297283485,0.192989395526265,
0.848087448045772));
#33517=CARTESIAN_POINT('Ctrl Pts',(-0.114211862278114,0.178865343704439,
0.859201237102576));
#33518=CARTESIAN_POINT('Ctrl Pts',(-0.212226703060007,0.00106173613023704,
0.87031502615938));
#33519=CARTESIAN_POINT('Ctrl Pts',(-0.115986907202372,-0.177733495821244,
0.881428815216186));
#33520=CARTESIAN_POINT('Ctrl Pts',(0.0864164308168349,-0.193836899073011,
0.892542604272987));
#33521=CARTESIAN_POINT('Ctrl Pts',(0.209722137515851,-0.0325245933019137,
0.903656393329794));
#33522=CARTESIAN_POINT('Ctrl Pts',(0.141066632550109,0.158560663604232,
0.914770182386597));
#33523=CARTESIAN_POINT('Ctrl Pts',(-0.0567086770128242,0.204512072930204,
0.925883971443401));
#33524=CARTESIAN_POINT('Ctrl Pts',(-0.20257793524978,0.0632720324586165,
0.936997760500206));
#33525=CARTESIAN_POINT('Ctrl Pts',(-0.163025289051846,-0.135882018994204,
0.948111549557009));
#33526=CARTESIAN_POINT('Ctrl Pts',(0.025746241081202,-0.210661507423248,
0.959225338613814));
#33527=CARTESIAN_POINT('Ctrl Pts',(0.190951951020682,-0.0926202387459321,
0.970339127670618));
#33528=CARTESIAN_POINT('Ctrl Pts',(0.181377171383915,0.110197442139303,
0.981452916727422));
#33529=CARTESIAN_POINT('Ctrl Pts',(0.00578581152757031,0.212150124582537,
0.992566705784226));
#33530=CARTESIAN_POINT('Ctrl Pts',(-0.175101368126144,0.119919407681051,
1.00368049484103));
#33531=CARTESIAN_POINT('Ctrl Pts',(-0.195716279284241,-0.0820749112141317,
1.01479428389783));
#33532=CARTESIAN_POINT('Ctrl Pts',(-0.0371898606828745,-0.208945128817718,
1.02590807295464));
#33533=CARTESIAN_POINT('Ctrl Pts',(0.15537685929014,-0.144565502642925,
1.03702186201144));
#33534=CARTESIAN_POINT('Ctrl Pts',(0.205725377795173,0.0521365687486478,
1.04813565106825));
#33535=CARTESIAN_POINT('Ctrl Pts',(0.0677711249544383,0.201117446888019,
1.05924944012505));
#33536=CARTESIAN_POINT('Ctrl Pts',(-0.132214807152008,0.166013245381199,
1.07036322918185));
#33537=CARTESIAN_POINT('Ctrl Pts',(-0.211183026844882,-0.0210447625070621,
1.08147701823866));
#33538=CARTESIAN_POINT('Ctrl Pts',(-0.0968530270931527,-0.188840260522183,
1.09259080729546));
#33539=CARTESIAN_POINT('Ctrl Pts',(0.106127646747548,-0.183788126532363,
1.10370459635227));
#33540=CARTESIAN_POINT('Ctrl Pts',(0.211968481949499,-0.0105126360047333,
1.11481838540907));
#33541=CARTESIAN_POINT('Ctrl Pts',(0.123792161737694,0.172385189467092,
1.12593217446588));
#33542=CARTESIAN_POINT('Ctrl Pts',(-0.0776925280115889,0.197496896045118,
1.13704596352268));
#33543=CARTESIAN_POINT('Ctrl Pts',(-0.208064365778478,0.0418374539025449,
1.14815975257949));
#33544=CARTESIAN_POINT('Ctrl Pts',(-0.147992529938032,-0.152116284264268,
1.15927354163629));
#33545=CARTESIAN_POINT('Ctrl Pts',(0.0475385469041886,-0.206836262328918,
1.17038733069309));
#33546=CARTESIAN_POINT('Ctrl Pts',(0.199557052641187,-0.0722366638006762,
1.1815011197499));
#33547=CARTESIAN_POINT('Ctrl Pts',(0.168918724964821,0.12848197232356,1.1926149088067));
#33548=CARTESIAN_POINT('Ctrl Pts',(-0.0163328273404871,0.211599602095504,
1.2037286978635));
#33549=CARTESIAN_POINT('Ctrl Pts',(-0.186634757554183,0.101037716366665,
1.21484248692031));
#33550=CARTESIAN_POINT('Ctrl Pts',(-0.18610777759643,-0.102005136998184,
1.22595627597711));
#33551=CARTESIAN_POINT('Ctrl Pts',(-0.0152342381989151,-0.211681531651681,
1.23707006503392));
#33552=CARTESIAN_POINT('Ctrl Pts',(0.169583372190078,-0.127603419752538,
1.24818385409072));
#33553=CARTESIAN_POINT('Ctrl Pts',(0.199179398807247,0.0732715493672994,
1.25929764314753));
#33554=CARTESIAN_POINT('Ctrl Pts',(0.046464262848129,0.207080238395369,
1.27041143220433));
#33555=CARTESIAN_POINT('Ctrl Pts',(-0.148780139836465,0.151346036770516,
1.28152522126114));
#33556=CARTESIAN_POINT('Ctrl Pts',(-0.207844393247192,-0.0429169086911673,
1.29263901031794));
#33557=CARTESIAN_POINT('Ctrl Pts',(-0.0766663164030391,-0.197897520917011,
1.30375279937474));
#33558=CARTESIAN_POINT('Ctrl Pts',(0.124685309300001,-0.171740287936918,
1.31486658843155));
#33559=CARTESIAN_POINT('Ctrl Pts',(0.211911057373125,0.0116127782590458,
1.32598037748835));
#33560=CARTESIAN_POINT('Ctrl Pts',(0.105172211397869,0.184336536816879,
1.33709416654516));
#33561=CARTESIAN_POINT('Ctrl Pts',(-0.0978319524040202,0.188334972707259,
1.34820795560196));
#33562=CARTESIAN_POINT('Ctrl Pts',(-0.211289420680394,0.0199482722156909,
1.35932174465877));
#33563=CARTESIAN_POINT('Ctrl Pts',(-0.131351286023602,-0.166697308065347,
1.37043553371557));
#33564=CARTESIAN_POINT('Ctrl Pts',(0.068814170356646,-0.200762951794954,
1.38154932277237));
#33565=CARTESIAN_POINT('Ctrl Pts',(0.205993236201476,-0.0510679889459757,
1.39266311182918));
#33566=CARTESIAN_POINT('Ctrl Pts',(0.154624356833139,0.14537008334725,1.40377690088598));
#33567=CARTESIAN_POINT('Ctrl Pts',(-0.0382739499121438,0.208749269721634,
1.41489068994279));
#33568=CARTESIAN_POINT('Ctrl Pts',(-0.196139676231217,0.0810578821846344,
1.42600447899959));
#33569=CARTESIAN_POINT('Ctrl Pts',(-0.174476532550337,-0.120826704256352,
1.43711826805639));
#33570=CARTESIAN_POINT('Ctrl Pts',(0.00688696012917997,-0.212117237867469,
1.4482320571132));
#33571=CARTESIAN_POINT('Ctrl Pts',(0.181946739990165,-0.109254458384087,
1.45934584617));
#33572=CARTESIAN_POINT('Ctrl Pts',(0.190468605530186,0.0936101664599312,
1.47045963522681));
#33573=CARTESIAN_POINT('Ctrl Pts',(0.0246523959685209,0.210792343236835,
1.48157342428361));
#33574=CARTESIAN_POINT('Ctrl Pts',(-0.163728430436396,0.135033899797455,
1.49268721334042));
#33575=CARTESIAN_POINT('Ctrl Pts',(-0.202246769118763,-0.0643226075283309,
1.50380100239722));
#33576=CARTESIAN_POINT('Ctrl Pts',(-0.0556463435921781,-0.204803895031906,
1.51491479145403));
#33577=CARTESIAN_POINT('Ctrl Pts',(0.141887805935659,-0.157825869489257,
1.52602858051082));
#33578=CARTESIAN_POINT('Ctrl Pts',(0.209550447837631,0.0336119924283981,
1.53714236956763));
#33579=CARTESIAN_POINT('Ctrl Pts',(0.0854091687186523,0.194284362567952,
1.54825615862443));
#33580=CARTESIAN_POINT('Ctrl Pts',(-0.116908053510435,0.177126155552421,
1.55936994768124));
#33581=CARTESIAN_POINT('Ctrl Pts',(-0.212218080567246,-0.00215782804277307,
1.57048373673804));
#33582=CARTESIAN_POINT('Ctrl Pts',(-0.113282353851889,-0.179466348735714,
1.58159752579485));
#33583=CARTESIAN_POINT('Ctrl Pts',(0.089341732011876,-0.192508009658716,
1.59271131485165));
#33584=CARTESIAN_POINT('Ctrl Pts',(0.210190822884773,-0.0293435190237031,
1.60382510390846));
#33585=CARTESIAN_POINT('Ctrl Pts',(0.138648901988495,0.160676771609172,
1.61493889296526));
#33586=CARTESIAN_POINT('Ctrl Pts',(-0.0597980782594448,0.203632875576831,
1.62605268202207));
#33587=CARTESIAN_POINT('Ctrl Pts',(-0.203514747072184,0.0601917643824736,
1.63716647107887));
#33588=CARTESIAN_POINT('Ctrl Pts',(-0.160945267273914,-0.13832491317789,
1.64828026013567));
#33589=CARTESIAN_POINT('Ctrl Pts',(0.0289262341422404,-0.210266915972054,
1.65939404919248));
#33590=CARTESIAN_POINT('Ctrl Pts',(0.19234614482316,-0.0896808740081667,
1.67050783824928));
#33591=CARTESIAN_POINT('Ctrl Pts',(0.179661583341645,0.112859981157414,
1.68162162730609));
#33592=CARTESIAN_POINT('Ctrl Pts',(0.00262376933475311,0.212352024863603,
1.69273541636289));
#33593=CARTESIAN_POINT('Ctrl Pts',(-0.177006197242412,0.116971330774799,
1.7038492054197));
#33594=CARTESIAN_POINT('Ctrl Pts',(-0.188438751949388,-0.0172339073385976,
1.71125839812423));
#33595=CARTESIAN_POINT('Ctrl Pts',(-0.164517074058987,-0.0719397484879835,
1.7149629944765));
#33596=CARTESIAN_POINT('Ctrl Pts',(-0.146649036946525,0.124726608657099,
0.785037005523502));
#33597=CARTESIAN_POINT('Ctrl Pts',(-0.188123601695047,0.0759623149459762,
0.78874160187577));
#33598=CARTESIAN_POINT('Ctrl Pts',(-0.217886373242709,-0.0653490907656594,
0.796150794580307));
#33599=CARTESIAN_POINT('Ctrl Pts',(-0.0629708293942997,-0.218813637584587,
0.807264583637111));
#33600=CARTESIAN_POINT('Ctrl Pts',(0.149542981076344,-0.171418700808033,
0.818378372693914));
#33601=CARTESIAN_POINT('Ctrl Pts',(0.225195614202741,0.0325890023924215,
0.829492161750719));
#33602=CARTESIAN_POINT('Ctrl Pts',(0.0947155514542305,0.206917019327413,
0.840605950807523));
#33603=CARTESIAN_POINT('Ctrl Pts',(-0.122454283303893,0.191773665487537,
0.851719739864327));
#33604=CARTESIAN_POINT('Ctrl Pts',(-0.227542641392875,0.00113835931130726,
0.862833528921131));
#33605=CARTESIAN_POINT('Ctrl Pts',(-0.124357429349293,-0.190560134610961,
0.873947317977936));
#33606=CARTESIAN_POINT('Ctrl Pts',(0.0926529161707207,-0.20782568535688,
0.885061107034739));
#33607=CARTESIAN_POINT('Ctrl Pts',(0.224857326815389,-0.0348718222704234,
0.896174896091545));
#33608=CARTESIAN_POINT('Ctrl Pts',(0.151247103781158,0.170003640905229,
0.907288685148347));
#33609=CARTESIAN_POINT('Ctrl Pts',(-0.0608012185617612,0.219271263230777,
0.918402474205154));
#33610=CARTESIAN_POINT('Ctrl Pts',(-0.217197543051952,0.0678382370566187,
0.929516263261956));
#33611=CARTESIAN_POINT('Ctrl Pts',(-0.174790468634879,-0.145688327971602,
0.940630052318761));
#33612=CARTESIAN_POINT('Ctrl Pts',(0.0276042911522686,-0.225864489000412,
0.951743841375564));
#33613=CARTESIAN_POINT('Ctrl Pts',(0.20473253689515,-0.0993044393887096,
0.962857630432368));
#33614=CARTESIAN_POINT('Ctrl Pts',(0.194466766292811,0.118150151218368,
0.973971419489174));
#33615=CARTESIAN_POINT('Ctrl Pts',(0.00620336092773602,0.227460536413689,
0.985085208545976));
#33616=CARTESIAN_POINT('Ctrl Pts',(-0.187738052000287,0.128573729811465,
0.996198997602783));
#33617=CARTESIAN_POINT('Ctrl Pts',(-0.209840696339377,-0.0879980785663373,
1.00731278665958));
#33618=CARTESIAN_POINT('Ctrl Pts',(-0.0398737718241875,-0.224024243094024,
1.01842657571639));
#33619=CARTESIAN_POINT('Ctrl Pts',(0.166590068377075,-0.154998479698188,
1.02954036477319));
#33620=CARTESIAN_POINT('Ctrl Pts',(0.22057212966186,0.055899151215077,1.04065415383));
#33621=CARTESIAN_POINT('Ctrl Pts',(0.0726620192461797,0.215631654430176,
1.0517679428868));
#33622=CARTESIAN_POINT('Ctrl Pts',(-0.141756461448261,0.177994059256345,
1.06288173194361));
#33623=CARTESIAN_POINT('Ctrl Pts',(-0.226423645341368,-0.0225635171224834,
1.07399552100041));
#33624=CARTESIAN_POINT('Ctrl Pts',(-0.103842698840025,-0.202468450298578,
1.08510931005722));
#33625=CARTESIAN_POINT('Ctrl Pts',(0.113786647568658,-0.197051714816478,
1.09622309911402));
#33626=CARTESIAN_POINT('Ctrl Pts',(0.227265785027954,-0.0112713100190907,
1.10733688817082));
#33627=CARTESIAN_POINT('Ctrl Pts',(0.132725972082619,0.184825852650891,
1.11845067722763));
#33628=CARTESIAN_POINT('Ctrl Pts',(-0.0832994283252297,0.211749816328691,
1.12956446628443));
#33629=CARTESIAN_POINT('Ctrl Pts',(-0.223079917307022,0.0448567717109849,
1.14067825534124));
#33630=CARTESIAN_POINT('Ctrl Pts',(-0.158672828079473,-0.163094184762292,
1.15179204439804));
#33631=CARTESIAN_POINT('Ctrl Pts',(0.0509693001615336,-0.221763184309772,
1.16290583345485));
#33632=CARTESIAN_POINT('Ctrl Pts',(0.213958649933481,-0.0774498262924409,
1.17401962251165));
#33633=CARTESIAN_POINT('Ctrl Pts',(0.181109220965206,0.137754236070862,
1.18513341156845));
#33634=CARTESIAN_POINT('Ctrl Pts',(-0.0175115318707909,0.226870283919355,
1.19624720062525));
#33635=CARTESIAN_POINT('Ctrl Pts',(-0.20010378099117,0.108329388012377,
1.20736098968206));
#33636=CARTESIAN_POINT('Ctrl Pts',(-0.199538770039111,-0.109366625281109,
1.21847477873886));
#33637=CARTESIAN_POINT('Ctrl Pts',(-0.0163336599466904,-0.226958126152927,
1.22958856779567));
#33638=CARTESIAN_POINT('Ctrl Pts',(0.181821834331238,-0.13681228027675,
1.24070235685247));
#33639=CARTESIAN_POINT('Ctrl Pts',(0.213553741645938,0.0785593972935142,
1.25181614590928));
#33640=CARTESIAN_POINT('Ctrl Pts',(0.0498174873679621,0.222024767596873,
1.26292993496608));
#33641=CARTESIAN_POINT('Ctrl Pts',(-0.159517278066646,0.162268350186683,
1.27404372402289));
#33642=CARTESIAN_POINT('Ctrl Pts',(-0.222844069837872,-0.0460141283976122,
1.28515751307969));
#33643=CARTESIAN_POINT('Ctrl Pts',(-0.0821991572628677,-0.212179353423901,
1.29627130213649));
#33644=CARTESIAN_POINT('Ctrl Pts',(0.13368357615671,-0.184134409983696,
1.3073850911933));
#33645=CARTESIAN_POINT('Ctrl Pts',(0.227204216245135,0.0124508471406916,
1.3184988802501));
#33646=CARTESIAN_POINT('Ctrl Pts',(0.112762260533419,0.197639702675246,
1.32961266930691));
#33647=CARTESIAN_POINT('Ctrl Pts',(-0.104892271055723,0.20192669696399,
1.34072645836371));
#33648=CARTESIAN_POINT('Ctrl Pts',(-0.226537717387964,0.0213878955180253,
1.35184024742052));
#33649=CARTESIAN_POINT('Ctrl Pts',(-0.140830621883197,-0.178727489252595,
1.36295403647732));
#33650=CARTESIAN_POINT('Ctrl Pts',(0.0737803389603765,-0.215251576199333,
1.37406782553412));
#33651=CARTESIAN_POINT('Ctrl Pts',(0.220859318825196,-0.0547534543384197,
1.38518161459093));
#33652=CARTESIAN_POINT('Ctrl Pts',(0.165783259458819,0.155861125237303,
1.39629540364773));
#33653=CARTESIAN_POINT('Ctrl Pts',(-0.0410360974089359,0.223814249274108,
1.40740919270454));
#33654=CARTESIAN_POINT('Ctrl Pts',(-0.210294648920666,0.0869076527697323,
1.41852298176134));
#33655=CARTESIAN_POINT('Ctrl Pts',(-0.187068123403623,-0.129546504001961,
1.42963677081815));
#33656=CARTESIAN_POINT('Ctrl Pts',(0.0073839770225235,-0.227425276336115,
1.44075055987495));
#33657=CARTESIAN_POINT('Ctrl Pts',(0.195077439423252,-0.117139114382011,
1.45186434893176));
#33658=CARTESIAN_POINT('Ctrl Pts',(0.204214309414691,0.10036580802698,1.46297813798855));
#33659=CARTESIAN_POINT('Ctrl Pts',(0.0264315056232782,0.226004766949337,
1.47409192704536));
#33660=CARTESIAN_POINT('Ctrl Pts',(-0.175544354199732,0.144779001862013,
1.48520571610217));
#33661=CARTESIAN_POINT('Ctrl Pts',(-0.216842477383471,-0.0689646298380053,
1.49631950515897));
#33662=CARTESIAN_POINT('Ctrl Pts',(-0.0596622188548986,-0.21958414549715,
1.50743329421577));
#33663=CARTESIAN_POINT('Ctrl Pts',(0.152127539459117,-0.169215818301425,
1.51854708327258));
#33664=CARTESIAN_POINT('Ctrl Pts',(0.224673246667516,0.0360376966204509,
1.52966087232938));
#33665=CARTESIAN_POINT('Ctrl Pts',(0.0915729621635637,0.208305441316416,
1.54077466138618));
#33666=CARTESIAN_POINT('Ctrl Pts',(-0.125345052777559,0.189908963919433,
1.55188845044299));
#33667=CARTESIAN_POINT('Ctrl Pts',(-0.227533396633615,-0.00231355378679829,
1.56300223949979));
#33668=CARTESIAN_POINT('Ctrl Pts',(-0.121457694281633,-0.192418043741239,
1.5741160285566));
#33669=CARTESIAN_POINT('Ctrl Pts',(0.09578932997347,-0.206400892891616,
1.5852298176134));
#33670=CARTESIAN_POINT('Ctrl Pts',(0.225359836185271,-0.0314611767988859,
1.59634360667021));
#33671=CARTESIAN_POINT('Ctrl Pts',(0.148654890877534,0.172272463810048,
1.60745739572701));
#33672=CARTESIAN_POINT('Ctrl Pts',(-0.0641135751589405,0.218328616121778,
1.61857118478381));
#33673=CARTESIAN_POINT('Ctrl Pts',(-0.218201962540567,0.0645356727509123,
1.62968497384062));
#33674=CARTESIAN_POINT('Ctrl Pts',(-0.172560336221374,-0.148307520501026,
1.64079876289742));
#33675=CARTESIAN_POINT('Ctrl Pts',(0.0310137773775485,-0.225441420744716,
1.65191255195423));
#33676=CARTESIAN_POINT('Ctrl Pts',(0.206227346623875,-0.0961529471080275,
1.66302634101103));
#33677=CARTESIAN_POINT('Ctrl Pts',(0.192627368002909,0.121004839870914,
1.67414013006784));
#33678=CARTESIAN_POINT('Ctrl Pts',(0.00281312104568935,0.227677007397733,
1.68525391912464));
#33679=CARTESIAN_POINT('Ctrl Pts',(-0.189780348479797,0.125412896624096,
1.69636770818145));
#33680=CARTESIAN_POINT('Ctrl Pts',(-0.202037965727701,-0.0184776408472769,
1.70377690088598));
#33681=CARTESIAN_POINT('Ctrl Pts',(-0.17638991251268,-0.0771314832491481,
1.70748149723825));
#33682=CARTESIAN_POINT('Ctrl Pts',(-0.156520011427169,0.133121980333222,
0.777555508285253));
#33683=CARTESIAN_POINT('Ctrl Pts',(-0.200786236992242,0.081075352766987,
0.781260104637521));
#33684=CARTESIAN_POINT('Ctrl Pts',(-0.232552346335619,-0.0697477504548899,
0.788669297342057));
#33685=CARTESIAN_POINT('Ctrl Pts',(-0.06720940785972,-0.233542025016153,
0.799783086398862));
#33686=CARTESIAN_POINT('Ctrl Pts',(0.159608747485041,-0.182956926059375,
0.810896875455666));
#33687=CARTESIAN_POINT('Ctrl Pts',(0.240353573690459,0.0347825743221341,
0.82201066451247));
#33688=CARTESIAN_POINT('Ctrl Pts',(0.101090873180113,0.220844643128561,
0.833124453569275));
#33689=CARTESIAN_POINT('Ctrl Pts',(-0.130696704329673,0.204681987270635,
0.844238242626078));
#33690=CARTESIAN_POINT('Ctrl Pts',(-0.242858579725743,0.00121498249237738,
0.855352031682883));
#33691=CARTESIAN_POINT('Ctrl Pts',(-0.132727951496213,-0.203386773400678,
0.866465820739686));
#33692=CARTESIAN_POINT('Ctrl Pts',(0.0988894015246068,-0.221814471640749,
0.877579609796491));
#33693=CARTESIAN_POINT('Ctrl Pts',(0.239992516114928,-0.0372190512389329,
0.888693398853296));
#33694=CARTESIAN_POINT('Ctrl Pts',(0.161427575012208,0.181446618206226,
0.899807187910099));
#33695=CARTESIAN_POINT('Ctrl Pts',(-0.0648937601106981,0.234030453531351,
0.910920976966904));
#33696=CARTESIAN_POINT('Ctrl Pts',(-0.231817150854124,0.0724044416546206,
0.922034766023707));
#33697=CARTESIAN_POINT('Ctrl Pts',(-0.186555648217912,-0.155494636948999,
0.933148555080512));
#33698=CARTESIAN_POINT('Ctrl Pts',(0.029462341223335,-0.241067470577576,
0.944262344137316));
#33699=CARTESIAN_POINT('Ctrl Pts',(0.218513122769618,-0.105988640031487,
0.95537613319412));
#33700=CARTESIAN_POINT('Ctrl Pts',(0.207556361201707,0.126102860297433,
0.966489922250924));
#33701=CARTESIAN_POINT('Ctrl Pts',(0.00662091032790181,0.242770948244842,
0.977603711307729));
#33702=CARTESIAN_POINT('Ctrl Pts',(-0.200374735874429,0.13722805194188,
0.988717500364533));
#33703=CARTESIAN_POINT('Ctrl Pts',(-0.223965113394512,-0.0939212459185429,
0.999831289421336));
#33704=CARTESIAN_POINT('Ctrl Pts',(-0.0425576829655005,-0.239103357370329,
1.01094507847814));
#33705=CARTESIAN_POINT('Ctrl Pts',(0.177803277464009,-0.16543145675345,
1.02205886753495));
#33706=CARTESIAN_POINT('Ctrl Pts',(0.235418881528546,0.0596617336815061,
1.03317265659175));
#33707=CARTESIAN_POINT('Ctrl Pts',(0.0775529135379212,0.230145861972334,
1.04428644564855));
#33708=CARTESIAN_POINT('Ctrl Pts',(-0.151298115744515,0.18997487313149,
1.05540023470536));
#33709=CARTESIAN_POINT('Ctrl Pts',(-0.241664263837854,-0.0240822717379046,
1.06651402376216));
#33710=CARTESIAN_POINT('Ctrl Pts',(-0.110832370586897,-0.216096640074974,
1.07762781281897));
#33711=CARTESIAN_POINT('Ctrl Pts',(0.121445648389767,-0.210315303100593,
1.08874160187577));
#33712=CARTESIAN_POINT('Ctrl Pts',(0.242563088106409,-0.0120299840334481,
1.09985539093258));
#33713=CARTESIAN_POINT('Ctrl Pts',(0.141659782427545,0.197266515834691,
1.11096917998938));
#33714=CARTESIAN_POINT('Ctrl Pts',(-0.0889063286388705,0.226002736612265,
1.12208296904618));
#33715=CARTESIAN_POINT('Ctrl Pts',(-0.238095468835566,0.0478760895194249,
1.13319675810299));
#33716=CARTESIAN_POINT('Ctrl Pts',(-0.169353126220915,-0.174072085260317,
1.14431054715979));
#33717=CARTESIAN_POINT('Ctrl Pts',(0.0544000534188783,-0.236690106290626,
1.1554243362166));
#33718=CARTESIAN_POINT('Ctrl Pts',(0.228360247225775,-0.0826629887842052,
1.1665381252734));
#33719=CARTESIAN_POINT('Ctrl Pts',(0.193299716965591,0.147026499818165,
1.1776519143302));
#33720=CARTESIAN_POINT('Ctrl Pts',(-0.0186902364010947,0.242140965743205,
1.18876570338701));
#33721=CARTESIAN_POINT('Ctrl Pts',(-0.213572804428157,0.115621059658089,
1.19987949244381));
#33722=CARTESIAN_POINT('Ctrl Pts',(-0.212969762481792,-0.116728113564033,
1.21099328150062));
#33723=CARTESIAN_POINT('Ctrl Pts',(-0.0174330816944656,-0.242234720654174,
1.22210707055742));
#33724=CARTESIAN_POINT('Ctrl Pts',(0.194060296472398,-0.146021140800962,
1.23322085961423));
#33725=CARTESIAN_POINT('Ctrl Pts',(0.227928084484629,0.0838472452197288,
1.24433464867103));
#33726=CARTESIAN_POINT('Ctrl Pts',(0.053170711887795,0.236969296798376,
1.25544843772783));
#33727=CARTESIAN_POINT('Ctrl Pts',(-0.170254416296827,0.17319066360285,
1.26656222678464));
#33728=CARTESIAN_POINT('Ctrl Pts',(-0.237843746428552,-0.0491113481040567,
1.27767601584144));
#33729=CARTESIAN_POINT('Ctrl Pts',(-0.0877319981226961,-0.226461185930791,
1.28878980489824));
#33730=CARTESIAN_POINT('Ctrl Pts',(0.142681843013418,-0.196528532030473,
1.29990359395505));
#33731=CARTESIAN_POINT('Ctrl Pts',(0.242497375117146,0.0132889160223372,
1.31101738301185));
#33732=CARTESIAN_POINT('Ctrl Pts',(0.120352309668968,0.210942868533614,
1.32213117206866));
#33733=CARTESIAN_POINT('Ctrl Pts',(-0.111952589707427,0.215518421220722,
1.33324496112546));
#33734=CARTESIAN_POINT('Ctrl Pts',(-0.241786014095534,0.0228275188203595,
1.34435875018226));
#33735=CARTESIAN_POINT('Ctrl Pts',(-0.150309957742793,-0.190757670439842,
1.35547253923907));
#33736=CARTESIAN_POINT('Ctrl Pts',(0.0787465075641072,-0.229740200603712,
1.36658632829588));
#33737=CARTESIAN_POINT('Ctrl Pts',(0.235725401448916,-0.0584389197308638,
1.37770011735268));
#33738=CARTESIAN_POINT('Ctrl Pts',(0.176942162084499,0.166352167127356,
1.38881390640948));
#33739=CARTESIAN_POINT('Ctrl Pts',(-0.0437982449057285,0.238879228826581,
1.39992769546629));
#33740=CARTESIAN_POINT('Ctrl Pts',(-0.224449621610114,0.0927574233548304,
1.41104148452309));
#33741=CARTESIAN_POINT('Ctrl Pts',(-0.199659714256911,-0.13826630374757,
1.42215527357989));
#33742=CARTESIAN_POINT('Ctrl Pts',(0.00788099391586731,-0.242733314804761,
1.4332690626367));
#33743=CARTESIAN_POINT('Ctrl Pts',(0.208208138856338,-0.125023770379934,
1.4443828516935));
#33744=CARTESIAN_POINT('Ctrl Pts',(0.217960013299196,0.107121449594028,
1.45549664075031));
#33745=CARTESIAN_POINT('Ctrl Pts',(0.028210615278035,0.241217190661839,
1.46661042980711));
#33746=CARTESIAN_POINT('Ctrl Pts',(-0.187360277963068,0.154524103926572,
1.47772421886392));
#33747=CARTESIAN_POINT('Ctrl Pts',(-0.23143818564818,-0.0736066521476796,
1.48883800792072));
#33748=CARTESIAN_POINT('Ctrl Pts',(-0.0636780941176189,-0.234364395962394,
1.49995179697753));
#33749=CARTESIAN_POINT('Ctrl Pts',(0.162367272982574,-0.180605767113594,
1.51106558603433));
#33750=CARTESIAN_POINT('Ctrl Pts',(0.2397960454974,0.0384634008125035,1.52217937509113));
#33751=CARTESIAN_POINT('Ctrl Pts',(0.0977367556084749,0.222326520064881,
1.53329316414794));
#33752=CARTESIAN_POINT('Ctrl Pts',(-0.133782052044684,0.202691772286445,
1.54440695320474));
#33753=CARTESIAN_POINT('Ctrl Pts',(-0.242848712699985,-0.00246927953082339,
1.55552074226155));
#33754=CARTESIAN_POINT('Ctrl Pts',(-0.129633034711377,-0.205369738746763,
1.56663453131835));
#33755=CARTESIAN_POINT('Ctrl Pts',(0.102236927935064,-0.220293776124516,
1.57774832037515));
#33756=CARTESIAN_POINT('Ctrl Pts',(0.240528849485768,-0.0335788345740686,
1.58886210943196));
#33757=CARTESIAN_POINT('Ctrl Pts',(0.158660879766572,0.183868156010923,
1.59997589848876));
#33758=CARTESIAN_POINT('Ctrl Pts',(-0.0684290720584363,0.233024356666725,
1.61108968754557));
#33759=CARTESIAN_POINT('Ctrl Pts',(-0.23288917800895,0.0688795811193509,
1.62220347660237));
#33760=CARTESIAN_POINT('Ctrl Pts',(-0.184175405168835,-0.158290127824162,
1.63331726565918));
#33761=CARTESIAN_POINT('Ctrl Pts',(0.0331013206128567,-0.240615925517378,
1.64443105471598));
#33762=CARTESIAN_POINT('Ctrl Pts',(0.220108548424591,-0.102625020207888,
1.65554484377279));
#33763=CARTESIAN_POINT('Ctrl Pts',(0.205593152664173,0.129149698584414,
1.66665863282959));
#33764=CARTESIAN_POINT('Ctrl Pts',(0.00300247275662535,0.243001989931863,
1.67777242188639));
#33765=CARTESIAN_POINT('Ctrl Pts',(-0.202554499717183,0.133854462473394,
1.6888862109432));
#33766=CARTESIAN_POINT('Ctrl Pts',(-0.215637179506013,-0.0197213743559566,
1.69629540364773));
#33767=CARTESIAN_POINT('Ctrl Pts',(-0.188262750966373,-0.0823232180103128,
1.7));
#33768=CARTESIAN_POINT('Ctrl Pts',(-0.126907087985236,0.107935865304854,
0.8));
#33769=CARTESIAN_POINT('Ctrl Pts',(-0.135120815820747,0.100273328983374,
0.8));
#33770=CARTESIAN_POINT('Ctrl Pts',(-0.142440162795362,0.0917707005673423,
0.8));
#33771=CARTESIAN_POINT('Ctrl Pts',(-0.148860420961125,0.0826220371750322,
0.8));
#33772=CARTESIAN_POINT('Ctrl Pts',(-0.153630780718642,0.0758244264629785,
0.8));
#33773=CARTESIAN_POINT('Ctrl Pts',(-0.157904437427575,0.0686688635836137,
0.8));
#33774=CARTESIAN_POINT('Ctrl Pts',(-0.161669292800466,0.0612205436816197,
0.8));
#33775=CARTESIAN_POINT('Ctrl Pts',(-0.163886790527543,0.0568334873893247,
0.8));
#33776=CARTESIAN_POINT('Ctrl Pts',(-0.165929164676721,0.0523396591094527,
0.8));
#33777=CARTESIAN_POINT('Ctrl Pts',(-0.167781485419322,0.0477808011974605,
0.8));
#33778=CARTESIAN_POINT('Ctrl Pts',(-0.172341905336402,0.0365568776388491,
0.8));
#33779=CARTESIAN_POINT('Ctrl Pts',(-0.175769282371032,0.024914892102173,
0.8));
#33780=CARTESIAN_POINT('Ctrl Pts',(-0.178035222124413,0.0130530737274266,
0.8));
#33781=CARTESIAN_POINT('Ctrl Pts',(-0.179475251863618,0.00551475714368376,
0.8));
#33782=CARTESIAN_POINT('Ctrl Pts',(-0.180445476974817,-0.00211322491662525,
0.8));
#33783=CARTESIAN_POINT('Ctrl Pts',(-0.180929041702956,-0.00978511330991493,
0.8));
#33784=CARTESIAN_POINT('Ctrl Pts',(-0.181154762272538,-0.0133662326867636,
0.8));
#33785=CARTESIAN_POINT('Ctrl Pts',(-0.181273901675413,-0.0169534510679824,
0.8));
#33786=CARTESIAN_POINT('Ctrl Pts',(-0.181285306139082,-0.0205319858475477,
0.8));
#33787=CARTESIAN_POINT('Ctrl Pts',(-0.18132084415518,-0.0316832359459324,
0.8));
#33788=CARTESIAN_POINT('Ctrl Pts',(-0.180314596981932,-0.0427772557222799,
0.8));
#33789=CARTESIAN_POINT('Ctrl Pts',(-0.178232649680767,-0.053673233795859,
0.8));
#33790=CARTESIAN_POINT('Ctrl Pts',(-0.177072367625385,-0.0597456294936455,
0.8));
#33791=CARTESIAN_POINT('Ctrl Pts',(-0.175577442236952,-0.0657567536750286,
0.8));
#33792=CARTESIAN_POINT('Ctrl Pts',(-0.173766632602371,-0.0716904360104152,
0.8));
#33793=CARTESIAN_POINT('Ctrl Pts',(-0.17263375533703,-0.0754026615746807,
0.8));
#33794=CARTESIAN_POINT('Ctrl Pts',(-0.171376588698951,-0.0790860937830887,
0.8));
#33795=CARTESIAN_POINT('Ctrl Pts',(-0.17000084111904,-0.0827319119339195,
0.8));
#33796=CARTESIAN_POINT('Ctrl Pts',(-0.165618690539351,-0.0943448882941177,
0.8));
#33797=CARTESIAN_POINT('Ctrl Pts',(-0.160069009775015,-0.105495622492882,
0.8));
#33798=CARTESIAN_POINT('Ctrl Pts',(-0.153517412526831,-0.116061366452211,
0.8));
#33799=CARTESIAN_POINT('Ctrl Pts',(-0.149177021710609,-0.123061103510275,
0.8));
#33800=CARTESIAN_POINT('Ctrl Pts',(-0.144395700078728,-0.129804236115551,
0.8));
#33801=CARTESIAN_POINT('Ctrl Pts',(-0.139210064136084,-0.136252864813496,
0.8));
#33802=CARTESIAN_POINT('Ctrl Pts',(-0.13649895134849,-0.139624285391187,
0.8));
#33803=CARTESIAN_POINT('Ctrl Pts',(-0.133675938748059,-0.142916515743411,
0.8));
#33804=CARTESIAN_POINT('Ctrl Pts',(-0.130749381376745,-0.146119375612755,
0.8));
#33805=CARTESIAN_POINT('Ctrl Pts',(-0.124483125872831,-0.152977241609597,
0.8));
#33806=CARTESIAN_POINT('Ctrl Pts',(-0.117767487241387,-0.159399582279811,
0.8));
#33807=CARTESIAN_POINT('Ctrl Pts',(-0.110656616745505,-0.165335584860524,
0.8));
#33808=CARTESIAN_POINT('Ctrl Pts',(-0.106173937599239,-0.169077629522446,
0.8));
#33809=CARTESIAN_POINT('Ctrl Pts',(-0.10153394483554,-0.172626328540978,
0.8));
#33810=CARTESIAN_POINT('Ctrl Pts',(-0.0967480797506452,-0.175967583788754,
0.8));
#33811=CARTESIAN_POINT('Ctrl Pts',(-0.0926327467056763,-0.178840706597052,
0.8));
#33812=CARTESIAN_POINT('Ctrl Pts',(-0.0884162860091264,-0.181555556620875,
0.8));
#33813=CARTESIAN_POINT('Ctrl Pts',(-0.0841104480426287,-0.184101786598396,
0.8));
#33814=CARTESIAN_POINT('Ctrl Pts',(-0.0753786167196158,-0.189265299681399,
0.8));
#33815=CARTESIAN_POINT('Ctrl Pts',(-0.0662752406232737,-0.193739549767325,
0.8));
#33816=CARTESIAN_POINT('Ctrl Pts',(-0.0568593821206139,-0.197450435399565,
0.8));
#33817=CARTESIAN_POINT('Ctrl Pts',(-0.0556199805901397,-0.197938896152316,
0.8));
#33818=CARTESIAN_POINT('Ctrl Pts',(-0.0543751496950137,-0.198414110578975,
0.8));
#33819=CARTESIAN_POINT('Ctrl Pts',(-0.0531250805644623,-0.198876136975596,
0.8));
#33820=CARTESIAN_POINT('Ctrl Pts',(0.166729862742343,-0.000130123946020723,
0.912851963660979));
#33821=CARTESIAN_POINT('Ctrl Pts',(0.166803013417109,-0.0086545516860567,
0.912280605963333));
#33822=CARTESIAN_POINT('Ctrl Pts',(0.166205714872852,-0.0171686904331816,
0.911709248265688));
#33823=CARTESIAN_POINT('Ctrl Pts',(0.164902316607877,-0.0255733139699205,
0.911137890568042));
#33824=CARTESIAN_POINT('Ctrl Pts',(0.156451280631859,-0.08006761381865,
0.907433294215774));
#33825=CARTESIAN_POINT('Ctrl Pts',(0.118315613047404,-0.129957863303896,
0.903728697863506));
#33826=CARTESIAN_POINT('Ctrl Pts',(0.0679483908354429,-0.152412778753583,
0.900024101511237));
#33827=CARTESIAN_POINT('Ctrl Pts',(0.017581168623482,-0.17486769420327,
0.896319505158969));
#33828=CARTESIAN_POINT('Ctrl Pts',(-0.045017608215985,-0.169887275617398,
0.892614908806701));
#33829=CARTESIAN_POINT('Ctrl Pts',(-0.0911993932476663,-0.139748404661014,
0.888910312454434));
#33830=CARTESIAN_POINT('Ctrl Pts',(-0.137381178279348,-0.109609533704629,
0.885205716102165));
#33831=CARTESIAN_POINT('Ctrl Pts',(-0.167145971503243,-0.0543122103777309,
0.881501119749897));
#33832=CARTESIAN_POINT('Ctrl Pts',(-0.16687148086939,0.000831769447747308,
0.877796523397629));
#33833=CARTESIAN_POINT('Ctrl Pts',(-0.166596990235537,0.0559757492732252,
0.874091927045361));
#33834=CARTESIAN_POINT('Ctrl Pts',(-0.136283215743936,0.110966385597283,
0.870387330693093));
#33835=CARTESIAN_POINT('Ctrl Pts',(-0.0898039369556689,0.140645828726608,
0.866682734340825));
#33836=CARTESIAN_POINT('Ctrl Pts',(-0.0433246581674013,0.170325271855933,
0.862978137988557));
#33837=CARTESIAN_POINT('Ctrl Pts',(0.0193201249175325,0.174693521790525,
0.859273541636289));
#33838=CARTESIAN_POINT('Ctrl Pts',(0.0694616476641393,0.151734327892468,
0.855568945284021));
#33839=CARTESIAN_POINT('Ctrl Pts',(0.119603170410746,0.12877513399441,0.851864348931753));
#33840=CARTESIAN_POINT('Ctrl Pts',(0.157241432819026,0.0784884962637034,
0.848159752579484));
#33841=CARTESIAN_POINT('Ctrl Pts',(0.16514918952844,0.0239211592586256,
0.844455156227216));
#33842=CARTESIAN_POINT('Ctrl Pts',(0.166289903708577,0.0160496809897125,
0.843920758705137));
#33843=CARTESIAN_POINT('Ctrl Pts',(0.16681196167645,0.00808912649634021,
0.843386361183058));
#33844=CARTESIAN_POINT('Ctrl Pts',(0.166745353727506,0.000120148921586877,
0.842851963660979));
#33845=CARTESIAN_POINT('Ctrl Pts',(0.0530170217188587,-0.198517432567173,
0.8));
#33846=CARTESIAN_POINT('Ctrl Pts',(0.119028790974553,-0.18088801151799,
0.803704596352268));
#33847=CARTESIAN_POINT('Ctrl Pts',(0.230942256426658,-0.0749063428374961,
0.811113789056804));
#33848=CARTESIAN_POINT('Ctrl Pts',(0.188114631577322,0.153856547759368,
0.822227578113608));
#33849=CARTESIAN_POINT('Ctrl Pts',(-0.0272119409517698,0.241262826763902,
0.833341367170412));
#33850=CARTESIAN_POINT('Ctrl Pts',(-0.217470922739143,0.108102090643486,
0.844455156227217));
#33851=CARTESIAN_POINT('Ctrl Pts',(-0.208759451561279,-0.124141896006793,
0.85556894528402));
#33852=CARTESIAN_POINT('Ctrl Pts',(-0.00892472216375234,-0.242686445659381,
0.866682734340826));
#33853=CARTESIAN_POINT('Ctrl Pts',(0.199056267666047,-0.139134372529335,
0.877796523397629));
#33854=CARTESIAN_POINT('Ctrl Pts',(0.224850619698646,0.091788306500609,
0.888910312454433));
#33855=CARTESIAN_POINT('Ctrl Pts',(0.0448304764247631,0.238686010114805,
0.900024101511237));
#33856=CARTESIAN_POINT('Ctrl Pts',(-0.176220286722883,0.167116974718297,
0.911137890568042));
#33857=CARTESIAN_POINT('Ctrl Pts',(-0.235976306336092,-0.0574188764093974,
0.922251679624847));
#33858=CARTESIAN_POINT('Ctrl Pts',(-0.0797396575425977,-0.229397140881452,
0.933365468681649));
#33859=CARTESIAN_POINT('Ctrl Pts',(0.14948314505928,-0.19140635164143,0.944479257738454));
#33860=CARTESIAN_POINT('Ctrl Pts',(0.241882569451173,0.0217812340617926,
0.955593046795258));
#33861=CARTESIAN_POINT('Ctrl Pts',(0.112884009708659,0.215032004451281,
0.966706835852063));
#33862=CARTESIAN_POINT('Ctrl Pts',(-0.119438498942156,0.211461649464463,
0.977820624908867));
#33863=CARTESIAN_POINT('Ctrl Pts',(-0.242437629122786,0.0143379927471741,
0.988934413965671));
#33864=CARTESIAN_POINT('Ctrl Pts',(-0.143530830111561,-0.195909362177039,
1.00004820302247));
#33865=CARTESIAN_POINT('Ctrl Pts',(0.086751356142284,-0.226838671363958,
1.01116199207928));
#33866=CARTESIAN_POINT('Ctrl Pts',(0.237629047152892,-0.05013996417456,
1.02227578113608));
#33867=CARTESIAN_POINT('Ctrl Pts',(0.1710021738693,0.172452416697446,1.03338957019289));
#33868=CARTESIAN_POINT('Ctrl Pts',(-0.0521449271278155,0.237197146991165,
1.04450335924969));
#33869=CARTESIAN_POINT('Ctrl Pts',(-0.227563185653378,0.0848326375129703,
1.0556171483065));
#33870=CARTESIAN_POINT('Ctrl Pts',(-0.194690279246867,-0.145180146557101,
1.0667309373633));
#33871=CARTESIAN_POINT('Ctrl Pts',(0.0163848475034698,-0.242307896337387,
1.0778447264201));
#33872=CARTESIAN_POINT('Ctrl Pts',(0.212462737615647,-0.117648480480376,
1.08895851547691));
#33873=CARTESIAN_POINT('Ctrl Pts',(0.214071074445423,0.114695923700636,
1.10007230453371));
#33874=CARTESIAN_POINT('Ctrl Pts',(0.019737729131079,0.242057848222183,
1.11118609359052));
#33875=CARTESIAN_POINT('Ctrl Pts',(-0.192661783512051,0.147861479120299,
1.12229988264732));
#33876=CARTESIAN_POINT('Ctrl Pts',(-0.228715780766039,-0.0816741786716276,
1.13341367170413));
#33877=CARTESIAN_POINT('Ctrl Pts',(-0.0554236300753314,-0.236452534483491,
1.14452746076093));
#33878=CARTESIAN_POINT('Ctrl Pts',(0.168598397772042,-0.174803203925221,
1.15564124981773));
#33879=CARTESIAN_POINT('Ctrl Pts',(0.238300400101745,0.0468454815872605,
1.16675503887454));
#33880=CARTESIAN_POINT('Ctrl Pts',(0.0898833437085198,0.225615966539919,
1.17786882793134));
#33881=CARTESIAN_POINT('Ctrl Pts',(-0.140804956527845,0.197877598659039,
1.18898261698814));
#33882=CARTESIAN_POINT('Ctrl Pts',(-0.242612883217311,-0.0109803793588139,
1.20009640604495));
#33883=CARTESIAN_POINT('Ctrl Pts',(-0.12235448648082,-0.2097878916237,1.21121019510175));
#33884=CARTESIAN_POINT('Ctrl Pts',(0.109896359325859,-0.21657416752884,
1.22232398415856));
#33885=CARTESIAN_POINT('Ctrl Pts',(0.241557821132076,-0.0251276517767584,
1.23343777321536));
#33886=CARTESIAN_POINT('Ctrl Pts',(0.152118669804104,0.189318488613562,
1.24455156227217));
#33887=CARTESIAN_POINT('Ctrl Pts',(-0.0765564251386213,0.230479269358191,
1.25566535132897));
#33888=CARTESIAN_POINT('Ctrl Pts',(-0.23515855594305,0.0606797610465845,
1.26677914038578));
#33889=CARTESIAN_POINT('Ctrl Pts',(-0.178517393613401,-0.164660620706261,
1.27789292944258));
#33890=CARTESIAN_POINT('Ctrl Pts',(0.0415227636155418,-0.239285268948212,
1.28900671849938));
#33891=CARTESIAN_POINT('Ctrl Pts',(0.223556664406995,-0.0948893968423596,
1.30012050755619));
#33892=CARTESIAN_POINT('Ctrl Pts',(0.200966614961749,0.136359816312279,
1.31123429661299));
#33893=CARTESIAN_POINT('Ctrl Pts',(-0.00557045627447471,0.242797343170749,
1.3223480856698));
#33894=CARTESIAN_POINT('Ctrl Pts',(-0.207008825709279,0.126999708315969,
1.3334618747266));
#33895=CARTESIAN_POINT('Ctrl Pts',(-0.218969669332857,-0.105042199835232,
1.3445756637834));
#33896=CARTESIAN_POINT('Ctrl Pts',(-0.0305050913306782,-0.240937791217362,
1.35568945284021));
#33897=CARTESIAN_POINT('Ctrl Pts',(0.185881142716884,-0.15630028987845,
1.36680324189701));
#33898=CARTESIAN_POINT('Ctrl Pts',(0.23212825880178,0.0714006393532108,
1.37791703095382));
#33899=CARTESIAN_POINT('Ctrl Pts',(0.0659057470887793,0.233747753644337,
1.38903082001062));
#33900=CARTESIAN_POINT('Ctrl Pts',(-0.160641042350602,0.182142898149225,
1.40014460906743));
#33901=CARTESIAN_POINT('Ctrl Pts',(-0.240151263944613,-0.0361794176709605,
1.41125839812423));
#33902=CARTESIAN_POINT('Ctrl Pts',(-0.0998483101275995,-0.221386302178844,
1.42237218718103));
#33903=CARTESIAN_POINT('Ctrl Pts',(0.131846934264022,-0.203955793640817,
1.43348597623784));
#33904=CARTESIAN_POINT('Ctrl Pts',(0.242861184558351,0.00015776588975909,
1.44459976529464));
#33905=CARTESIAN_POINT('Ctrl Pts',(0.13158183823911,0.204126920402922,1.45571355435144));
#33906=CARTESIAN_POINT('Ctrl Pts',(-0.10013585656473,0.221256389923926,
1.46682734340825));
#33907=CARTESIAN_POINT('Ctrl Pts',(-0.240198066802314,0.0358673761285168,
1.47794113246505));
#33908=CARTESIAN_POINT('Ctrl Pts',(-0.160404261381875,-0.182351453033287,
1.48905492152186));
#33909=CARTESIAN_POINT('Ctrl Pts',(0.0662093815164626,-0.233661930697804,
1.50016871057866));
#33910=CARTESIAN_POINT('Ctrl Pts',(0.232220830617013,-0.0710989904726924,
1.51128249963547));
#33911=CARTESIAN_POINT('Ctrl Pts',(0.185677912288661,0.156541656658069,
1.52239628869227));
#33912=CARTESIAN_POINT('Ctrl Pts',(-0.0308180903310451,0.240897960470908,
1.53351007774908));
#33913=CARTESIAN_POINT('Ctrl Pts',(-0.219105973246366,0.104757609325286,
1.54462386680588));
#33914=CARTESIAN_POINT('Ctrl Pts',(-0.206843620635952,-0.127268531807556,
1.55573765586268));
#33915=CARTESIAN_POINT('Ctrl Pts',(-0.00525505851706014,-0.242804414954791,
1.56685144491949));
#33916=CARTESIAN_POINT('Ctrl Pts',(0.201143714017778,-0.136098524667356,
1.57796523397629));
#33917=CARTESIAN_POINT('Ctrl Pts',(0.223432989115882,0.0951796228419585,
1.5890790230331));
#33918=CARTESIAN_POINT('Ctrl Pts',(0.041212233239435,0.2393392912824,1.6001928120899));
#33919=CARTESIAN_POINT('Ctrl Pts',(-0.178731921787321,0.164428017156146,
1.6113066011467));
#33920=CARTESIAN_POINT('Ctrl Pts',(-0.235078089364662,-0.0609842187918821,
1.62242039020351));
#33921=CARTESIAN_POINT('Ctrl Pts',(-0.0762596568913861,-0.230580482955351,
1.63353417926032));
#33922=CARTESIAN_POINT('Ctrl Pts',(0.15236975797671,-0.18911696954633,1.64464796831712));
#33923=CARTESIAN_POINT('Ctrl Pts',(0.241514918660579,0.0254343397173533,
1.65576175737392));
#33924=CARTESIAN_POINT('Ctrl Pts',(0.109634140470589,0.216730418270261,
1.66687554643072));
#33925=CARTESIAN_POINT('Ctrl Pts',(-0.122663843019391,0.209602590285094,
1.67798933548753));
#33926=CARTESIAN_POINT('Ctrl Pts',(-0.242556018767321,0.0107153659861808,
1.68910312454434));
#33927=CARTESIAN_POINT('Ctrl Pts',(-0.140685982558438,-0.198157528783211,
1.70021691360114));
#33928=CARTESIAN_POINT('Ctrl Pts',(0.0904627772969653,-0.225303732602113,
1.71133070265794));
#33929=CARTESIAN_POINT('Ctrl Pts',(0.188575434363683,-0.106431345694512,
1.71873989536248));
#33930=CARTESIAN_POINT('Ctrl Pts',(0.201667586144654,-0.0393720754290199,
1.72244449171475));
#33931=CARTESIAN_POINT('Ctrl Pts',(0.0496734897087673,-0.185997880000277,
0.792518502761751));
#33932=CARTESIAN_POINT('Ctrl Pts',(0.111522209883364,-0.169480262890401,
0.796223099114019));
#33933=CARTESIAN_POINT('Ctrl Pts',(0.216377824064917,-0.0701823552026538,
0.803632291818555));
#33934=CARTESIAN_POINT('Ctrl Pts',(0.176251134310715,0.144153545294923,
0.814746080875359));
#33935=CARTESIAN_POINT('Ctrl Pts',(-0.025495812948363,0.226047524998972,
0.825859869932164));
#33936=CARTESIAN_POINT('Ctrl Pts',(-0.203756063475674,0.101284604698293,
0.836973658988968));
#33937=CARTESIAN_POINT('Ctrl Pts',(-0.195593983451704,-0.116312855641356,
0.848087448045772));
#33938=CARTESIAN_POINT('Ctrl Pts',(-0.0083618822819891,-0.227381363005354,
0.859201237102576));
#33939=CARTESIAN_POINT('Ctrl Pts',(0.186502733326074,-0.130359827804384,
0.87031502615938));
#33940=CARTESIAN_POINT('Ctrl Pts',(0.210670357962369,0.0859996535173407,
0.881428815216184));
#33941=CARTESIAN_POINT('Ctrl Pts',(0.0420032309836913,0.223633215949719,
0.892542604272988));
#33942=CARTESIAN_POINT('Ctrl Pts',(-0.16510690935118,0.156577700042264,
0.903656393329793));
#33943=CARTESIAN_POINT('Ctrl Pts',(-0.221094400331606,-0.0537977403094414,
0.914770182386598));
#33944=CARTESIAN_POINT('Ctrl Pts',(-0.0747108556819193,-0.214930151626042,
0.925883971443401));
#33945=CARTESIAN_POINT('Ctrl Pts',(0.140055952352658,-0.179335261208594,
0.936997760500206));
#33946=CARTESIAN_POINT('Ctrl Pts',(0.226628183455449,0.0204075949748767,
0.948111549557009));
#33947=CARTESIAN_POINT('Ctrl Pts',(0.105764950816784,0.201470956192298,
0.959225338613814));
#33948=CARTESIAN_POINT('Ctrl Pts',(-0.111906079513391,0.198125766554245,
0.970339127670618));
#33949=CARTESIAN_POINT('Ctrl Pts',(-0.227148238147163,0.0134337635740443,
0.981452916727423));
#33950=CARTESIAN_POINT('Ctrl Pts',(-0.134479021666759,-0.183554288235144,
0.992566705784226));
#33951=CARTESIAN_POINT('Ctrl Pts',(0.0812803597193106,-0.212533032641853,
1.00368049484103));
#33952=CARTESIAN_POINT('Ctrl Pts',(0.222642910626845,-0.0469778745330203,
1.01479428389783));
#33953=CARTESIAN_POINT('Ctrl Pts',(0.160217878116906,0.161576661010844,
1.02590807295464));
#33954=CARTESIAN_POINT('Ctrl Pts',(-0.0488563939857563,0.222238248359082,
1.03702186201144));
#33955=CARTESIAN_POINT('Ctrl Pts',(-0.21321185525264,0.0794826455702088,
1.04813565106825));
#33956=CARTESIAN_POINT('Ctrl Pts',(-0.182412087081199,-0.136024323549586,
1.05924944012505));
#33957=CARTESIAN_POINT('Ctrl Pts',(0.0153515329125665,-0.227026686992996,
1.07036322918186));
#33958=CARTESIAN_POINT('Ctrl Pts',(0.199063720825595,-0.110228949022901,
1.08147701823866));
#33959=CARTESIAN_POINT('Ctrl Pts',(0.200570627482587,0.107462595990271,
1.09259080729546));
#33960=CARTESIAN_POINT('Ctrl Pts',(0.0184929642043311,0.226792408226016,
1.10370459635227));
#33961=CARTESIAN_POINT('Ctrl Pts',(-0.180511518947779,0.138536557190134,
1.11481838540907));
#33962=CARTESIAN_POINT('Ctrl Pts',(-0.214291761660261,-0.0765233757420587,
1.12593217446588));
#33963=CARTESIAN_POINT('Ctrl Pts',(-0.0519283246948251,-0.221540595029306,
1.13704596352268));
#33964=CARTESIAN_POINT('Ctrl Pts',(0.157965696772913,-0.163779195241938,
1.14815975257948));
#33965=CARTESIAN_POINT('Ctrl Pts',(0.22327192453058,0.0438911593311794,
1.15927354163629));
#33966=CARTESIAN_POINT('Ctrl Pts',(0.0842148276900768,0.211387438009701,
1.17038733069309));
#33967=CARTESIAN_POINT('Ctrl Pts',(-0.131925055996524,0.185398397380911,
1.1815011197499));
#33968=CARTESIAN_POINT('Ctrl Pts',(-0.227312439797474,-0.0102878989312292,
1.1926149088067));
#33969=CARTESIAN_POINT('Ctrl Pts',(-0.114638169553469,-0.196557564679025,
1.20372869786351));
#33970=CARTESIAN_POINT('Ctrl Pts',(0.102965717368131,-0.202915862361653,
1.21484248692031));
#33971=CARTESIAN_POINT('Ctrl Pts',(0.226323915472005,-0.0235429700022985,
1.22595627597712));
#33972=CARTESIAN_POINT('Ctrl Pts',(0.142525267056592,0.177379069795616,
1.23707006503392));
#33973=CARTESIAN_POINT('Ctrl Pts',(-0.071728374642188,0.215944035394125,
1.24818385409072));
#33974=CARTESIAN_POINT('Ctrl Pts',(-0.220328221575874,0.0568529764244717,
1.25929764314753));
#33975=CARTESIAN_POINT('Ctrl Pts',(-0.16725914860919,-0.154276256623111,
1.27041143220433));
#33976=CARTESIAN_POINT('Ctrl Pts',(0.0389041199272518,-0.224194682371805,
1.28152522126113));
#33977=CARTESIAN_POINT('Ctrl Pts',(0.209458006291536,-0.088905172804972,
1.29263901031794));
#33978=CARTESIAN_POINT('Ctrl Pts',(0.188292604081856,0.127760249683509,
1.30375279937474));
#33979=CARTESIAN_POINT('Ctrl Pts',(-0.0052191540273722,0.227485266736855,
1.31486658843155));
#33980=CARTESIAN_POINT('Ctrl Pts',(-0.193953761266,0.118990439287648,1.32598037748835));
#33981=CARTESIAN_POINT('Ctrl Pts',(-0.205160291232821,-0.0984176866850601,
1.33709416654516));
#33982=CARTESIAN_POINT('Ctrl Pts',(-0.028581279957875,-0.225742987902158,
1.34820795560196));
#33983=CARTESIAN_POINT('Ctrl Pts',(0.174158500995476,-0.146443172193371,
1.35932174465876));
#33984=CARTESIAN_POINT('Ctrl Pts',(0.217489030897462,0.0668977398036206,
1.37043553371557));
#33985=CARTESIAN_POINT('Ctrl Pts',(0.0617493843227067,0.219006391884312,
1.38154932277237));
#33986=CARTESIAN_POINT('Ctrl Pts',(-0.150510174002661,0.17065600977586,
1.39266311182918));
#33987=CARTESIAN_POINT('Ctrl Pts',(-0.225006063172667,-0.0338977534588365,
1.40377690088598));
#33988=CARTESIAN_POINT('Ctrl Pts',(-0.0935513509578539,-0.207424518511403,
1.41489068994279));
#33989=CARTESIAN_POINT('Ctrl Pts',(0.123531973693776,-0.191093269444383,
1.42600447899959));
#33990=CARTESIAN_POINT('Ctrl Pts',(0.22754508195105,0.000147816343643338,
1.43711826805639));
#33991=CARTESIAN_POINT('Ctrl Pts',(0.123283596017355,0.191253604053547,
1.4482320571132));
#33992=CARTESIAN_POINT('Ctrl Pts',(-0.0938207632055154,0.207302799206008,
1.45934584617));
#33993=CARTESIAN_POINT('Ctrl Pts',(-0.225049914396199,0.033605390895932,
1.4704596352268));
#33994=CARTESIAN_POINT('Ctrl Pts',(-0.150288325686177,-0.170851412092914,
1.48157342428361));
#33995=CARTESIAN_POINT('Ctrl Pts',(0.0620338699676892,-0.218925981383812,
1.49268721334041));
#33996=CARTESIAN_POINT('Ctrl Pts',(0.217575764647534,-0.066615114486764,
1.50380100239722));
#33997=CARTESIAN_POINT('Ctrl Pts',(0.173968087346094,0.146669317115412,
1.51491479145402));
#33998=CARTESIAN_POINT('Ctrl Pts',(-0.0288745395963744,0.225705669091897,
1.52602858051083));
#33999=CARTESIAN_POINT('Ctrl Pts',(-0.205287999105225,0.0981510439482811,
1.53714236956763));
#34000=CARTESIAN_POINT('Ctrl Pts',(-0.1937989748928,-0.119242309357106,
1.54825615862444));
#34001=CARTESIAN_POINT('Ctrl Pts',(-0.00492364691005069,-0.227491892537031,
1.55936994768124));
#34002=CARTESIAN_POINT('Ctrl Pts',(0.188458534340702,-0.127515436462881,
1.57048373673804));
#34003=CARTESIAN_POINT('Ctrl Pts',(0.209342130614232,0.0891770956278107,
1.58159752579485));
#34004=CARTESIAN_POINT('Ctrl Pts',(0.0386131732285934,0.224245297773695,
1.59271131485165));
#34005=CARTESIAN_POINT('Ctrl Pts',(-0.167460147509052,0.154058322275268,
1.60382510390846));
#34006=CARTESIAN_POINT('Ctrl Pts',(-0.220252829642796,-0.057138233464333,
1.61493889296526));
#34007=CARTESIAN_POINT('Ctrl Pts',(-0.0714503221602304,-0.21603886592994,
1.62605268202207));
#34008=CARTESIAN_POINT('Ctrl Pts',(0.14276052028949,-0.177190259579807,
1.63716647107887));
#34009=CARTESIAN_POINT('Ctrl Pts',(0.226283718655826,0.0238303165896214,
1.64828026013567));
#34010=CARTESIAN_POINT('Ctrl Pts',(0.102720035411913,0.203062259110174,
1.65939404919248));
#34011=CARTESIAN_POINT('Ctrl Pts',(-0.114928016442956,0.196383949416646,
1.67050783824928));
#34012=CARTESIAN_POINT('Ctrl Pts',(-0.227259161518541,0.0100395986945998,
1.68162162730609));
#34013=CARTESIAN_POINT('Ctrl Pts',(-0.131813585150871,-0.185660673640335,
1.69273541636289));
#34014=CARTESIAN_POINT('Ctrl Pts',(0.0847577191513361,-0.211094895184898,
1.70384920541969));
#34015=CARTESIAN_POINT('Ctrl Pts',(0.176682876451709,-0.0997192257060721,
1.71125839812423));
#34016=CARTESIAN_POINT('Ctrl Pts',(0.188949368338152,-0.0368890654402894,
1.7149629944765));
#34017=CARTESIAN_POINT('Ctrl Pts',(0.0463299576986758,-0.173478327433381,
0.785037005523502));
#34018=CARTESIAN_POINT('Ctrl Pts',(0.104015628792176,-0.158072514262811,
0.78874160187577));
#34019=CARTESIAN_POINT('Ctrl Pts',(0.201813391703176,-0.0654583675678116,
0.796150794580307));
#34020=CARTESIAN_POINT('Ctrl Pts',(0.164387637044107,0.134450542830478,
0.80726458363711));
#34021=CARTESIAN_POINT('Ctrl Pts',(-0.0237796849449563,0.210832223234042,
0.818378372693916));
#34022=CARTESIAN_POINT('Ctrl Pts',(-0.190041204212204,0.0944671187531002,
0.829492161750717));
#34023=CARTESIAN_POINT('Ctrl Pts',(-0.182428515342129,-0.10848381527592,
0.840605950807524));
#34024=CARTESIAN_POINT('Ctrl Pts',(-0.00779904240022581,-0.212076280351327,
0.851719739864326));
#34025=CARTESIAN_POINT('Ctrl Pts',(0.173949198986102,-0.121585283079433,
0.862833528921132));
#34026=CARTESIAN_POINT('Ctrl Pts',(0.196490096226091,0.0802110005340724,
0.873947317977935));
#34027=CARTESIAN_POINT('Ctrl Pts',(0.0391759855426195,0.208580421784633,
0.885061107034741));
#34028=CARTESIAN_POINT('Ctrl Pts',(-0.153993531979477,0.146038425366231,
0.896174896091543));
#34029=CARTESIAN_POINT('Ctrl Pts',(-0.206212494327119,-0.0501766042094856,
0.907288685148349));
#34030=CARTESIAN_POINT('Ctrl Pts',(-0.0696820538212414,-0.200463162370631,
0.918402474205152));
#34031=CARTESIAN_POINT('Ctrl Pts',(0.130628759646036,-0.167264170775759,
0.929516263261957));
#34032=CARTESIAN_POINT('Ctrl Pts',(0.211373797459724,0.0190339558879606,
0.94063005231876));
#34033=CARTESIAN_POINT('Ctrl Pts',(0.098645891924909,0.187909907933315,
0.951743841375565));
#34034=CARTESIAN_POINT('Ctrl Pts',(-0.104373660084627,0.184789883644027,
0.962857630432369));
#34035=CARTESIAN_POINT('Ctrl Pts',(-0.21185884717154,0.0125295344009149,
0.973971419489173));
#34036=CARTESIAN_POINT('Ctrl Pts',(-0.125427213221957,-0.17119921429325,
0.985085208545978));
#34037=CARTESIAN_POINT('Ctrl Pts',(0.0758093632963375,-0.198227393919747,
0.996198997602781));
#34038=CARTESIAN_POINT('Ctrl Pts',(0.207656774100798,-0.0438157848914807,
1.00731278665959));
#34039=CARTESIAN_POINT('Ctrl Pts',(0.149433582364513,0.150700905324243,
1.01842657571639));
#34040=CARTESIAN_POINT('Ctrl Pts',(-0.0455678608436973,0.207279349727,1.0295403647732));
#34041=CARTESIAN_POINT('Ctrl Pts',(-0.198860524851901,0.0741326536274474,
1.04065415383));
#34042=CARTESIAN_POINT('Ctrl Pts',(-0.170133894915531,-0.126868500542071,
1.0517679428868));
#34043=CARTESIAN_POINT('Ctrl Pts',(0.0143182183216636,-0.211745477648606,
1.06288173194361));
#34044=CARTESIAN_POINT('Ctrl Pts',(0.185664704035542,-0.102809417565425,
1.07399552100041));
#34045=CARTESIAN_POINT('Ctrl Pts',(0.187070180519752,0.100229268279905,
1.08510931005721));
#34046=CARTESIAN_POINT('Ctrl Pts',(0.017248199277583,0.211526968229848,
1.09622309911402));
#34047=CARTESIAN_POINT('Ctrl Pts',(-0.168361254383508,0.12921163525997,
1.10733688817082));
#34048=CARTESIAN_POINT('Ctrl Pts',(-0.199867742554481,-0.07137257281249,
1.11845067722763));
#34049=CARTESIAN_POINT('Ctrl Pts',(-0.0484330193143192,-0.206628655575122,
1.12956446628443));
#34050=CARTESIAN_POINT('Ctrl Pts',(0.147332995773784,-0.152755186558655,
1.14067825534124));
#34051=CARTESIAN_POINT('Ctrl Pts',(0.208243448959415,0.0409368370750985,
1.15179204439804));
#34052=CARTESIAN_POINT('Ctrl Pts',(0.0785463116716341,0.197158909479484,
1.16290583345485));
#34053=CARTESIAN_POINT('Ctrl Pts',(-0.123045155465202,0.172919196102783,
1.17401962251165));
#34054=CARTESIAN_POINT('Ctrl Pts',(-0.212011996377637,-0.00959541850364452,
1.18513341156845));
#34055=CARTESIAN_POINT('Ctrl Pts',(-0.106921852626119,-0.18332723773435,
1.19624720062526));
#34056=CARTESIAN_POINT('Ctrl Pts',(0.0960350754104022,-0.189257557194465,
1.20736098968206));
#34057=CARTESIAN_POINT('Ctrl Pts',(0.211090009811934,-0.0219582882278384,
1.21847477873886));
#34058=CARTESIAN_POINT('Ctrl Pts',(0.132931864309081,0.16543965097767,1.22958856779567));
#34059=CARTESIAN_POINT('Ctrl Pts',(-0.0669003241457547,0.201408801430058,
1.24070235685247));
#34060=CARTESIAN_POINT('Ctrl Pts',(-0.205497887208699,0.0530261918023587,
1.25181614590928));
#34061=CARTESIAN_POINT('Ctrl Pts',(-0.156000903604979,-0.143891892539961,
1.26292993496608));
#34062=CARTESIAN_POINT('Ctrl Pts',(0.0362854762389619,-0.209104095795397,
1.27404372402289));
#34063=CARTESIAN_POINT('Ctrl Pts',(0.195359348176077,-0.0829209487675844,
1.28515751307969));
#34064=CARTESIAN_POINT('Ctrl Pts',(0.175618593201963,0.119160683054738,
1.2962713021365));
#34065=CARTESIAN_POINT('Ctrl Pts',(-0.00486785178026968,0.212173190302961,
1.3073850911933));
#34066=CARTESIAN_POINT('Ctrl Pts',(-0.180898696822721,0.110981170259326,
1.3184988802501));
#34067=CARTESIAN_POINT('Ctrl Pts',(-0.191350913132785,-0.0917931735348885,
1.32961266930691));
#34068=CARTESIAN_POINT('Ctrl Pts',(-0.026657468585072,-0.210548184586953,
1.34072645836371));
#34069=CARTESIAN_POINT('Ctrl Pts',(0.162435859274068,-0.136586054508292,
1.35184024742051));
#34070=CARTESIAN_POINT('Ctrl Pts',(0.202849802993145,0.0623948402540306,
1.36295403647732));
#34071=CARTESIAN_POINT('Ctrl Pts',(0.057593021556634,0.204265030124287,
1.37406782553412));
#34072=CARTESIAN_POINT('Ctrl Pts',(-0.14037930565472,0.159169121402496,
1.38518161459093));
#34073=CARTESIAN_POINT('Ctrl Pts',(-0.209860862400721,-0.0316160892467124,
1.39629540364773));
#34074=CARTESIAN_POINT('Ctrl Pts',(-0.0872543917881084,-0.193462734843961,
1.40740919270454));
#34075=CARTESIAN_POINT('Ctrl Pts',(0.11521701312353,-0.178230745247949,
1.41852298176134));
#34076=CARTESIAN_POINT('Ctrl Pts',(0.212228979343748,0.000137866797527619,
1.42963677081814));
#34077=CARTESIAN_POINT('Ctrl Pts',(0.1149853537956,0.178380287704172,1.44075055987495));
#34078=CARTESIAN_POINT('Ctrl Pts',(-0.0875056698463009,0.19334920848809,
1.45186434893175));
#34079=CARTESIAN_POINT('Ctrl Pts',(-0.209901761990083,0.0313434056633472,
1.46297813798856));
#34080=CARTESIAN_POINT('Ctrl Pts',(-0.14017238999048,-0.159351371152542,
1.47409192704536));
#34081=CARTESIAN_POINT('Ctrl Pts',(0.0578583584189162,-0.204190032069821,
1.48520571610217));
#34082=CARTESIAN_POINT('Ctrl Pts',(0.202930698678054,-0.0621312385008357,
1.49631950515897));
#34083=CARTESIAN_POINT('Ctrl Pts',(0.162258262403527,0.136796977572755,
1.50743329421577));
#34084=CARTESIAN_POINT('Ctrl Pts',(-0.0269309888617035,0.210513377712887,
1.51854708327258));
#34085=CARTESIAN_POINT('Ctrl Pts',(-0.191470024964085,0.0915444785712757,
1.52966087232938));
#34086=CARTESIAN_POINT('Ctrl Pts',(-0.180754329149647,-0.111216086906656,
1.54077466138619));
#34087=CARTESIAN_POINT('Ctrl Pts',(-0.00459223530304152,-0.212179370119272,
1.55188845044299));
#34088=CARTESIAN_POINT('Ctrl Pts',(0.175773354663627,-0.118932348258406,
1.5630022394998));
#34089=CARTESIAN_POINT('Ctrl Pts',(0.195251272112581,0.0831745684136627,
1.5741160285566));
#34090=CARTESIAN_POINT('Ctrl Pts',(0.0360141132177518,0.20915130426499,
1.5852298176134));
#34091=CARTESIAN_POINT('Ctrl Pts',(-0.156188373230783,0.14368862739439,
1.59634360667021));
#34092=CARTESIAN_POINT('Ctrl Pts',(-0.20542756992093,-0.0532922481367839,
1.60745739572701));
#34093=CARTESIAN_POINT('Ctrl Pts',(-0.0666409874290749,-0.201497248904528,
1.61857118478382));
#34094=CARTESIAN_POINT('Ctrl Pts',(0.13315128260227,-0.165263549613285,
1.62968497384062));
#34095=CARTESIAN_POINT('Ctrl Pts',(0.211052518651072,0.0222262934618894,
1.64079876289742));
#34096=CARTESIAN_POINT('Ctrl Pts',(0.095805930353238,0.189394099950088,
1.65191255195423));
#34097=CARTESIAN_POINT('Ctrl Pts',(-0.107192189866521,0.183165308548198,
1.66302634101103));
#34098=CARTESIAN_POINT('Ctrl Pts',(-0.21196230426976,0.00936383140301889,
1.67414013006784));
#34099=CARTESIAN_POINT('Ctrl Pts',(-0.122941187743304,-0.173163818497459,
1.68525391912464));
#34100=CARTESIAN_POINT('Ctrl Pts',(0.0790526610057068,-0.196886057767682,
1.69636770818145));
#34101=CARTESIAN_POINT('Ctrl Pts',(0.164790318539736,-0.0930071057176319,
1.70377690088598));
#34102=CARTESIAN_POINT('Ctrl Pts',(0.176231150531649,-0.034406055451559,
1.70748149723825));
#34103=CARTESIAN_POINT('Ctrl Pts',(0.0429864256885843,-0.160958774866485,
0.777555508285253));
#34104=CARTESIAN_POINT('Ctrl Pts',(0.0965090477009877,-0.146664765635222,
0.781260104637521));
#34105=CARTESIAN_POINT('Ctrl Pts',(0.187248959341434,-0.0607343799329692,
0.788669297342056));
#34106=CARTESIAN_POINT('Ctrl Pts',(0.1525241397775,0.124747540366033,0.799783086398862));
#34107=CARTESIAN_POINT('Ctrl Pts',(-0.0220635569415495,0.195616921469113,
0.810896875455666));
#34108=CARTESIAN_POINT('Ctrl Pts',(-0.176326344948735,0.0876496328079073,
0.82201066451247));
#34109=CARTESIAN_POINT('Ctrl Pts',(-0.169263047232554,-0.100654774910484,
0.833124453569274));
#34110=CARTESIAN_POINT('Ctrl Pts',(-0.00723620251846265,-0.196771197697301,
0.844238242626078));
#34111=CARTESIAN_POINT('Ctrl Pts',(0.161395664646129,-0.112810738354482,
0.855352031682883));
#34112=CARTESIAN_POINT('Ctrl Pts',(0.182309834489814,0.0744223475508041,
0.866465820739686));
#34113=CARTESIAN_POINT('Ctrl Pts',(0.0363487401015477,0.193527627619547,
0.877579609796491));
#34114=CARTESIAN_POINT('Ctrl Pts',(-0.142880154607774,0.135499150690198,
0.888693398853294));
#34115=CARTESIAN_POINT('Ctrl Pts',(-0.191330588322633,-0.0465554681095297,
0.8998071879101));
#34116=CARTESIAN_POINT('Ctrl Pts',(-0.0646532519605634,-0.185996173115221,
0.910920976966903));
#34117=CARTESIAN_POINT('Ctrl Pts',(0.121201566939414,-0.155193080342923,
0.922034766023707));
#34118=CARTESIAN_POINT('Ctrl Pts',(0.196119411464,0.0176603168010446,0.933148555080512));
#34119=CARTESIAN_POINT('Ctrl Pts',(0.0915268330330338,0.174348859674332,
0.944262344137316));
#34120=CARTESIAN_POINT('Ctrl Pts',(-0.0968412406558618,0.17145400073381,
0.95537613319412));
#34121=CARTESIAN_POINT('Ctrl Pts',(-0.196569456195918,0.0116253052277854,
0.966489922250924));
#34122=CARTESIAN_POINT('Ctrl Pts',(-0.116375404777155,-0.158844140351355,
0.977603711307728));
#34123=CARTESIAN_POINT('Ctrl Pts',(0.0703383668733642,-0.183921755197642,
0.988717500364533));
#34124=CARTESIAN_POINT('Ctrl Pts',(0.19267063757475,-0.0406536952499414,
0.999831289421336));
#34125=CARTESIAN_POINT('Ctrl Pts',(0.13864928661212,0.139825149637642,1.01094507847814));
#34126=CARTESIAN_POINT('Ctrl Pts',(-0.0422793277016381,0.192320451094917,
1.02205886753494));
#34127=CARTESIAN_POINT('Ctrl Pts',(-0.184509194451163,0.0687826616846859,
1.03317265659175));
#34128=CARTESIAN_POINT('Ctrl Pts',(-0.157855702749863,-0.117712677534557,
1.04428644564855));
#34129=CARTESIAN_POINT('Ctrl Pts',(0.0132849037307607,-0.196464268304215,
1.05540023470536));
#34130=CARTESIAN_POINT('Ctrl Pts',(0.172265687245489,-0.0953898861079487,
1.06651402376216));
#34131=CARTESIAN_POINT('Ctrl Pts',(0.173569733556916,0.0929959405695393,
1.07762781281897));
#34132=CARTESIAN_POINT('Ctrl Pts',(0.0160034343508349,0.196261528233681,
1.08874160187577));
#34133=CARTESIAN_POINT('Ctrl Pts',(-0.156210989819237,0.119886713329805,
1.09985539093257));
#34134=CARTESIAN_POINT('Ctrl Pts',(-0.185443723448703,-0.066221769882921,
1.11096917998938));
#34135=CARTESIAN_POINT('Ctrl Pts',(-0.0449377139338128,-0.191716716120937,
1.12208296904618));
#34136=CARTESIAN_POINT('Ctrl Pts',(0.136700294774655,-0.141731177875371,
1.13319675810299));
#34137=CARTESIAN_POINT('Ctrl Pts',(0.193214973388251,0.0379825148190173,
1.14431054715979));
#34138=CARTESIAN_POINT('Ctrl Pts',(0.0728777956531908,0.182930380949266,
1.1554243362166));
#34139=CARTESIAN_POINT('Ctrl Pts',(-0.11416525493388,0.160439994824655,
1.1665381252734));
#34140=CARTESIAN_POINT('Ctrl Pts',(-0.196711552957801,-0.00890293807605981,
1.1776519143302));
#34141=CARTESIAN_POINT('Ctrl Pts',(-0.0992055356987686,-0.170096910789675,
1.18876570338701));
#34142=CARTESIAN_POINT('Ctrl Pts',(0.0891044334526734,-0.175599252027278,
1.19987949244381));
#34143=CARTESIAN_POINT('Ctrl Pts',(0.195856104151863,-0.0203736064533785,
1.21099328150062));
#34144=CARTESIAN_POINT('Ctrl Pts',(0.12333846156157,0.153500232159725,1.22210707055742));
#34145=CARTESIAN_POINT('Ctrl Pts',(-0.0620722736493212,0.186873567465992,
1.23322085961422));
#34146=CARTESIAN_POINT('Ctrl Pts',(-0.190667552841524,0.0491994071802457,
1.24433464867103));
#34147=CARTESIAN_POINT('Ctrl Pts',(-0.144742658600767,-0.13350752845681,
1.25544843772783));
#34148=CARTESIAN_POINT('Ctrl Pts',(0.0336668325506717,-0.194013509218991,
1.26656222678464));
#34149=CARTESIAN_POINT('Ctrl Pts',(0.181260690060617,-0.0769367247301966,
1.27767601584144));
#34150=CARTESIAN_POINT('Ctrl Pts',(0.16294458232207,0.110561116425968,1.28878980489824));
#34151=CARTESIAN_POINT('Ctrl Pts',(-0.00451654953316709,0.196861113869068,
1.29990359395505));
#34152=CARTESIAN_POINT('Ctrl Pts',(-0.167843632379442,0.102971901231004,
1.31101738301185));
#34153=CARTESIAN_POINT('Ctrl Pts',(-0.177541535032749,-0.0851686603847167,
1.32213117206866));
#34154=CARTESIAN_POINT('Ctrl Pts',(-0.0247336572122691,-0.195353381271748,
1.33324496112546));
#34155=CARTESIAN_POINT('Ctrl Pts',(0.15071321755266,-0.126728936823214,
1.34435875018226));
#34156=CARTESIAN_POINT('Ctrl Pts',(0.188210575088826,0.0578919407044404,
1.35547253923907));
#34157=CARTESIAN_POINT('Ctrl Pts',(0.0534366587905616,0.189523668364262,
1.36658632829587));
#34158=CARTESIAN_POINT('Ctrl Pts',(-0.130248437306779,0.147682233029131,
1.37770011735268));
#34159=CARTESIAN_POINT('Ctrl Pts',(-0.194715661628775,-0.0293344250345881,
1.38881390640948));
#34160=CARTESIAN_POINT('Ctrl Pts',(-0.0809574326183627,-0.17950095117652,
1.39992769546629));
#34161=CARTESIAN_POINT('Ctrl Pts',(0.106902052553284,-0.165368221051515,
1.41104148452309));
#34162=CARTESIAN_POINT('Ctrl Pts',(0.196912876736446,0.000127917251411783,
1.4221552735799));
#34163=CARTESIAN_POINT('Ctrl Pts',(0.106687111573845,0.165506971354797,
1.4332690626367));
#34164=CARTESIAN_POINT('Ctrl Pts',(-0.0811905764870862,0.179395617770172,
1.44438285169351));
#34165=CARTESIAN_POINT('Ctrl Pts',(-0.194753609583967,0.0290814204307625,
1.45549664075031));
#34166=CARTESIAN_POINT('Ctrl Pts',(-0.130056454294782,-0.14785133021217,
1.46661042980711));
#34167=CARTESIAN_POINT('Ctrl Pts',(0.053682846870143,-0.189454082755829,
1.47772421886392));
#34168=CARTESIAN_POINT('Ctrl Pts',(0.188285632708575,-0.0576473625149073,
1.48883800792072));
#34169=CARTESIAN_POINT('Ctrl Pts',(0.15054843746096,0.126924638030098,1.49995179697752));
#34170=CARTESIAN_POINT('Ctrl Pts',(-0.024987438127033,0.195321086333876,
1.51106558603433));
#34171=CARTESIAN_POINT('Ctrl Pts',(-0.177652050822945,0.0849379131942705,
1.52217937509113));
#34172=CARTESIAN_POINT('Ctrl Pts',(-0.167709683406495,-0.103189864456206,
1.53329316414794));
#34173=CARTESIAN_POINT('Ctrl Pts',(-0.00426082369603206,-0.196866847701512,
1.54440695320474));
#34174=CARTESIAN_POINT('Ctrl Pts',(0.163088174986552,-0.110349260053931,
1.55552074226154));
#34175=CARTESIAN_POINT('Ctrl Pts',(0.181160413610931,0.0771720411995148,
1.56663453131835));
#34176=CARTESIAN_POINT('Ctrl Pts',(0.03341505320691,0.194057310756286,1.57774832037515));
#34177=CARTESIAN_POINT('Ctrl Pts',(-0.144916598952513,0.133318932513512,
1.58886210943196));
#34178=CARTESIAN_POINT('Ctrl Pts',(-0.190602310199064,-0.049446262809235,
1.59997589848876));
#34179=CARTESIAN_POINT('Ctrl Pts',(-0.0618316526979189,-0.186955631879117,
1.61108968754557));
#34180=CARTESIAN_POINT('Ctrl Pts',(0.12354204491505,-0.153336839646763,
1.62220347660237));
#34181=CARTESIAN_POINT('Ctrl Pts',(0.195821318646319,0.0206222703341576,
1.63331726565918));
#34182=CARTESIAN_POINT('Ctrl Pts',(0.0888918252945621,0.175725940790001,
1.64443105471598));
#34183=CARTESIAN_POINT('Ctrl Pts',(-0.0994563632900866,0.16994666767975,
1.65554484377278));
#34184=CARTESIAN_POINT('Ctrl Pts',(-0.19666544702098,0.008688064111438,
1.66665863282959));
#34185=CARTESIAN_POINT('Ctrl Pts',(-0.114068790335738,-0.160666963354583,
1.67777242188639));
#34186=CARTESIAN_POINT('Ctrl Pts',(0.0733476028600775,-0.182677220350466,
1.6888862109432));
#34187=CARTESIAN_POINT('Ctrl Pts',(0.152897760627763,-0.0862949857291919,
1.69629540364773));
#34188=CARTESIAN_POINT('Ctrl Pts',(0.163512932725146,-0.0319230454628286,
1.7));
#34189=CARTESIAN_POINT('Ctrl Pts',(0.166381444272219,9.40568719243839E-5,
0.86214803633902));
#34190=CARTESIAN_POINT('Ctrl Pts',(0.166493197029431,0.0216823422355625,
0.863587297805909));
#34191=CARTESIAN_POINT('Ctrl Pts',(0.162594223870085,0.0432319486948127,
0.865026559272798));
#34192=CARTESIAN_POINT('Ctrl Pts',(0.154497290451155,0.0630677132447136,
0.866465820739686));
#34193=CARTESIAN_POINT('Ctrl Pts',(0.133656136360392,0.114124107573719,
0.870170417091954));
#34194=CARTESIAN_POINT('Ctrl Pts',(0.0850024382309698,0.153825867596633,
0.873875013444223));
#34195=CARTESIAN_POINT('Ctrl Pts',(0.0308041067147051,0.164005334786532,
0.877579609796491));
#34196=CARTESIAN_POINT('Ctrl Pts',(-0.0233942248015594,0.174184801976431,
0.881284206148759));
#34197=CARTESIAN_POINT('Ctrl Pts',(-0.0831371897046666,0.154841976333314,
0.884988802501027));
#34198=CARTESIAN_POINT('Ctrl Pts',(-0.12108374444203,0.114828127045135,
0.888693398853295));
#34199=CARTESIAN_POINT('Ctrl Pts',(-0.159030299179393,0.0748142777569551,
0.892397995205563));
#34200=CARTESIAN_POINT('Ctrl Pts',(-0.175180443751013,0.0141294048237127,
0.896102591557831));
#34201=CARTESIAN_POINT('Ctrl Pts',(-0.162142626643145,-0.039453149143857,
0.899807187910099));
#34202=CARTESIAN_POINT('Ctrl Pts',(-0.149104809535276,-0.0930357031114267,
0.903511784262367));
#34203=CARTESIAN_POINT('Ctrl Pts',(-0.10687903074792,-0.139515938113324,
0.907216380614635));
#34204=CARTESIAN_POINT('Ctrl Pts',(-0.0547903382042454,-0.157622206818889,
0.910920976966903));
#34205=CARTESIAN_POINT('Ctrl Pts',(-0.00270164566057092,-0.175728475524455,
0.914625573319171));
#34206=CARTESIAN_POINT('Ctrl Pts',(0.0592499606394216,-0.165460777933689,
0.918330169671439));
#34207=CARTESIAN_POINT('Ctrl Pts',(0.102712071210182,-0.131518029614312,
0.922034766023707));
#34208=CARTESIAN_POINT('Ctrl Pts',(0.142261505739626,-0.100630976850939,
0.925405856128812));
#34209=CARTESIAN_POINT('Ctrl Pts',(0.166500629757864,-0.0501396913203886,
0.928776946233916));
#34210=CARTESIAN_POINT('Ctrl Pts',(0.16681765906064,8.64047405809373E-5,
0.93214803633902));
#34211=CARTESIAN_POINT('Ctrl Pts',(0.0530170217188587,-0.198517432567173,
0.8));
#34212=CARTESIAN_POINT('Ctrl Pts',(0.0654219024915668,-0.193924365121538,
0.8));
#34213=CARTESIAN_POINT('Ctrl Pts',(0.0772726753754473,-0.188065368475528,
0.8));
#34214=CARTESIAN_POINT('Ctrl Pts',(0.0884514733522922,-0.181103303150236,
0.8));
#34215=CARTESIAN_POINT('Ctrl Pts',(0.09412650504638,-0.177568939128346,
0.8));
#34216=CARTESIAN_POINT('Ctrl Pts',(0.0996279181736098,-0.173749544851002,
0.8));
#34217=CARTESIAN_POINT('Ctrl Pts',(0.104936837602987,-0.16966283510169,
0.8));
#34218=CARTESIAN_POINT('Ctrl Pts',(0.10962098777257,-0.166057061380704,
0.8));
#34219=CARTESIAN_POINT('Ctrl Pts',(0.114155265023366,-0.162243133727946,
0.8));
#34220=CARTESIAN_POINT('Ctrl Pts',(0.118524756406352,-0.158232269033094,
0.8));
#34221=CARTESIAN_POINT('Ctrl Pts',(0.121396569737292,-0.155596160230106,
0.8));
#34222=CARTESIAN_POINT('Ctrl Pts',(0.124191187364035,-0.152880333162932,
0.8));
#34223=CARTESIAN_POINT('Ctrl Pts',(0.126901910586196,-0.150092210881471,
0.8));
#34224=CARTESIAN_POINT('Ctrl Pts',(0.135875513595552,-0.140862385316535,
0.8));
#34225=CARTESIAN_POINT('Ctrl Pts',(0.143945927205397,-0.130830324459656,
0.8));
#34226=CARTESIAN_POINT('Ctrl Pts',(0.150974563153614,-0.120127060905897,
0.8));
#34227=CARTESIAN_POINT('Ctrl Pts',(0.155531899783608,-0.113187111901085,
0.8));
#34228=CARTESIAN_POINT('Ctrl Pts',(0.159650421905677,-0.105964391211092,
0.8));
#34229=CARTESIAN_POINT('Ctrl Pts',(0.163280590687062,-0.0984918775736134,
0.8));
#34230=CARTESIAN_POINT('Ctrl Pts',(0.165013714615195,-0.0949243321044268,
0.8));
#34231=CARTESIAN_POINT('Ctrl Pts',(0.166631773157808,-0.0913069558365289,
0.8));
#34232=CARTESIAN_POINT('Ctrl Pts',(0.168128066663937,-0.0876495022602451,
0.8));
#34233=CARTESIAN_POINT('Ctrl Pts',(0.172146949722996,-0.0778259762228617,
0.8));
#34234=CARTESIAN_POINT('Ctrl Pts',(0.175295994023174,-0.0677004884915743,
0.8));
#34235=CARTESIAN_POINT('Ctrl Pts',(0.177480263226672,-0.0573468152173212,
0.8));
#34236=CARTESIAN_POINT('Ctrl Pts',(0.179333801272362,-0.048560843554235,
0.8));
#34237=CARTESIAN_POINT('Ctrl Pts',(0.180491858406323,-0.0396100717078052,
0.8));
#34238=CARTESIAN_POINT('Ctrl Pts',(0.18096708784323,-0.0305729202789466,
0.8));
#34239=CARTESIAN_POINT('Ctrl Pts',(0.181136159028966,-0.0273577955642423,
0.8));
#34240=CARTESIAN_POINT('Ctrl Pts',(0.181218443079545,-0.0241331712280784,
0.8));
#34241=CARTESIAN_POINT('Ctrl Pts',(0.181214870924098,-0.0209122942089756,
0.8));
#34242=CARTESIAN_POINT('Ctrl Pts',(0.1812018830209,-0.00920159472786908,
0.8));
#34243=CARTESIAN_POINT('Ctrl Pts',(0.180059445076844,0.00249593154933228,
0.8));
#34244=CARTESIAN_POINT('Ctrl Pts',(0.177833010924532,0.0140076329059244,
0.8));
#34245=CARTESIAN_POINT('Ctrl Pts',(0.176687470499003,0.019930610352574,
0.8));
#34246=CARTESIAN_POINT('Ctrl Pts',(0.17525426981669,0.0258042115192748,
0.8));
#34247=CARTESIAN_POINT('Ctrl Pts',(0.173535645755736,0.0316026384872638,
0.8));
#34248=CARTESIAN_POINT('Ctrl Pts',(0.171850920647243,0.0372866945438873,
0.8));
#34249=CARTESIAN_POINT('Ctrl Pts',(0.169889181319091,0.0429039115259332,
0.8));
#34250=CARTESIAN_POINT('Ctrl Pts',(0.167664346683561,0.0483972355746533,
0.8));
#34251=CARTESIAN_POINT('Ctrl Pts',(0.16420912784319,0.0569284928853236,
0.8));
#34252=CARTESIAN_POINT('Ctrl Pts',(0.160117674787075,0.065174591642692,
0.8));
#34253=CARTESIAN_POINT('Ctrl Pts',(0.155399354804051,0.073039643321633,
0.8));
#34254=CARTESIAN_POINT('Ctrl Pts',(0.15298274940935,0.0770679259275847,
0.8));
#34255=CARTESIAN_POINT('Ctrl Pts',(0.150400765188628,0.0809963604120499,
0.8));
#34256=CARTESIAN_POINT('Ctrl Pts',(0.147663479517856,0.0847983168718068,
0.8));
#34257=CARTESIAN_POINT('Ctrl Pts',(0.142228073022467,0.0923478317277872,
0.8));
#34258=CARTESIAN_POINT('Ctrl Pts',(0.136173701728632,0.0994134091821942,
0.8));
#34259=CARTESIAN_POINT('Ctrl Pts',(0.129505054411736,0.105883695181419,
0.8));
#34260=CARTESIAN_POINT('Ctrl Pts',(0.128726565799248,0.106639027369579,
0.8));
#34261=CARTESIAN_POINT('Ctrl Pts',(0.127939691591626,0.107386221438147,
0.8));
#34262=CARTESIAN_POINT('Ctrl Pts',(0.127144588893496,0.108125211870903,
0.8));
#34263=CARTESIAN_POINT('Origin',(0.,0.,1.3));
#34264=CARTESIAN_POINT('Origin',(0.,0.,1.8));
#34265=CARTESIAN_POINT('Origin',(0.4,0.6,0.8));
#34266=CARTESIAN_POINT('',(0.4,0.6,0.8));
#34267=CARTESIAN_POINT('',(-0.4,0.6,0.8));
#34268=CARTESIAN_POINT('',(0.4,0.6,0.8));
#34269=CARTESIAN_POINT('',(-0.4,0.6,3.6));
#34270=CARTESIAN_POINT('',(-0.4,0.6,0.8));
#34271=CARTESIAN_POINT('',(0.4,0.6,3.6));
#34272=CARTESIAN_POINT('',(0.4,0.6,3.6));
#34273=CARTESIAN_POINT('',(0.4,0.6,0.8));
#34274=CARTESIAN_POINT('Origin',(0.4,-0.6,0.8));
#34275=CARTESIAN_POINT('',(0.4,-0.6,0.8));
#34276=CARTESIAN_POINT('',(0.4,-0.6,0.8));
#34277=CARTESIAN_POINT('',(0.4,-0.6,3.6));
#34278=CARTESIAN_POINT('',(0.4,-0.6,3.6));
#34279=CARTESIAN_POINT('',(0.4,-0.6,0.8));
#34280=CARTESIAN_POINT('Origin',(-0.4,-0.6,0.8));
#34281=CARTESIAN_POINT('',(-0.4,-0.6,0.8));
#34282=CARTESIAN_POINT('',(-0.4,-0.6,0.8));
#34283=CARTESIAN_POINT('',(-0.4,-0.6,3.6));
#34284=CARTESIAN_POINT('',(-0.4,-0.6,3.6));
#34285=CARTESIAN_POINT('',(-0.4,-0.6,0.8));
#34286=CARTESIAN_POINT('Origin',(-0.4,0.6,0.8));
#34287=CARTESIAN_POINT('',(-0.4,0.6,0.8));
#34288=CARTESIAN_POINT('',(-0.4,0.6,3.6));
#34289=CARTESIAN_POINT('Origin',(0.,0.,3.6));
#34290=CARTESIAN_POINT('Origin',(0.,0.,0.8));
#43951=UNCERTAINTY_MEASURE_WITH_UNIT(LENGTH_MEASURE(0.001),#43981,
'DISTANCE_ACCURACY_VALUE',
'Maximum model space distance between geometric entities at asserted c
onnectivities');
#43961=UNCERTAINTY_MEASURE_WITH_UNIT(LENGTH_MEASURE(0.001),#43981,
'DISTANCE_ACCURACY_VALUE',
'Maximum model space distance between geometric entities at asserted c
onnectivities');
#43970=(
GEOMETRIC_REPRESENTATION_CONTEXT(3)
GLOBAL_UNCERTAINTY_ASSIGNED_CONTEXT((#43951))
GLOBAL_UNIT_ASSIGNED_CONTEXT((#43981,#43983,#43984))
REPRESENTATION_CONTEXT('','3D')
);
#43980=(
GEOMETRIC_REPRESENTATION_CONTEXT(3)
GLOBAL_UNCERTAINTY_ASSIGNED_CONTEXT((#43961))
GLOBAL_UNIT_ASSIGNED_CONTEXT((#43981,#43983,#43984))
REPRESENTATION_CONTEXT('','3D')
);
#43981=(
LENGTH_UNIT()
NAMED_UNIT(*)
SI_UNIT(.CENTI.,.METRE.)
);
#43983=(
NAMED_UNIT(*)
PLANE_ANGLE_UNIT()
SI_UNIT($,.RADIAN.)
);
#43984=(
NAMED_UNIT(*)
SI_UNIT($,.STERADIAN.)
SOLID_ANGLE_UNIT()
);
#43993=SHAPE_DEFINITION_REPRESENTATION(#44011,#44063);
#44011=PRODUCT_DEFINITION_SHAPE('',$,#44082);
#44063=SHAPE_REPRESENTATION('',(#11896),#43970);
#44073=PRODUCT_DEFINITION_CONTEXT('part definition',#44129,'design');
#44082=PRODUCT_DEFINITION('Terminal insulator','Terminal insulator',#44100,
#44073);
#44100=PRODUCT_DEFINITION_FORMATION('',$,#44139);
#44129=APPLICATION_CONTEXT(
'Core Data for Automotive Mechanical Design Process');
#44130=PRODUCT_CONTEXT('part definition',#44129,'mechanical');
#44139=PRODUCT('Terminal insulator','Terminal insulator',$,(#44130));
#44156=PRESENTATION_STYLE_ASSIGNMENT((#44168));
#44168=SURFACE_STYLE_USAGE(.BOTH.,#44180);
#44180=SURFACE_SIDE_STYLE('',(#44192));
#44192=SURFACE_STYLE_FILL_AREA(#44204);
#44204=FILL_AREA_STYLE('Insulator gray',(#44216));
#44216=FILL_AREA_STYLE_COLOUR('Insulator gray',#44228);
#44228=COLOUR_RGB('Insulator gray',0.576470588235294,0.615686274509804,
0.666666666666667);
ENDSEC;
END-ISO-10303-21;
